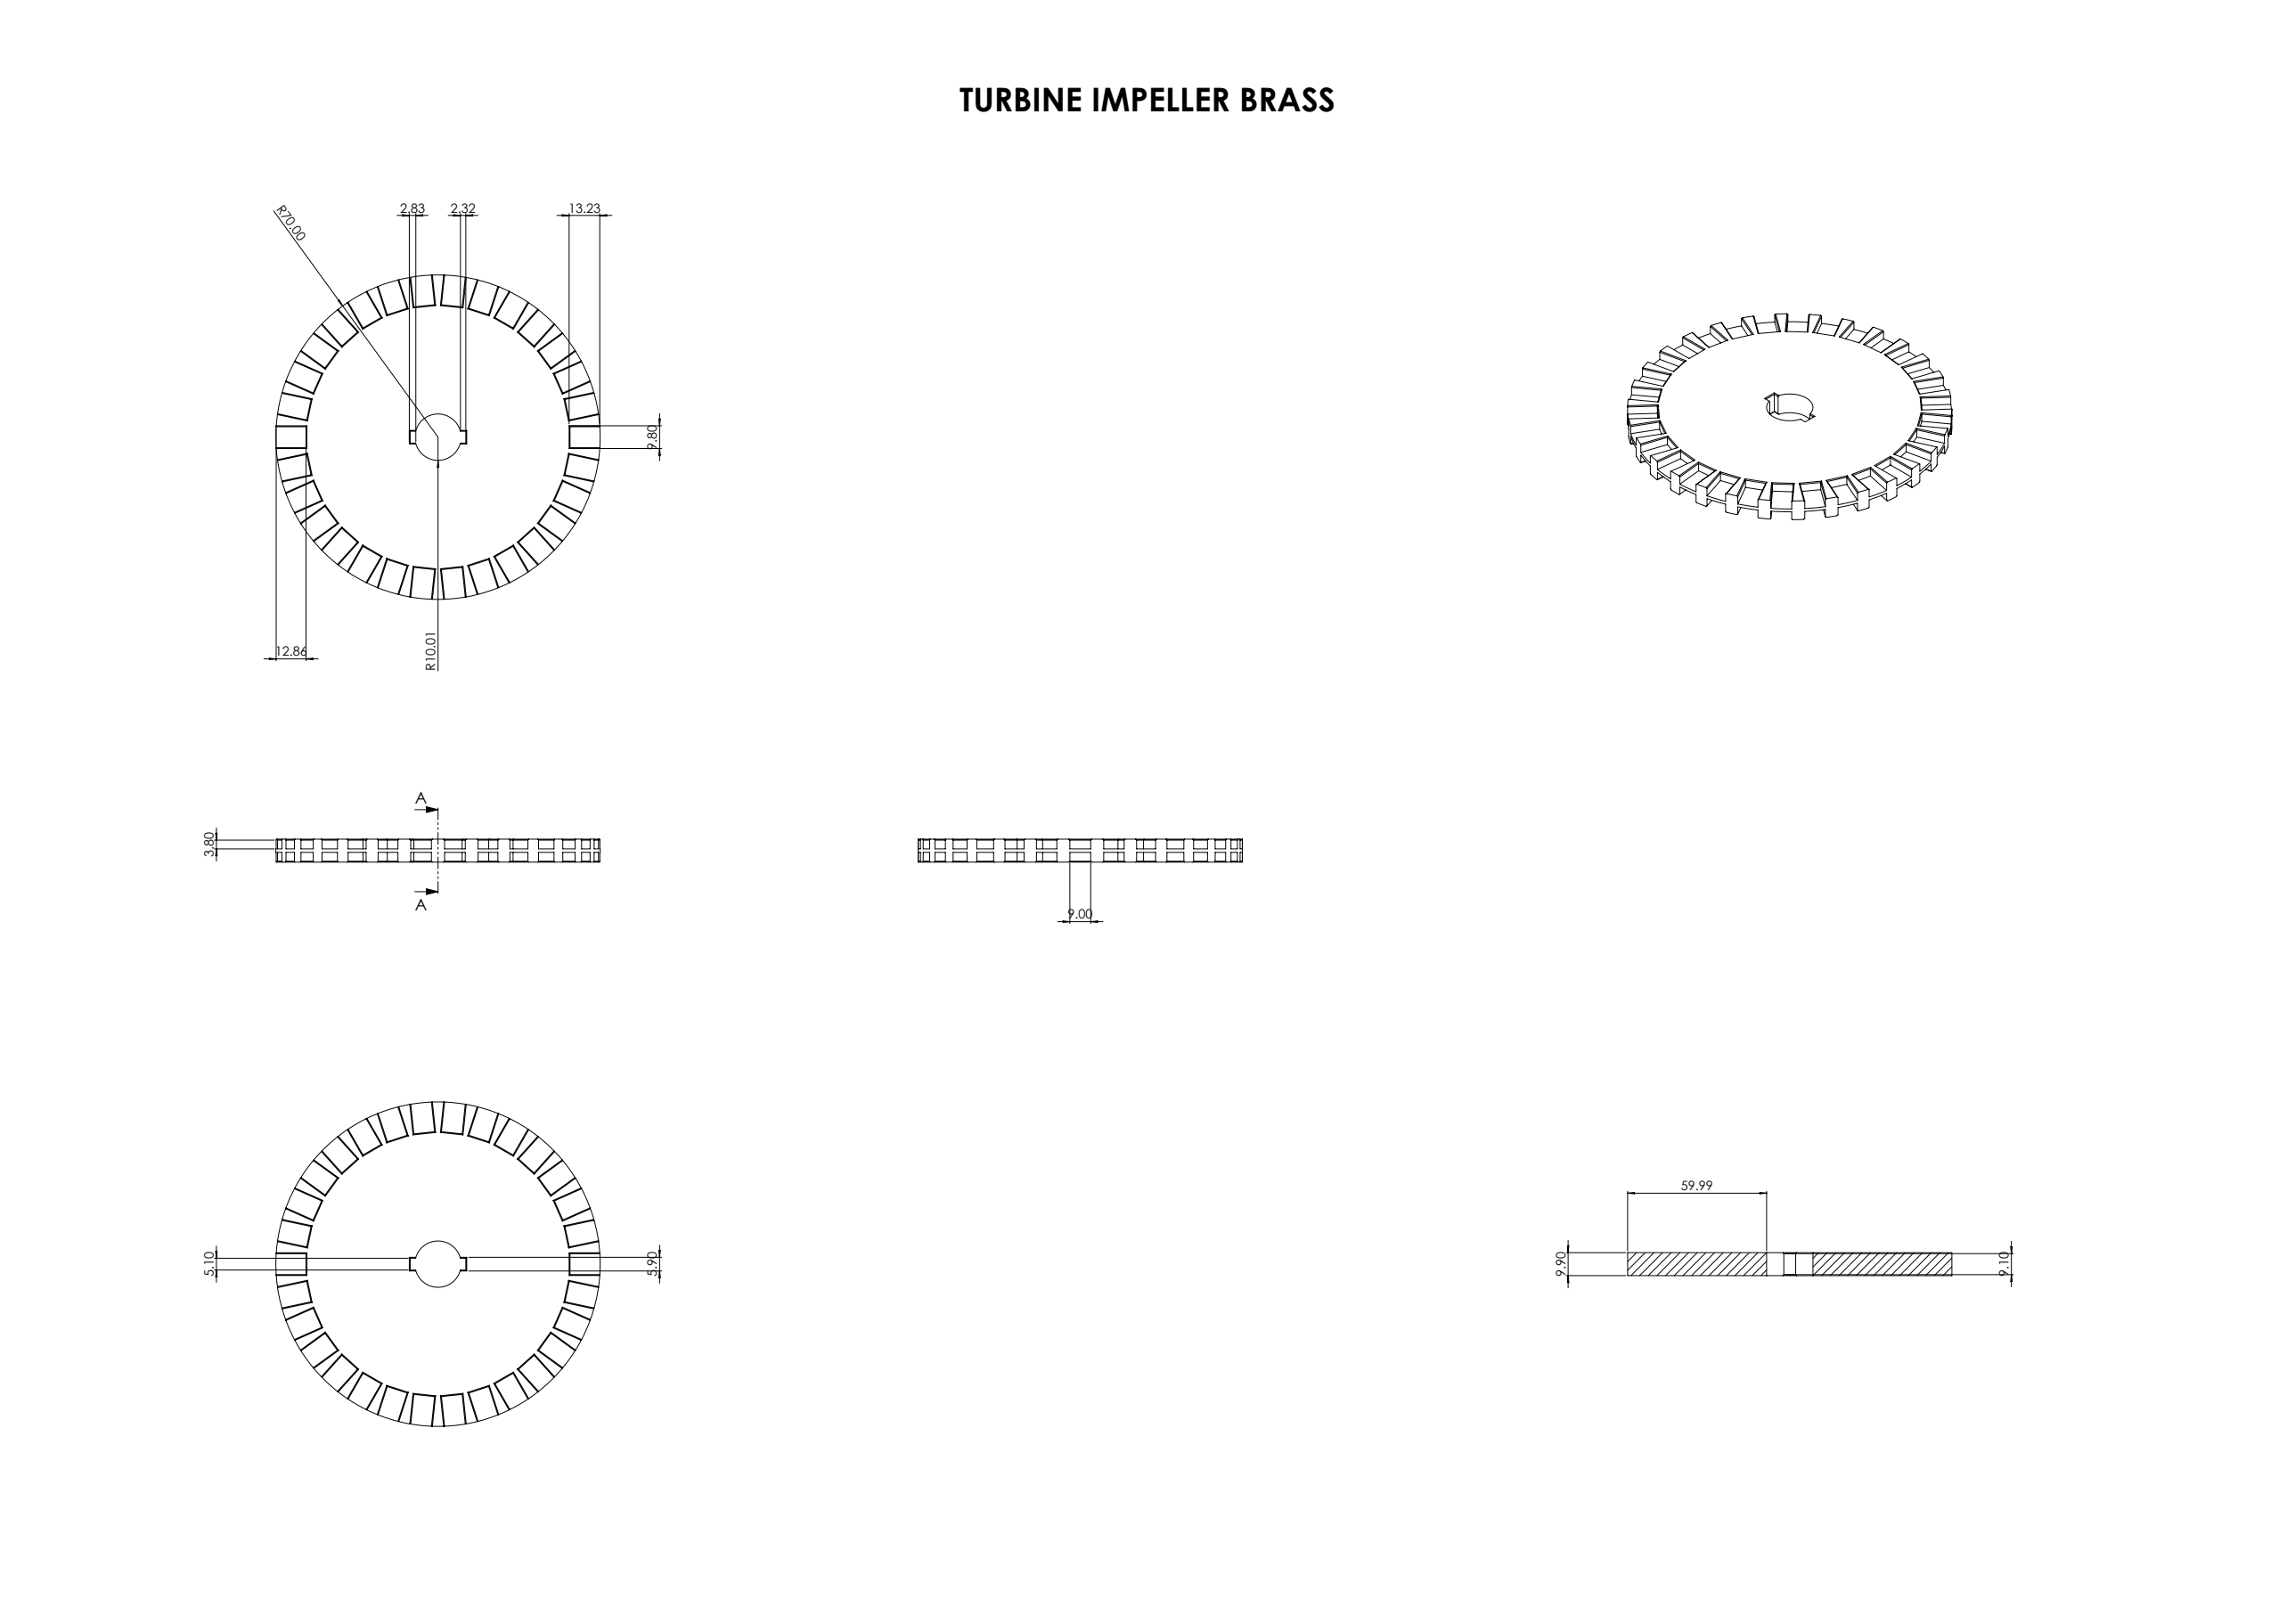
ISO-10303-21;
HEADER;
/* Generated by software containing ST-Developer
 * from STEP Tools, Inc. (www.steptools.com) 
 */

FILE_DESCRIPTION(
/* description */ (''),
/* implementation_level */ '2;1');

FILE_NAME(
/* name */ '04_Turbine_Impeller_Brass.step',
/* time_stamp */ '2026-10-26T04:15:57-07:00',
/* author */ (''),
/* organization */ (''),
/* preprocessor_version */ 'ST-DEVELOPER v20.2',
/* originating_system */ 'Autodesk Translation Framework v15.15.0.0',
/* authorisation */ '');

FILE_SCHEMA (('AUTOMOTIVE_DESIGN { 1 0 10303 214 3 1 1 }'));
ENDSEC;

DATA;
#10=MECHANICAL_DESIGN_GEOMETRIC_PRESENTATION_REPRESENTATION('',(#455),#55737);
#202=ELLIPSE('',#28373,98.9949493661168,70.);
#203=ELLIPSE('',#28377,98.9949493661169,70.);
#204=ELLIPSE('',#28379,98.994949366116,70.);
#205=ELLIPSE('',#28381,98.9949493661166,70.);
#206=ELLIPSE('',#28383,98.9949493661167,70.);
#207=ELLIPSE('',#28386,98.9949493661165,70.);
#208=ELLIPSE('',#28388,98.9949493661168,70.);
#209=ELLIPSE('',#28390,98.9949493661164,70.);
#210=ELLIPSE('',#28392,98.9949493661164,70.);
#211=ELLIPSE('',#28394,98.9949493661161,70.);
#212=ELLIPSE('',#28396,98.9949493661166,70.);
#213=ELLIPSE('',#28398,98.9949493661183,70.);
#214=ELLIPSE('',#28400,98.9949493661177,70.);
#215=ELLIPSE('',#28402,98.9949493661167,70.);
#216=ELLIPSE('',#28404,98.9949493661162,70.);
#217=ELLIPSE('',#28406,98.9949493661183,70.);
#218=ELLIPSE('',#28408,98.9949493661169,70.);
#219=ELLIPSE('',#28410,98.9949493661158,70.);
#220=ELLIPSE('',#28412,98.9949493661173,70.);
#221=ELLIPSE('',#28414,98.9949493661164,70.);
#222=ELLIPSE('',#28416,98.9949493661164,70.);
#223=ELLIPSE('',#28418,98.9949493661165,70.);
#224=ELLIPSE('',#28420,98.9949493661166,70.);
#225=ELLIPSE('',#28422,98.9949493661157,70.);
#226=ELLIPSE('',#28424,98.9949493661165,70.);
#227=ELLIPSE('',#28426,98.9949493661161,70.);
#228=ELLIPSE('',#28428,98.9949493661176,70.);
#229=ELLIPSE('',#28430,98.9949493661175,70.);
#230=ELLIPSE('',#28432,98.9949493661175,70.);
#231=ELLIPSE('',#28434,98.9949493661157,70.);
#232=ELLIPSE('',#28436,98.9949493661157,70.);
#233=ELLIPSE('',#28438,98.9949493661164,70.);
#234=ELLIPSE('',#28440,98.9949493661164,70.);
#235=ELLIPSE('',#28442,98.9949493661168,70.);
#236=ELLIPSE('',#28444,98.9949493661168,70.);
#237=ELLIPSE('',#28446,98.9949493661169,70.);
#238=ELLIPSE('',#28448,98.9949493661168,70.);
#239=ELLIPSE('',#28450,98.9949493661164,70.);
#240=ELLIPSE('',#28452,98.9949493661169,70.);
#241=ELLIPSE('',#28454,98.9949493661162,70.);
#242=ELLIPSE('',#28456,98.9949493661177,70.);
#243=ELLIPSE('',#28458,98.9949493661175,70.);
#244=ELLIPSE('',#28460,98.9949493661171,70.);
#245=ELLIPSE('',#28462,98.9949493661161,70.);
#246=ELLIPSE('',#28464,98.9949493661165,70.);
#247=ELLIPSE('',#28466,98.9949493661153,70.);
#248=ELLIPSE('',#28468,98.9949493661177,70.);
#249=ELLIPSE('',#28470,98.9949493661165,70.);
#250=ELLIPSE('',#28472,98.9949493661174,70.);
#251=ELLIPSE('',#28474,98.9949493661164,70.);
#252=ELLIPSE('',#28476,98.9949493661164,70.);
#253=ELLIPSE('',#28478,98.9949493661163,70.);
#254=ELLIPSE('',#28480,98.9949493661165,70.);
#255=ELLIPSE('',#28482,98.994949366118,70.);
#256=ELLIPSE('',#28484,98.9949493661142,70.);
#257=ELLIPSE('',#28486,98.9949493661172,70.);
#258=ELLIPSE('',#28488,98.9949493661162,70.);
#259=ELLIPSE('',#28490,98.9949493661172,70.);
#260=ELLIPSE('',#28492,98.9949493661145,70.);
#261=ELLIPSE('',#28494,98.9949493661177,70.);
#262=ELLIPSE('',#28496,98.9949493661172,70.);
#263=ELLIPSE('',#28498,98.9949493661164,70.);
#264=ELLIPSE('',#28500,98.9949493661167,70.);
#265=ELLIPSE('',#28502,98.9949493661168,70.);
#266=ELLIPSE('',#28504,98.9949493661167,70.);
#267=ELLIPSE('',#28507,98.9949493661169,70.);
#268=ELLIPSE('',#28509,98.9949493661168,70.);
#269=ELLIPSE('',#28511,98.9949493661169,70.);
#270=ELLIPSE('',#28513,98.9949493661159,70.);
#271=ELLIPSE('',#28515,98.9949493661171,70.);
#272=ELLIPSE('',#28517,98.994949366117,70.);
#273=ELLIPSE('',#28519,98.9949493661175,70.);
#274=ELLIPSE('',#28521,98.9949493661167,70.);
#275=ELLIPSE('',#28523,98.9949493661162,70.);
#276=ELLIPSE('',#28525,98.9949493661158,70.);
#277=ELLIPSE('',#28527,98.9949493661165,70.);
#278=ELLIPSE('',#28529,98.9949493661165,70.);
#279=ELLIPSE('',#28531,98.9949493661172,70.);
#280=ELLIPSE('',#28533,98.9949493661169,70.);
#281=ELLIPSE('',#28535,98.9949493661167,70.);
#282=ELLIPSE('',#28537,98.9949493661167,70.);
#283=ELLIPSE('',#28539,98.9949493661169,70.);
#284=ELLIPSE('',#28541,98.9949493661168,70.);
#285=ELLIPSE('',#28543,98.9949493661168,70.);
#286=ELLIPSE('',#28545,98.9949493661165,70.);
#287=ELLIPSE('',#28547,98.9949493661166,70.);
#288=ELLIPSE('',#28549,98.9949493661168,70.);
#289=ELLIPSE('',#28551,98.9949493661175,70.);
#290=ELLIPSE('',#28553,98.9949493661167,70.);
#291=ELLIPSE('',#28555,98.994949366117,70.);
#292=ELLIPSE('',#28557,98.9949493661167,70.);
#293=ELLIPSE('',#28559,98.9949493661163,70.);
#294=ELLIPSE('',#28561,98.9949493661166,70.);
#295=ELLIPSE('',#28563,98.9949493661168,70.);
#296=ELLIPSE('',#28565,98.9949493661167,70.);
#297=ELLIPSE('',#28567,98.9949493661168,70.);
#298=ELLIPSE('',#28569,98.9949493661169,70.);
#299=ELLIPSE('',#28571,98.9949493661166,70.);
#300=ELLIPSE('',#28573,98.9949493661162,70.);
#301=ELLIPSE('',#28575,98.994949366117,70.);
#302=ELLIPSE('',#28577,98.9949493661165,70.);
#303=ELLIPSE('',#28579,98.9949493661173,70.);
#304=ELLIPSE('',#28581,98.9949493661167,70.);
#305=ELLIPSE('',#28583,98.9949493661156,70.);
#306=ELLIPSE('',#28585,98.9949493661166,70.);
#307=ELLIPSE('',#28587,98.9949493661165,70.);
#308=ELLIPSE('',#28589,98.9949493661157,70.);
#309=ELLIPSE('',#28591,98.9949493661168,70.);
#310=ELLIPSE('',#28593,98.9949493661167,70.);
#311=ELLIPSE('',#28595,98.9949493661167,70.);
#312=ELLIPSE('',#28597,98.9949493661167,70.);
#313=ELLIPSE('',#28599,98.9949493661168,70.);
#314=ELLIPSE('',#28601,98.9949493661165,70.);
#315=ELLIPSE('',#28603,98.9949493661168,70.);
#316=ELLIPSE('',#28605,98.994949366117,70.);
#317=ELLIPSE('',#28607,98.9949493661166,70.);
#318=ELLIPSE('',#28609,98.9949493661156,70.);
#319=ELLIPSE('',#28611,98.9949493661171,70.);
#320=ELLIPSE('',#28613,98.9949493661167,70.);
#321=ELLIPSE('',#28615,98.9949493661169,70.);
#322=ELLIPSE('',#28899,14.1562777593547,10.01);
#323=ELLIPSE('',#28901,14.1562777593547,10.01);
#324=ELLIPSE('',#28906,14.1562777593547,10.01);
#325=ELLIPSE('',#28907,14.1562777593547,10.01);
#326=ELLIPSE('',#28908,14.1562777593547,10.01);
#327=ELLIPSE('',#28912,14.1562777593547,10.01);
#328=ELLIPSE('',#28914,14.1562777593547,10.01);
#329=ELLIPSE('',#28921,14.1562777593547,10.01);
#415=SHAPE_REPRESENTATION_RELATIONSHIP('SRR','None',#55824,#435);
#435=ADVANCED_BREP_SHAPE_REPRESENTATION('',(#475),#55720);
#455=STYLED_ITEM('',(#55984),#475);
#475=MANIFOLD_SOLID_BREP('Body1',#27224);
#681=FACE_BOUND('',#9022,.T.);
#682=FACE_BOUND('',#9161,.T.);
#929=PLANE('',#28372);
#930=PLANE('',#28374);
#931=PLANE('',#28617);
#932=PLANE('',#28618);
#933=PLANE('',#28619);
#934=PLANE('',#28620);
#935=PLANE('',#28621);
#936=PLANE('',#28622);
#937=PLANE('',#28623);
#938=PLANE('',#28624);
#939=PLANE('',#28625);
#940=PLANE('',#28626);
#941=PLANE('',#28627);
#942=PLANE('',#28628);
#943=PLANE('',#28629);
#944=PLANE('',#28630);
#945=PLANE('',#28631);
#946=PLANE('',#28632);
#947=PLANE('',#28633);
#948=PLANE('',#28634);
#949=PLANE('',#28635);
#950=PLANE('',#28636);
#951=PLANE('',#28637);
#952=PLANE('',#28638);
#953=PLANE('',#28639);
#954=PLANE('',#28640);
#955=PLANE('',#28643);
#956=PLANE('',#28644);
#957=PLANE('',#28645);
#958=PLANE('',#28646);
#959=PLANE('',#28647);
#960=PLANE('',#28648);
#961=PLANE('',#28649);
#962=PLANE('',#28650);
#963=PLANE('',#28651);
#964=PLANE('',#28652);
#965=PLANE('',#28653);
#966=PLANE('',#28654);
#967=PLANE('',#28655);
#968=PLANE('',#28656);
#969=PLANE('',#28657);
#970=PLANE('',#28658);
#971=PLANE('',#28659);
#972=PLANE('',#28660);
#973=PLANE('',#28661);
#974=PLANE('',#28662);
#975=PLANE('',#28663);
#976=PLANE('',#28664);
#977=PLANE('',#28665);
#978=PLANE('',#28666);
#979=PLANE('',#28667);
#980=PLANE('',#28668);
#981=PLANE('',#28669);
#982=PLANE('',#28670);
#983=PLANE('',#28671);
#984=PLANE('',#28672);
#985=PLANE('',#28673);
#986=PLANE('',#28674);
#987=PLANE('',#28675);
#988=PLANE('',#28676);
#989=PLANE('',#28677);
#990=PLANE('',#28678);
#991=PLANE('',#28679);
#992=PLANE('',#28680);
#993=PLANE('',#28681);
#994=PLANE('',#28682);
#995=PLANE('',#28683);
#996=PLANE('',#28684);
#997=PLANE('',#28685);
#998=PLANE('',#28686);
#999=PLANE('',#28687);
#1000=PLANE('',#28688);
#1001=PLANE('',#28689);
#1002=PLANE('',#28690);
#1003=PLANE('',#28691);
#1004=PLANE('',#28692);
#1005=PLANE('',#28693);
#1006=PLANE('',#28694);
#1007=PLANE('',#28695);
#1008=PLANE('',#28696);
#1009=PLANE('',#28697);
#1010=PLANE('',#28698);
#1011=PLANE('',#28699);
#1012=PLANE('',#28700);
#1013=PLANE('',#28701);
#1014=PLANE('',#28702);
#1015=PLANE('',#28703);
#1016=PLANE('',#28704);
#1017=PLANE('',#28705);
#1018=PLANE('',#28706);
#1019=PLANE('',#28707);
#1020=PLANE('',#28708);
#1021=PLANE('',#28709);
#1022=PLANE('',#28710);
#1023=PLANE('',#28711);
#1024=PLANE('',#28712);
#1025=PLANE('',#28713);
#1026=PLANE('',#28714);
#1027=PLANE('',#28715);
#1028=PLANE('',#28716);
#1029=PLANE('',#28717);
#1030=PLANE('',#28718);
#1031=PLANE('',#28719);
#1032=PLANE('',#28720);
#1033=PLANE('',#28721);
#1034=PLANE('',#28722);
#1035=PLANE('',#28723);
#1036=PLANE('',#28724);
#1037=PLANE('',#28725);
#1038=PLANE('',#28726);
#1039=PLANE('',#28727);
#1040=PLANE('',#28728);
#1041=PLANE('',#28729);
#1042=PLANE('',#28730);
#1043=PLANE('',#28731);
#1044=PLANE('',#28732);
#1045=PLANE('',#28733);
#1046=PLANE('',#28734);
#1047=PLANE('',#28735);
#1048=PLANE('',#28736);
#1049=PLANE('',#28737);
#1050=PLANE('',#28738);
#1051=PLANE('',#28739);
#1052=PLANE('',#28740);
#1053=PLANE('',#28741);
#1054=PLANE('',#28742);
#1055=PLANE('',#28743);
#1056=PLANE('',#28744);
#1057=PLANE('',#28745);
#1058=PLANE('',#28746);
#1059=PLANE('',#28747);
#1060=PLANE('',#28748);
#1061=PLANE('',#28749);
#1062=PLANE('',#28750);
#1063=PLANE('',#28751);
#1064=PLANE('',#28752);
#1065=PLANE('',#28753);
#1066=PLANE('',#28754);
#1067=PLANE('',#28755);
#1068=PLANE('',#28756);
#1069=PLANE('',#28757);
#1070=PLANE('',#28758);
#1071=PLANE('',#28759);
#1072=PLANE('',#28760);
#1073=PLANE('',#28761);
#1074=PLANE('',#28762);
#1075=PLANE('',#28763);
#1076=PLANE('',#28764);
#1077=PLANE('',#28765);
#1078=PLANE('',#28766);
#1079=PLANE('',#28767);
#1080=PLANE('',#28768);
#1081=PLANE('',#28769);
#1082=PLANE('',#28770);
#1083=PLANE('',#28771);
#1084=PLANE('',#28772);
#1085=PLANE('',#28773);
#1086=PLANE('',#28774);
#1087=PLANE('',#28775);
#1088=PLANE('',#28776);
#1089=PLANE('',#28777);
#1090=PLANE('',#28778);
#1091=PLANE('',#28779);
#1092=PLANE('',#28780);
#1093=PLANE('',#28783);
#1094=PLANE('',#28784);
#1095=PLANE('',#28785);
#1096=PLANE('',#28786);
#1097=PLANE('',#28787);
#1098=PLANE('',#28788);
#1099=PLANE('',#28789);
#1100=PLANE('',#28790);
#1101=PLANE('',#28791);
#1102=PLANE('',#28792);
#1103=PLANE('',#28793);
#1104=PLANE('',#28794);
#1105=PLANE('',#28795);
#1106=PLANE('',#28796);
#1107=PLANE('',#28797);
#1108=PLANE('',#28798);
#1109=PLANE('',#28799);
#1110=PLANE('',#28800);
#1111=PLANE('',#28801);
#1112=PLANE('',#28802);
#1113=PLANE('',#28803);
#1114=PLANE('',#28804);
#1115=PLANE('',#28805);
#1116=PLANE('',#28806);
#1117=PLANE('',#28807);
#1118=PLANE('',#28808);
#1119=PLANE('',#28809);
#1120=PLANE('',#28810);
#1121=PLANE('',#28811);
#1122=PLANE('',#28812);
#1123=PLANE('',#28813);
#1124=PLANE('',#28814);
#1125=PLANE('',#28815);
#1126=PLANE('',#28816);
#1127=PLANE('',#28817);
#1128=PLANE('',#28818);
#1129=PLANE('',#28819);
#1130=PLANE('',#28820);
#1131=PLANE('',#28821);
#1132=PLANE('',#28822);
#1133=PLANE('',#28823);
#1134=PLANE('',#28824);
#1135=PLANE('',#28825);
#1136=PLANE('',#28826);
#1137=PLANE('',#28827);
#1138=PLANE('',#28828);
#1139=PLANE('',#28829);
#1140=PLANE('',#28830);
#1141=PLANE('',#28831);
#1142=PLANE('',#28832);
#1143=PLANE('',#28833);
#1144=PLANE('',#28834);
#1145=PLANE('',#28835);
#1146=PLANE('',#28836);
#1147=PLANE('',#28837);
#1148=PLANE('',#28838);
#1149=PLANE('',#28839);
#1150=PLANE('',#28840);
#1151=PLANE('',#28841);
#1152=PLANE('',#28842);
#1153=PLANE('',#28843);
#1154=PLANE('',#28844);
#1155=PLANE('',#28845);
#1156=PLANE('',#28846);
#1157=PLANE('',#28847);
#1158=PLANE('',#28848);
#1159=PLANE('',#28849);
#1160=PLANE('',#28850);
#1161=PLANE('',#28851);
#1162=PLANE('',#28852);
#1163=PLANE('',#28853);
#1164=PLANE('',#28854);
#1165=PLANE('',#28855);
#1166=PLANE('',#28856);
#1167=PLANE('',#28857);
#1168=PLANE('',#28858);
#1169=PLANE('',#28859);
#1170=PLANE('',#28860);
#1171=PLANE('',#28861);
#1172=PLANE('',#28862);
#1173=PLANE('',#28863);
#1174=PLANE('',#28864);
#1175=PLANE('',#28865);
#1176=PLANE('',#28866);
#1177=PLANE('',#28867);
#1178=PLANE('',#28868);
#1179=PLANE('',#28869);
#1180=PLANE('',#28870);
#1181=PLANE('',#28871);
#1182=PLANE('',#28872);
#1183=PLANE('',#28873);
#1184=PLANE('',#28874);
#1185=PLANE('',#28875);
#1186=PLANE('',#28876);
#1187=PLANE('',#28877);
#1188=PLANE('',#28878);
#1189=PLANE('',#28879);
#1190=PLANE('',#28880);
#1191=PLANE('',#28881);
#1192=PLANE('',#28882);
#1193=PLANE('',#28883);
#1194=PLANE('',#28884);
#1195=PLANE('',#28885);
#1196=PLANE('',#28886);
#1197=PLANE('',#28887);
#1198=PLANE('',#28888);
#1199=PLANE('',#28889);
#1200=PLANE('',#28890);
#1201=PLANE('',#28891);
#1202=PLANE('',#28892);
#1203=PLANE('',#28893);
#1204=PLANE('',#28894);
#1205=PLANE('',#28895);
#1206=PLANE('',#28896);
#1207=PLANE('',#28897);
#1208=PLANE('',#28898);
#1209=PLANE('',#28900);
#1210=PLANE('',#28902);
#1211=PLANE('',#28903);
#1212=PLANE('',#28904);
#1213=PLANE('',#28909);
#1214=PLANE('',#28910);
#1215=PLANE('',#28911);
#1216=PLANE('',#28913);
#1217=PLANE('',#28915);
#1218=PLANE('',#28916);
#1219=PLANE('',#28917);
#1220=PLANE('',#28918);
#1221=PLANE('',#28919);
#1222=PLANE('',#28920);
#1223=PLANE('',#28922);
#1224=PLANE('',#28923);
#1225=PLANE('',#28924);
#1226=PLANE('',#28925);
#1227=PLANE('',#28926);
#1228=PLANE('',#28927);
#1229=PLANE('',#28928);
#1230=PLANE('',#28929);
#1231=PLANE('',#28930);
#1232=PLANE('',#28931);
#1233=PLANE('',#28932);
#1234=PLANE('',#28933);
#1235=PLANE('',#28934);
#1236=PLANE('',#28935);
#1237=PLANE('',#28936);
#1238=PLANE('',#28937);
#1239=PLANE('',#28938);
#1240=PLANE('',#28939);
#1241=PLANE('',#28940);
#1242=PLANE('',#28941);
#1243=PLANE('',#28942);
#1244=PLANE('',#28943);
#1245=PLANE('',#28944);
#1246=PLANE('',#28945);
#1247=PLANE('',#28946);
#1248=PLANE('',#28947);
#1249=PLANE('',#28948);
#1250=PLANE('',#28949);
#1251=PLANE('',#28950);
#1252=PLANE('',#28951);
#1253=PLANE('',#28952);
#1254=PLANE('',#28953);
#1255=PLANE('',#28954);
#1256=PLANE('',#28955);
#1257=PLANE('',#28956);
#1258=PLANE('',#28957);
#1259=PLANE('',#28958);
#1260=PLANE('',#28959);
#1261=PLANE('',#28960);
#1262=PLANE('',#28961);
#1263=PLANE('',#28962);
#1264=PLANE('',#28963);
#1265=PLANE('',#28964);
#1266=PLANE('',#28965);
#1267=PLANE('',#28966);
#1268=PLANE('',#28967);
#1269=PLANE('',#28968);
#1270=PLANE('',#28969);
#1271=PLANE('',#28970);
#1272=PLANE('',#28971);
#1273=PLANE('',#28972);
#1274=PLANE('',#28973);
#1275=PLANE('',#28974);
#1276=PLANE('',#28975);
#1277=PLANE('',#28976);
#1278=PLANE('',#28977);
#1279=PLANE('',#28978);
#1280=PLANE('',#28979);
#1281=PLANE('',#28980);
#1282=PLANE('',#28981);
#1283=PLANE('',#28982);
#1284=PLANE('',#28983);
#1285=PLANE('',#28984);
#1286=PLANE('',#28985);
#1287=PLANE('',#28986);
#1288=PLANE('',#28987);
#1289=PLANE('',#28988);
#1290=PLANE('',#28989);
#1291=PLANE('',#28990);
#1292=PLANE('',#28991);
#1293=PLANE('',#28992);
#1294=PLANE('',#28993);
#1295=PLANE('',#28994);
#1296=PLANE('',#28995);
#1297=PLANE('',#28996);
#1298=PLANE('',#28997);
#1299=PLANE('',#28998);
#1300=PLANE('',#28999);
#1301=PLANE('',#29000);
#1302=PLANE('',#29001);
#1303=PLANE('',#29002);
#1304=PLANE('',#29003);
#1305=PLANE('',#29004);
#1306=PLANE('',#29005);
#1307=PLANE('',#29006);
#1308=PLANE('',#29007);
#1309=PLANE('',#29008);
#1310=PLANE('',#29009);
#1311=PLANE('',#29010);
#1312=PLANE('',#29011);
#1313=PLANE('',#29012);
#1314=PLANE('',#29013);
#1315=PLANE('',#29014);
#1316=PLANE('',#29015);
#1317=PLANE('',#29016);
#1318=PLANE('',#29017);
#1319=PLANE('',#29018);
#1320=PLANE('',#29019);
#1321=PLANE('',#29020);
#1322=PLANE('',#29021);
#1323=PLANE('',#29022);
#1324=PLANE('',#29023);
#1325=PLANE('',#29024);
#1326=PLANE('',#29025);
#1327=PLANE('',#29026);
#1328=PLANE('',#29027);
#1329=PLANE('',#29028);
#1330=PLANE('',#29029);
#1331=PLANE('',#29030);
#1332=PLANE('',#29031);
#1333=PLANE('',#29032);
#1334=PLANE('',#29033);
#1335=PLANE('',#29034);
#1336=PLANE('',#29035);
#1337=PLANE('',#29036);
#1338=PLANE('',#29037);
#1339=PLANE('',#29038);
#1340=PLANE('',#29039);
#1341=PLANE('',#29040);
#1342=PLANE('',#29041);
#1343=PLANE('',#29042);
#1344=PLANE('',#29043);
#1345=PLANE('',#29044);
#1346=PLANE('',#29045);
#1347=PLANE('',#29046);
#1348=PLANE('',#29047);
#1349=PLANE('',#29048);
#1350=PLANE('',#29049);
#1351=PLANE('',#29050);
#1352=PLANE('',#29051);
#1353=PLANE('',#29052);
#1354=PLANE('',#29053);
#1355=PLANE('',#29054);
#1356=PLANE('',#29055);
#1357=PLANE('',#29056);
#1358=PLANE('',#29057);
#1359=PLANE('',#29058);
#1360=PLANE('',#29059);
#1361=PLANE('',#29060);
#1362=PLANE('',#29061);
#1363=PLANE('',#29062);
#1364=PLANE('',#29063);
#1365=PLANE('',#29064);
#1366=PLANE('',#29065);
#1367=PLANE('',#29066);
#1368=PLANE('',#29067);
#2353=LINE('',#42571,#4724);
#2354=LINE('',#42573,#4725);
#2355=LINE('',#42574,#4726);
#2356=LINE('',#42577,#4727);
#2357=LINE('',#42579,#4728);
#2358=LINE('',#42580,#4729);
#2359=LINE('',#42587,#4730);
#2360=LINE('',#42591,#4731);
#2361=LINE('',#42599,#4732);
#2362=LINE('',#42603,#4733);
#2363=LINE('',#42609,#4734);
#2364=LINE('',#42615,#4735);
#2365=LINE('',#42619,#4736);
#2366=LINE('',#42627,#4737);
#2367=LINE('',#42631,#4738);
#2368=LINE('',#42639,#4739);
#2369=LINE('',#42643,#4740);
#2370=LINE('',#42651,#4741);
#2371=LINE('',#42655,#4742);
#2372=LINE('',#42663,#4743);
#2373=LINE('',#42667,#4744);
#2374=LINE('',#42675,#4745);
#2375=LINE('',#42679,#4746);
#2376=LINE('',#42687,#4747);
#2377=LINE('',#42691,#4748);
#2378=LINE('',#42699,#4749);
#2379=LINE('',#42703,#4750);
#2380=LINE('',#42711,#4751);
#2381=LINE('',#42715,#4752);
#2382=LINE('',#42723,#4753);
#2383=LINE('',#42727,#4754);
#2384=LINE('',#42735,#4755);
#2385=LINE('',#42739,#4756);
#2386=LINE('',#42747,#4757);
#2387=LINE('',#42751,#4758);
#2388=LINE('',#42759,#4759);
#2389=LINE('',#42763,#4760);
#2390=LINE('',#42771,#4761);
#2391=LINE('',#42775,#4762);
#2392=LINE('',#42783,#4763);
#2393=LINE('',#42787,#4764);
#2394=LINE('',#42795,#4765);
#2395=LINE('',#42799,#4766);
#2396=LINE('',#42807,#4767);
#2397=LINE('',#42811,#4768);
#2398=LINE('',#42819,#4769);
#2399=LINE('',#42823,#4770);
#2400=LINE('',#42831,#4771);
#2401=LINE('',#42835,#4772);
#2402=LINE('',#42843,#4773);
#2403=LINE('',#42847,#4774);
#2404=LINE('',#42855,#4775);
#2405=LINE('',#42859,#4776);
#2406=LINE('',#42867,#4777);
#2407=LINE('',#42871,#4778);
#2408=LINE('',#42879,#4779);
#2409=LINE('',#42883,#4780);
#2410=LINE('',#42891,#4781);
#2411=LINE('',#42895,#4782);
#2412=LINE('',#42903,#4783);
#2413=LINE('',#42907,#4784);
#2414=LINE('',#42915,#4785);
#2415=LINE('',#42919,#4786);
#2416=LINE('',#42927,#4787);
#2417=LINE('',#42931,#4788);
#2418=LINE('',#42939,#4789);
#2419=LINE('',#42943,#4790);
#2420=LINE('',#42951,#4791);
#2421=LINE('',#42955,#4792);
#2422=LINE('',#42963,#4793);
#2423=LINE('',#42967,#4794);
#2424=LINE('',#42976,#4795);
#2425=LINE('',#42980,#4796);
#2426=LINE('',#42988,#4797);
#2427=LINE('',#42992,#4798);
#2428=LINE('',#43000,#4799);
#2429=LINE('',#43004,#4800);
#2430=LINE('',#43012,#4801);
#2431=LINE('',#43016,#4802);
#2432=LINE('',#43024,#4803);
#2433=LINE('',#43028,#4804);
#2434=LINE('',#43036,#4805);
#2435=LINE('',#43040,#4806);
#2436=LINE('',#43048,#4807);
#2437=LINE('',#43052,#4808);
#2438=LINE('',#43060,#4809);
#2439=LINE('',#43064,#4810);
#2440=LINE('',#43072,#4811);
#2441=LINE('',#43076,#4812);
#2442=LINE('',#43084,#4813);
#2443=LINE('',#43088,#4814);
#2444=LINE('',#43096,#4815);
#2445=LINE('',#43100,#4816);
#2446=LINE('',#43108,#4817);
#2447=LINE('',#43112,#4818);
#2448=LINE('',#43120,#4819);
#2449=LINE('',#43124,#4820);
#2450=LINE('',#43132,#4821);
#2451=LINE('',#43136,#4822);
#2452=LINE('',#43144,#4823);
#2453=LINE('',#43148,#4824);
#2454=LINE('',#43156,#4825);
#2455=LINE('',#43160,#4826);
#2456=LINE('',#43168,#4827);
#2457=LINE('',#43172,#4828);
#2458=LINE('',#43180,#4829);
#2459=LINE('',#43184,#4830);
#2460=LINE('',#43192,#4831);
#2461=LINE('',#43196,#4832);
#2462=LINE('',#43204,#4833);
#2463=LINE('',#43208,#4834);
#2464=LINE('',#43216,#4835);
#2465=LINE('',#43220,#4836);
#2466=LINE('',#43228,#4837);
#2467=LINE('',#43232,#4838);
#2468=LINE('',#43240,#4839);
#2469=LINE('',#43244,#4840);
#2470=LINE('',#43252,#4841);
#2471=LINE('',#43256,#4842);
#2472=LINE('',#43264,#4843);
#2473=LINE('',#43268,#4844);
#2474=LINE('',#43276,#4845);
#2475=LINE('',#43280,#4846);
#2476=LINE('',#43288,#4847);
#2477=LINE('',#43292,#4848);
#2478=LINE('',#43300,#4849);
#2479=LINE('',#43304,#4850);
#2480=LINE('',#43306,#4851);
#2481=LINE('',#43307,#4852);
#2482=LINE('',#43310,#4853);
#2483=LINE('',#43312,#4854);
#2484=LINE('',#43313,#4855);
#2485=LINE('',#43315,#4856);
#2486=LINE('',#43316,#4857);
#2487=LINE('',#43319,#4858);
#2488=LINE('',#43320,#4859);
#2489=LINE('',#43323,#4860);
#2490=LINE('',#43324,#4861);
#2491=LINE('',#43326,#4862);
#2492=LINE('',#43329,#4863);
#2493=LINE('',#43331,#4864);
#2494=LINE('',#43332,#4865);
#2495=LINE('',#43335,#4866);
#2496=LINE('',#43337,#4867);
#2497=LINE('',#43338,#4868);
#2498=LINE('',#43340,#4869);
#2499=LINE('',#43341,#4870);
#2500=LINE('',#43344,#4871);
#2501=LINE('',#43345,#4872);
#2502=LINE('',#43348,#4873);
#2503=LINE('',#43349,#4874);
#2504=LINE('',#43351,#4875);
#2505=LINE('',#43354,#4876);
#2506=LINE('',#43356,#4877);
#2507=LINE('',#43357,#4878);
#2508=LINE('',#43360,#4879);
#2509=LINE('',#43362,#4880);
#2510=LINE('',#43363,#4881);
#2511=LINE('',#43365,#4882);
#2512=LINE('',#43366,#4883);
#2513=LINE('',#43369,#4884);
#2514=LINE('',#43370,#4885);
#2515=LINE('',#43373,#4886);
#2516=LINE('',#43374,#4887);
#2517=LINE('',#43376,#4888);
#2518=LINE('',#43379,#4889);
#2519=LINE('',#43381,#4890);
#2520=LINE('',#43382,#4891);
#2521=LINE('',#43385,#4892);
#2522=LINE('',#43387,#4893);
#2523=LINE('',#43388,#4894);
#2524=LINE('',#43391,#4895);
#2525=LINE('',#43392,#4896);
#2526=LINE('',#43395,#4897);
#2527=LINE('',#43396,#4898);
#2528=LINE('',#43398,#4899);
#2529=LINE('',#43399,#4900);
#2530=LINE('',#43402,#4901);
#2531=LINE('',#43403,#4902);
#2532=LINE('',#43405,#4903);
#2533=LINE('',#43407,#4904);
#2534=LINE('',#43408,#4905);
#2535=LINE('',#43410,#4906);
#2536=LINE('',#43412,#4907);
#2537=LINE('',#43413,#4908);
#2538=LINE('',#43415,#4909);
#2539=LINE('',#43417,#4910);
#2540=LINE('',#43418,#4911);
#2541=LINE('',#43420,#4912);
#2542=LINE('',#43422,#4913);
#2543=LINE('',#43423,#4914);
#2544=LINE('',#43425,#4915);
#2545=LINE('',#43427,#4916);
#2546=LINE('',#43428,#4917);
#2547=LINE('',#43430,#4918);
#2548=LINE('',#43432,#4919);
#2549=LINE('',#43433,#4920);
#2550=LINE('',#43435,#4921);
#2551=LINE('',#43437,#4922);
#2552=LINE('',#43438,#4923);
#2553=LINE('',#43440,#4924);
#2554=LINE('',#43442,#4925);
#2555=LINE('',#43443,#4926);
#2556=LINE('',#43445,#4927);
#2557=LINE('',#43447,#4928);
#2558=LINE('',#43448,#4929);
#2559=LINE('',#43450,#4930);
#2560=LINE('',#43452,#4931);
#2561=LINE('',#43453,#4932);
#2562=LINE('',#43455,#4933);
#2563=LINE('',#43457,#4934);
#2564=LINE('',#43458,#4935);
#2565=LINE('',#43460,#4936);
#2566=LINE('',#43462,#4937);
#2567=LINE('',#43463,#4938);
#2568=LINE('',#43465,#4939);
#2569=LINE('',#43467,#4940);
#2570=LINE('',#43468,#4941);
#2571=LINE('',#43470,#4942);
#2572=LINE('',#43472,#4943);
#2573=LINE('',#43473,#4944);
#2574=LINE('',#43475,#4945);
#2575=LINE('',#43477,#4946);
#2576=LINE('',#43478,#4947);
#2577=LINE('',#43480,#4948);
#2578=LINE('',#43482,#4949);
#2579=LINE('',#43483,#4950);
#2580=LINE('',#43485,#4951);
#2581=LINE('',#43487,#4952);
#2582=LINE('',#43488,#4953);
#2583=LINE('',#43490,#4954);
#2584=LINE('',#43492,#4955);
#2585=LINE('',#43493,#4956);
#2586=LINE('',#43495,#4957);
#2587=LINE('',#43497,#4958);
#2588=LINE('',#43498,#4959);
#2589=LINE('',#43500,#4960);
#2590=LINE('',#43502,#4961);
#2591=LINE('',#43503,#4962);
#2592=LINE('',#43505,#4963);
#2593=LINE('',#43507,#4964);
#2594=LINE('',#43508,#4965);
#2595=LINE('',#43510,#4966);
#2596=LINE('',#43512,#4967);
#2597=LINE('',#43513,#4968);
#2598=LINE('',#43515,#4969);
#2599=LINE('',#43517,#4970);
#2600=LINE('',#43518,#4971);
#2601=LINE('',#43520,#4972);
#2602=LINE('',#43522,#4973);
#2603=LINE('',#43523,#4974);
#2604=LINE('',#43525,#4975);
#2605=LINE('',#43527,#4976);
#2606=LINE('',#43528,#4977);
#2607=LINE('',#43531,#4978);
#2608=LINE('',#43535,#4979);
#2609=LINE('',#43537,#4980);
#2610=LINE('',#43539,#4981);
#2611=LINE('',#43543,#4982);
#2612=LINE('',#43544,#4983);
#2613=LINE('',#43547,#4984);
#2614=LINE('',#43548,#4985);
#2615=LINE('',#43551,#4986);
#2616=LINE('',#43552,#4987);
#2617=LINE('',#43554,#4988);
#2618=LINE('',#43557,#4989);
#2619=LINE('',#43558,#4990);
#2620=LINE('',#43561,#4991);
#2621=LINE('',#43562,#4992);
#2622=LINE('',#43564,#4993);
#2623=LINE('',#43567,#4994);
#2624=LINE('',#43568,#4995);
#2625=LINE('',#43571,#4996);
#2626=LINE('',#43572,#4997);
#2627=LINE('',#43574,#4998);
#2628=LINE('',#43577,#4999);
#2629=LINE('',#43578,#5000);
#2630=LINE('',#43581,#5001);
#2631=LINE('',#43582,#5002);
#2632=LINE('',#43584,#5003);
#2633=LINE('',#43587,#5004);
#2634=LINE('',#43588,#5005);
#2635=LINE('',#43591,#5006);
#2636=LINE('',#43592,#5007);
#2637=LINE('',#43594,#5008);
#2638=LINE('',#43597,#5009);
#2639=LINE('',#43598,#5010);
#2640=LINE('',#43601,#5011);
#2641=LINE('',#43602,#5012);
#2642=LINE('',#43604,#5013);
#2643=LINE('',#43607,#5014);
#2644=LINE('',#43608,#5015);
#2645=LINE('',#43611,#5016);
#2646=LINE('',#43612,#5017);
#2647=LINE('',#43614,#5018);
#2648=LINE('',#43617,#5019);
#2649=LINE('',#43618,#5020);
#2650=LINE('',#43621,#5021);
#2651=LINE('',#43622,#5022);
#2652=LINE('',#43624,#5023);
#2653=LINE('',#43627,#5024);
#2654=LINE('',#43628,#5025);
#2655=LINE('',#43631,#5026);
#2656=LINE('',#43632,#5027);
#2657=LINE('',#43634,#5028);
#2658=LINE('',#43637,#5029);
#2659=LINE('',#43638,#5030);
#2660=LINE('',#43641,#5031);
#2661=LINE('',#43642,#5032);
#2662=LINE('',#43644,#5033);
#2663=LINE('',#43647,#5034);
#2664=LINE('',#43648,#5035);
#2665=LINE('',#43651,#5036);
#2666=LINE('',#43652,#5037);
#2667=LINE('',#43654,#5038);
#2668=LINE('',#43657,#5039);
#2669=LINE('',#43658,#5040);
#2670=LINE('',#43661,#5041);
#2671=LINE('',#43662,#5042);
#2672=LINE('',#43664,#5043);
#2673=LINE('',#43667,#5044);
#2674=LINE('',#43668,#5045);
#2675=LINE('',#43671,#5046);
#2676=LINE('',#43672,#5047);
#2677=LINE('',#43674,#5048);
#2678=LINE('',#43677,#5049);
#2679=LINE('',#43678,#5050);
#2680=LINE('',#43681,#5051);
#2681=LINE('',#43682,#5052);
#2682=LINE('',#43684,#5053);
#2683=LINE('',#43687,#5054);
#2684=LINE('',#43688,#5055);
#2685=LINE('',#43691,#5056);
#2686=LINE('',#43692,#5057);
#2687=LINE('',#43694,#5058);
#2688=LINE('',#43697,#5059);
#2689=LINE('',#43698,#5060);
#2690=LINE('',#43701,#5061);
#2691=LINE('',#43702,#5062);
#2692=LINE('',#43704,#5063);
#2693=LINE('',#43707,#5064);
#2694=LINE('',#43708,#5065);
#2695=LINE('',#43711,#5066);
#2696=LINE('',#43712,#5067);
#2697=LINE('',#43714,#5068);
#2698=LINE('',#43717,#5069);
#2699=LINE('',#43718,#5070);
#2700=LINE('',#43721,#5071);
#2701=LINE('',#43722,#5072);
#2702=LINE('',#43724,#5073);
#2703=LINE('',#43727,#5074);
#2704=LINE('',#43728,#5075);
#2705=LINE('',#43731,#5076);
#2706=LINE('',#43732,#5077);
#2707=LINE('',#43734,#5078);
#2708=LINE('',#43737,#5079);
#2709=LINE('',#43738,#5080);
#2710=LINE('',#43741,#5081);
#2711=LINE('',#43742,#5082);
#2712=LINE('',#43745,#5083);
#2713=LINE('',#43746,#5084);
#2714=LINE('',#43748,#5085);
#2715=LINE('',#43751,#5086);
#2716=LINE('',#43752,#5087);
#2717=LINE('',#43754,#5088);
#2718=LINE('',#43757,#5089);
#2719=LINE('',#43758,#5090);
#2720=LINE('',#43761,#5091);
#2721=LINE('',#43762,#5092);
#2722=LINE('',#43764,#5093);
#2723=LINE('',#43767,#5094);
#2724=LINE('',#43768,#5095);
#2725=LINE('',#43771,#5096);
#2726=LINE('',#43772,#5097);
#2727=LINE('',#43774,#5098);
#2728=LINE('',#43777,#5099);
#2729=LINE('',#43778,#5100);
#2730=LINE('',#43781,#5101);
#2731=LINE('',#43782,#5102);
#2732=LINE('',#43784,#5103);
#2733=LINE('',#43787,#5104);
#2734=LINE('',#43788,#5105);
#2735=LINE('',#43791,#5106);
#2736=LINE('',#43792,#5107);
#2737=LINE('',#43794,#5108);
#2738=LINE('',#43797,#5109);
#2739=LINE('',#43798,#5110);
#2740=LINE('',#43801,#5111);
#2741=LINE('',#43802,#5112);
#2742=LINE('',#43804,#5113);
#2743=LINE('',#43807,#5114);
#2744=LINE('',#43808,#5115);
#2745=LINE('',#43811,#5116);
#2746=LINE('',#43812,#5117);
#2747=LINE('',#43814,#5118);
#2748=LINE('',#43817,#5119);
#2749=LINE('',#43818,#5120);
#2750=LINE('',#43821,#5121);
#2751=LINE('',#43822,#5122);
#2752=LINE('',#43824,#5123);
#2753=LINE('',#43827,#5124);
#2754=LINE('',#43828,#5125);
#2755=LINE('',#43831,#5126);
#2756=LINE('',#43832,#5127);
#2757=LINE('',#43834,#5128);
#2758=LINE('',#43837,#5129);
#2759=LINE('',#43838,#5130);
#2760=LINE('',#43841,#5131);
#2761=LINE('',#43842,#5132);
#2762=LINE('',#43844,#5133);
#2763=LINE('',#43847,#5134);
#2764=LINE('',#43848,#5135);
#2765=LINE('',#43851,#5136);
#2766=LINE('',#43852,#5137);
#2767=LINE('',#43854,#5138);
#2768=LINE('',#43857,#5139);
#2769=LINE('',#43858,#5140);
#2770=LINE('',#43861,#5141);
#2771=LINE('',#43862,#5142);
#2772=LINE('',#43864,#5143);
#2773=LINE('',#43867,#5144);
#2774=LINE('',#43868,#5145);
#2775=LINE('',#43871,#5146);
#2776=LINE('',#43872,#5147);
#2777=LINE('',#43874,#5148);
#2778=LINE('',#43877,#5149);
#2779=LINE('',#43878,#5150);
#2780=LINE('',#43881,#5151);
#2781=LINE('',#43882,#5152);
#2782=LINE('',#43884,#5153);
#2783=LINE('',#43887,#5154);
#2784=LINE('',#43888,#5155);
#2785=LINE('',#43891,#5156);
#2786=LINE('',#43892,#5157);
#2787=LINE('',#43894,#5158);
#2788=LINE('',#43897,#5159);
#2789=LINE('',#43898,#5160);
#2790=LINE('',#43901,#5161);
#2791=LINE('',#43902,#5162);
#2792=LINE('',#43904,#5163);
#2793=LINE('',#43907,#5164);
#2794=LINE('',#43908,#5165);
#2795=LINE('',#43911,#5166);
#2796=LINE('',#43912,#5167);
#2797=LINE('',#43914,#5168);
#2798=LINE('',#43917,#5169);
#2799=LINE('',#43918,#5170);
#2800=LINE('',#43921,#5171);
#2801=LINE('',#43922,#5172);
#2802=LINE('',#43924,#5173);
#2803=LINE('',#43927,#5174);
#2804=LINE('',#43928,#5175);
#2805=LINE('',#43931,#5176);
#2806=LINE('',#43932,#5177);
#2807=LINE('',#43934,#5178);
#2808=LINE('',#43937,#5179);
#2809=LINE('',#43938,#5180);
#2810=LINE('',#43941,#5181);
#2811=LINE('',#43942,#5182);
#2812=LINE('',#43944,#5183);
#2813=LINE('',#43947,#5184);
#2814=LINE('',#43948,#5185);
#2815=LINE('',#43951,#5186);
#2816=LINE('',#43952,#5187);
#2817=LINE('',#43954,#5188);
#2818=LINE('',#43957,#5189);
#2819=LINE('',#43958,#5190);
#2820=LINE('',#43961,#5191);
#2821=LINE('',#43962,#5192);
#2822=LINE('',#43964,#5193);
#2823=LINE('',#43967,#5194);
#2824=LINE('',#43968,#5195);
#2825=LINE('',#43971,#5196);
#2826=LINE('',#43972,#5197);
#2827=LINE('',#43974,#5198);
#2828=LINE('',#43977,#5199);
#2829=LINE('',#43978,#5200);
#2830=LINE('',#43981,#5201);
#2831=LINE('',#43982,#5202);
#2832=LINE('',#43984,#5203);
#2833=LINE('',#43987,#5204);
#2834=LINE('',#43988,#5205);
#2835=LINE('',#43991,#5206);
#2836=LINE('',#43992,#5207);
#2837=LINE('',#43994,#5208);
#2838=LINE('',#43998,#5209);
#2839=LINE('',#44000,#5210);
#2840=LINE('',#44002,#5211);
#2841=LINE('',#44003,#5212);
#2842=LINE('',#44005,#5213);
#2843=LINE('',#44006,#5214);
#2844=LINE('',#44008,#5215);
#2845=LINE('',#44010,#5216);
#2846=LINE('',#44012,#5217);
#2847=LINE('',#44013,#5218);
#2848=LINE('',#44015,#5219);
#2849=LINE('',#44017,#5220);
#2850=LINE('',#44018,#5221);
#2851=LINE('',#44020,#5222);
#2852=LINE('',#44022,#5223);
#2853=LINE('',#44023,#5224);
#2854=LINE('',#44025,#5225);
#2855=LINE('',#44027,#5226);
#2856=LINE('',#44028,#5227);
#2857=LINE('',#44030,#5228);
#2858=LINE('',#44032,#5229);
#2859=LINE('',#44033,#5230);
#2860=LINE('',#44035,#5231);
#2861=LINE('',#44037,#5232);
#2862=LINE('',#44038,#5233);
#2863=LINE('',#44040,#5234);
#2864=LINE('',#44042,#5235);
#2865=LINE('',#44043,#5236);
#2866=LINE('',#44045,#5237);
#2867=LINE('',#44047,#5238);
#2868=LINE('',#44048,#5239);
#2869=LINE('',#44050,#5240);
#2870=LINE('',#44052,#5241);
#2871=LINE('',#44053,#5242);
#2872=LINE('',#44055,#5243);
#2873=LINE('',#44057,#5244);
#2874=LINE('',#44058,#5245);
#2875=LINE('',#44060,#5246);
#2876=LINE('',#44062,#5247);
#2877=LINE('',#44063,#5248);
#2878=LINE('',#44065,#5249);
#2879=LINE('',#44067,#5250);
#2880=LINE('',#44068,#5251);
#2881=LINE('',#44070,#5252);
#2882=LINE('',#44072,#5253);
#2883=LINE('',#44073,#5254);
#2884=LINE('',#44075,#5255);
#2885=LINE('',#44077,#5256);
#2886=LINE('',#44078,#5257);
#2887=LINE('',#44080,#5258);
#2888=LINE('',#44082,#5259);
#2889=LINE('',#44083,#5260);
#2890=LINE('',#44085,#5261);
#2891=LINE('',#44087,#5262);
#2892=LINE('',#44088,#5263);
#2893=LINE('',#44090,#5264);
#2894=LINE('',#44092,#5265);
#2895=LINE('',#44093,#5266);
#2896=LINE('',#44095,#5267);
#2897=LINE('',#44097,#5268);
#2898=LINE('',#44098,#5269);
#2899=LINE('',#44100,#5270);
#2900=LINE('',#44102,#5271);
#2901=LINE('',#44103,#5272);
#2902=LINE('',#44105,#5273);
#2903=LINE('',#44107,#5274);
#2904=LINE('',#44108,#5275);
#2905=LINE('',#44110,#5276);
#2906=LINE('',#44112,#5277);
#2907=LINE('',#44113,#5278);
#2908=LINE('',#44115,#5279);
#2909=LINE('',#44117,#5280);
#2910=LINE('',#44118,#5281);
#2911=LINE('',#44120,#5282);
#2912=LINE('',#44122,#5283);
#2913=LINE('',#44123,#5284);
#2914=LINE('',#44125,#5285);
#2915=LINE('',#44127,#5286);
#2916=LINE('',#44128,#5287);
#2917=LINE('',#44130,#5288);
#2918=LINE('',#44132,#5289);
#2919=LINE('',#44133,#5290);
#2920=LINE('',#44135,#5291);
#2921=LINE('',#44137,#5292);
#2922=LINE('',#44138,#5293);
#2923=LINE('',#44140,#5294);
#2924=LINE('',#44142,#5295);
#2925=LINE('',#44143,#5296);
#2926=LINE('',#44145,#5297);
#2927=LINE('',#44147,#5298);
#2928=LINE('',#44148,#5299);
#2929=LINE('',#44150,#5300);
#2930=LINE('',#44152,#5301);
#2931=LINE('',#44153,#5302);
#2932=LINE('',#44156,#5303);
#2933=LINE('',#44158,#5304);
#2934=LINE('',#44160,#5305);
#2935=LINE('',#44164,#5306);
#2936=LINE('',#44166,#5307);
#2937=LINE('',#44168,#5308);
#2938=LINE('',#44171,#5309);
#2939=LINE('',#44174,#5310);
#2940=LINE('',#44176,#5311);
#2941=LINE('',#44177,#5312);
#2942=LINE('',#44179,#5313);
#2943=LINE('',#44181,#5314);
#2944=LINE('',#44184,#5315);
#2945=LINE('',#44186,#5316);
#2946=LINE('',#44187,#5317);
#2947=LINE('',#44189,#5318);
#2948=LINE('',#44191,#5319);
#2949=LINE('',#44194,#5320);
#2950=LINE('',#44195,#5321);
#2951=LINE('',#44198,#5322);
#2952=LINE('',#44199,#5323);
#2953=LINE('',#44202,#5324);
#2954=LINE('',#44204,#5325);
#2955=LINE('',#44205,#5326);
#2956=LINE('',#44207,#5327);
#2957=LINE('',#44209,#5328);
#2958=LINE('',#44212,#5329);
#2959=LINE('',#44214,#5330);
#2960=LINE('',#44215,#5331);
#2961=LINE('',#44217,#5332);
#2962=LINE('',#44219,#5333);
#2963=LINE('',#44222,#5334);
#2964=LINE('',#44223,#5335);
#2965=LINE('',#44226,#5336);
#2966=LINE('',#44227,#5337);
#2967=LINE('',#44230,#5338);
#2968=LINE('',#44232,#5339);
#2969=LINE('',#44233,#5340);
#2970=LINE('',#44235,#5341);
#2971=LINE('',#44237,#5342);
#2972=LINE('',#44240,#5343);
#2973=LINE('',#44242,#5344);
#2974=LINE('',#44243,#5345);
#2975=LINE('',#44245,#5346);
#2976=LINE('',#44247,#5347);
#2977=LINE('',#44250,#5348);
#2978=LINE('',#44251,#5349);
#2979=LINE('',#44254,#5350);
#2980=LINE('',#44255,#5351);
#2981=LINE('',#44258,#5352);
#2982=LINE('',#44259,#5353);
#2983=LINE('',#44262,#5354);
#2984=LINE('',#44263,#5355);
#2985=LINE('',#44265,#5356);
#2986=LINE('',#44268,#5357);
#2987=LINE('',#44270,#5358);
#2988=LINE('',#44271,#5359);
#2989=LINE('',#44273,#5360);
#2990=LINE('',#44275,#5361);
#2991=LINE('',#44278,#5362);
#2992=LINE('',#44280,#5363);
#2993=LINE('',#44281,#5364);
#2994=LINE('',#44283,#5365);
#2995=LINE('',#44285,#5366);
#2996=LINE('',#44288,#5367);
#2997=LINE('',#44289,#5368);
#2998=LINE('',#44292,#5369);
#2999=LINE('',#44293,#5370);
#3000=LINE('',#44296,#5371);
#3001=LINE('',#44298,#5372);
#3002=LINE('',#44299,#5373);
#3003=LINE('',#44301,#5374);
#3004=LINE('',#44303,#5375);
#3005=LINE('',#44306,#5376);
#3006=LINE('',#44308,#5377);
#3007=LINE('',#44309,#5378);
#3008=LINE('',#44311,#5379);
#3009=LINE('',#44313,#5380);
#3010=LINE('',#44316,#5381);
#3011=LINE('',#44317,#5382);
#3012=LINE('',#44320,#5383);
#3013=LINE('',#44321,#5384);
#3014=LINE('',#44324,#5385);
#3015=LINE('',#44326,#5386);
#3016=LINE('',#44327,#5387);
#3017=LINE('',#44329,#5388);
#3018=LINE('',#44331,#5389);
#3019=LINE('',#44334,#5390);
#3020=LINE('',#44336,#5391);
#3021=LINE('',#44337,#5392);
#3022=LINE('',#44339,#5393);
#3023=LINE('',#44341,#5394);
#3024=LINE('',#44344,#5395);
#3025=LINE('',#44345,#5396);
#3026=LINE('',#44348,#5397);
#3027=LINE('',#44349,#5398);
#3028=LINE('',#44352,#5399);
#3029=LINE('',#44354,#5400);
#3030=LINE('',#44355,#5401);
#3031=LINE('',#44357,#5402);
#3032=LINE('',#44359,#5403);
#3033=LINE('',#44362,#5404);
#3034=LINE('',#44364,#5405);
#3035=LINE('',#44365,#5406);
#3036=LINE('',#44367,#5407);
#3037=LINE('',#44369,#5408);
#3038=LINE('',#44372,#5409);
#3039=LINE('',#44373,#5410);
#3040=LINE('',#44376,#5411);
#3041=LINE('',#44377,#5412);
#3042=LINE('',#44380,#5413);
#3043=LINE('',#44382,#5414);
#3044=LINE('',#44383,#5415);
#3045=LINE('',#44385,#5416);
#3046=LINE('',#44387,#5417);
#3047=LINE('',#44390,#5418);
#3048=LINE('',#44392,#5419);
#3049=LINE('',#44393,#5420);
#3050=LINE('',#44395,#5421);
#3051=LINE('',#44397,#5422);
#3052=LINE('',#44400,#5423);
#3053=LINE('',#44401,#5424);
#3054=LINE('',#44404,#5425);
#3055=LINE('',#44405,#5426);
#3056=LINE('',#44408,#5427);
#3057=LINE('',#44410,#5428);
#3058=LINE('',#44411,#5429);
#3059=LINE('',#44413,#5430);
#3060=LINE('',#44415,#5431);
#3061=LINE('',#44418,#5432);
#3062=LINE('',#44420,#5433);
#3063=LINE('',#44421,#5434);
#3064=LINE('',#44423,#5435);
#3065=LINE('',#44425,#5436);
#3066=LINE('',#44428,#5437);
#3067=LINE('',#44429,#5438);
#3068=LINE('',#44432,#5439);
#3069=LINE('',#44433,#5440);
#3070=LINE('',#44436,#5441);
#3071=LINE('',#44438,#5442);
#3072=LINE('',#44439,#5443);
#3073=LINE('',#44441,#5444);
#3074=LINE('',#44443,#5445);
#3075=LINE('',#44446,#5446);
#3076=LINE('',#44448,#5447);
#3077=LINE('',#44449,#5448);
#3078=LINE('',#44451,#5449);
#3079=LINE('',#44453,#5450);
#3080=LINE('',#44456,#5451);
#3081=LINE('',#44458,#5452);
#3082=LINE('',#44459,#5453);
#3083=LINE('',#44461,#5454);
#3084=LINE('',#44463,#5455);
#3085=LINE('',#44466,#5456);
#3086=LINE('',#44467,#5457);
#3087=LINE('',#44470,#5458);
#3088=LINE('',#44471,#5459);
#3089=LINE('',#44474,#5460);
#3090=LINE('',#44476,#5461);
#3091=LINE('',#44477,#5462);
#3092=LINE('',#44479,#5463);
#3093=LINE('',#44481,#5464);
#3094=LINE('',#44484,#5465);
#3095=LINE('',#44486,#5466);
#3096=LINE('',#44487,#5467);
#3097=LINE('',#44489,#5468);
#3098=LINE('',#44491,#5469);
#3099=LINE('',#44494,#5470);
#3100=LINE('',#44495,#5471);
#3101=LINE('',#44498,#5472);
#3102=LINE('',#44499,#5473);
#3103=LINE('',#44502,#5474);
#3104=LINE('',#44504,#5475);
#3105=LINE('',#44505,#5476);
#3106=LINE('',#44507,#5477);
#3107=LINE('',#44509,#5478);
#3108=LINE('',#44512,#5479);
#3109=LINE('',#44514,#5480);
#3110=LINE('',#44515,#5481);
#3111=LINE('',#44517,#5482);
#3112=LINE('',#44519,#5483);
#3113=LINE('',#44522,#5484);
#3114=LINE('',#44523,#5485);
#3115=LINE('',#44526,#5486);
#3116=LINE('',#44527,#5487);
#3117=LINE('',#44530,#5488);
#3118=LINE('',#44531,#5489);
#3119=LINE('',#44534,#5490);
#3120=LINE('',#44535,#5491);
#3121=LINE('',#44537,#5492);
#3122=LINE('',#44540,#5493);
#3123=LINE('',#44542,#5494);
#3124=LINE('',#44543,#5495);
#3125=LINE('',#44545,#5496);
#3126=LINE('',#44547,#5497);
#3127=LINE('',#44550,#5498);
#3128=LINE('',#44552,#5499);
#3129=LINE('',#44553,#5500);
#3130=LINE('',#44555,#5501);
#3131=LINE('',#44557,#5502);
#3132=LINE('',#44560,#5503);
#3133=LINE('',#44561,#5504);
#3134=LINE('',#44564,#5505);
#3135=LINE('',#44565,#5506);
#3136=LINE('',#44568,#5507);
#3137=LINE('',#44570,#5508);
#3138=LINE('',#44571,#5509);
#3139=LINE('',#44575,#5510);
#3140=LINE('',#44578,#5511);
#3141=LINE('',#44582,#5512);
#3142=LINE('',#44584,#5513);
#3143=LINE('',#44585,#5514);
#3144=LINE('',#44588,#5515);
#3145=LINE('',#44589,#5516);
#3146=LINE('',#44592,#5517);
#3147=LINE('',#44593,#5518);
#3148=LINE('',#44598,#5519);
#3149=LINE('',#44602,#5520);
#3150=LINE('',#44603,#5521);
#3151=LINE('',#44610,#5522);
#3152=LINE('',#44612,#5523);
#3153=LINE('',#44615,#5524);
#3154=LINE('',#44616,#5525);
#3155=LINE('',#44618,#5526);
#3156=LINE('',#44621,#5527);
#3157=LINE('',#44623,#5528);
#3158=LINE('',#44624,#5529);
#3159=LINE('',#44627,#5530);
#3160=LINE('',#44628,#5531);
#3161=LINE('',#44630,#5532);
#3162=LINE('',#44633,#5533);
#3163=LINE('',#44635,#5534);
#3164=LINE('',#44639,#5535);
#3165=LINE('',#44644,#5536);
#3166=LINE('',#44646,#5537);
#3167=LINE('',#44647,#5538);
#3168=LINE('',#44649,#5539);
#3169=LINE('',#44651,#5540);
#3170=LINE('',#44656,#5541);
#3171=LINE('',#44658,#5542);
#3172=LINE('',#44659,#5543);
#3173=LINE('',#44661,#5544);
#3174=LINE('',#44663,#5545);
#3175=LINE('',#44667,#5546);
#3176=LINE('',#44672,#5547);
#3177=LINE('',#44674,#5548);
#3178=LINE('',#44675,#5549);
#3179=LINE('',#44677,#5550);
#3180=LINE('',#44679,#5551);
#3181=LINE('',#44683,#5552);
#3182=LINE('',#44688,#5553);
#3183=LINE('',#44690,#5554);
#3184=LINE('',#44691,#5555);
#3185=LINE('',#44693,#5556);
#3186=LINE('',#44695,#5557);
#3187=LINE('',#44699,#5558);
#3188=LINE('',#44704,#5559);
#3189=LINE('',#44706,#5560);
#3190=LINE('',#44707,#5561);
#3191=LINE('',#44709,#5562);
#3192=LINE('',#44711,#5563);
#3193=LINE('',#44716,#5564);
#3194=LINE('',#44718,#5565);
#3195=LINE('',#44719,#5566);
#3196=LINE('',#44721,#5567);
#3197=LINE('',#44723,#5568);
#3198=LINE('',#44727,#5569);
#3199=LINE('',#44732,#5570);
#3200=LINE('',#44734,#5571);
#3201=LINE('',#44735,#5572);
#3202=LINE('',#44737,#5573);
#3203=LINE('',#44739,#5574);
#3204=LINE('',#44743,#5575);
#3205=LINE('',#44748,#5576);
#3206=LINE('',#44750,#5577);
#3207=LINE('',#44751,#5578);
#3208=LINE('',#44753,#5579);
#3209=LINE('',#44755,#5580);
#3210=LINE('',#44759,#5581);
#3211=LINE('',#44764,#5582);
#3212=LINE('',#44766,#5583);
#3213=LINE('',#44767,#5584);
#3214=LINE('',#44769,#5585);
#3215=LINE('',#44771,#5586);
#3216=LINE('',#44775,#5587);
#3217=LINE('',#44780,#5588);
#3218=LINE('',#44782,#5589);
#3219=LINE('',#44783,#5590);
#3220=LINE('',#44785,#5591);
#3221=LINE('',#44787,#5592);
#3222=LINE('',#44791,#5593);
#3223=LINE('',#44794,#5594);
#3224=LINE('',#44798,#5595);
#3225=LINE('',#44800,#5596);
#3226=LINE('',#44801,#5597);
#3227=LINE('',#44803,#5598);
#3228=LINE('',#44805,#5599);
#3229=LINE('',#44809,#5600);
#3230=LINE('',#44814,#5601);
#3231=LINE('',#44816,#5602);
#3232=LINE('',#44817,#5603);
#3233=LINE('',#44819,#5604);
#3234=LINE('',#44821,#5605);
#3235=LINE('',#44826,#5606);
#3236=LINE('',#44828,#5607);
#3237=LINE('',#44829,#5608);
#3238=LINE('',#44831,#5609);
#3239=LINE('',#44833,#5610);
#3240=LINE('',#44836,#5611);
#3241=LINE('',#44839,#5612);
#3242=LINE('',#44843,#5613);
#3243=LINE('',#44844,#5614);
#3244=LINE('',#44847,#5615);
#3245=LINE('',#44848,#5616);
#3246=LINE('',#44850,#5617);
#3247=LINE('',#44854,#5618);
#3248=LINE('',#44856,#5619);
#3249=LINE('',#44857,#5620);
#3250=LINE('',#44859,#5621);
#3251=LINE('',#44861,#5622);
#3252=LINE('',#44865,#5623);
#3253=LINE('',#44866,#5624);
#3254=LINE('',#44869,#5625);
#3255=LINE('',#44870,#5626);
#3256=LINE('',#44872,#5627);
#3257=LINE('',#44875,#5628);
#3258=LINE('',#44879,#5629);
#3259=LINE('',#44880,#5630);
#3260=LINE('',#44883,#5631);
#3261=LINE('',#44884,#5632);
#3262=LINE('',#44886,#5633);
#3263=LINE('',#44890,#5634);
#3264=LINE('',#44892,#5635);
#3265=LINE('',#44893,#5636);
#3266=LINE('',#44895,#5637);
#3267=LINE('',#44897,#5638);
#3268=LINE('',#44901,#5639);
#3269=LINE('',#44902,#5640);
#3270=LINE('',#44905,#5641);
#3271=LINE('',#44906,#5642);
#3272=LINE('',#44908,#5643);
#3273=LINE('',#44911,#5644);
#3274=LINE('',#44915,#5645);
#3275=LINE('',#44916,#5646);
#3276=LINE('',#44919,#5647);
#3277=LINE('',#44920,#5648);
#3278=LINE('',#44922,#5649);
#3279=LINE('',#44926,#5650);
#3280=LINE('',#44928,#5651);
#3281=LINE('',#44929,#5652);
#3282=LINE('',#44931,#5653);
#3283=LINE('',#44933,#5654);
#3284=LINE('',#44937,#5655);
#3285=LINE('',#44938,#5656);
#3286=LINE('',#44941,#5657);
#3287=LINE('',#44942,#5658);
#3288=LINE('',#44944,#5659);
#3289=LINE('',#44948,#5660);
#3290=LINE('',#44950,#5661);
#3291=LINE('',#44951,#5662);
#3292=LINE('',#44953,#5663);
#3293=LINE('',#44955,#5664);
#4724=VECTOR('',#32395,10.);
#4725=VECTOR('',#32396,10.);
#4726=VECTOR('',#32397,10.);
#4727=VECTOR('',#32400,10.);
#4728=VECTOR('',#32401,10.);
#4729=VECTOR('',#32402,10.);
#4730=VECTOR('',#32409,10.);
#4731=VECTOR('',#32412,10.);
#4732=VECTOR('',#32419,10.);
#4733=VECTOR('',#32422,10.);
#4734=VECTOR('',#32427,70.);
#4735=VECTOR('',#32432,10.);
#4736=VECTOR('',#32435,10.);
#4737=VECTOR('',#32442,10.);
#4738=VECTOR('',#32445,10.);
#4739=VECTOR('',#32452,10.);
#4740=VECTOR('',#32455,10.);
#4741=VECTOR('',#32462,10.);
#4742=VECTOR('',#32465,10.);
#4743=VECTOR('',#32472,10.);
#4744=VECTOR('',#32475,10.);
#4745=VECTOR('',#32482,10.);
#4746=VECTOR('',#32485,10.);
#4747=VECTOR('',#32492,10.);
#4748=VECTOR('',#32495,10.);
#4749=VECTOR('',#32502,10.);
#4750=VECTOR('',#32505,10.);
#4751=VECTOR('',#32512,10.);
#4752=VECTOR('',#32515,10.);
#4753=VECTOR('',#32522,10.);
#4754=VECTOR('',#32525,10.);
#4755=VECTOR('',#32532,10.);
#4756=VECTOR('',#32535,10.);
#4757=VECTOR('',#32542,10.);
#4758=VECTOR('',#32545,10.);
#4759=VECTOR('',#32552,10.);
#4760=VECTOR('',#32555,10.);
#4761=VECTOR('',#32562,10.);
#4762=VECTOR('',#32565,10.);
#4763=VECTOR('',#32572,10.);
#4764=VECTOR('',#32575,10.);
#4765=VECTOR('',#32582,10.);
#4766=VECTOR('',#32585,10.);
#4767=VECTOR('',#32592,10.);
#4768=VECTOR('',#32595,10.);
#4769=VECTOR('',#32602,10.);
#4770=VECTOR('',#32605,10.);
#4771=VECTOR('',#32612,10.);
#4772=VECTOR('',#32615,10.);
#4773=VECTOR('',#32622,10.);
#4774=VECTOR('',#32625,10.);
#4775=VECTOR('',#32632,10.);
#4776=VECTOR('',#32635,10.);
#4777=VECTOR('',#32642,10.);
#4778=VECTOR('',#32645,10.);
#4779=VECTOR('',#32652,10.);
#4780=VECTOR('',#32655,10.);
#4781=VECTOR('',#32662,10.);
#4782=VECTOR('',#32665,10.);
#4783=VECTOR('',#32672,10.);
#4784=VECTOR('',#32675,10.);
#4785=VECTOR('',#32682,10.);
#4786=VECTOR('',#32685,10.);
#4787=VECTOR('',#32692,10.);
#4788=VECTOR('',#32695,10.);
#4789=VECTOR('',#32702,10.);
#4790=VECTOR('',#32705,10.);
#4791=VECTOR('',#32712,10.);
#4792=VECTOR('',#32715,10.);
#4793=VECTOR('',#32722,10.);
#4794=VECTOR('',#32725,10.);
#4795=VECTOR('',#32734,10.);
#4796=VECTOR('',#32737,10.);
#4797=VECTOR('',#32744,10.);
#4798=VECTOR('',#32747,10.);
#4799=VECTOR('',#32754,10.);
#4800=VECTOR('',#32757,10.);
#4801=VECTOR('',#32764,10.);
#4802=VECTOR('',#32767,10.);
#4803=VECTOR('',#32774,10.);
#4804=VECTOR('',#32777,10.);
#4805=VECTOR('',#32784,10.);
#4806=VECTOR('',#32787,10.);
#4807=VECTOR('',#32794,10.);
#4808=VECTOR('',#32797,10.);
#4809=VECTOR('',#32804,10.);
#4810=VECTOR('',#32807,10.);
#4811=VECTOR('',#32814,10.);
#4812=VECTOR('',#32817,10.);
#4813=VECTOR('',#32824,10.);
#4814=VECTOR('',#32827,10.);
#4815=VECTOR('',#32834,10.);
#4816=VECTOR('',#32837,10.);
#4817=VECTOR('',#32844,10.);
#4818=VECTOR('',#32847,10.);
#4819=VECTOR('',#32854,10.);
#4820=VECTOR('',#32857,10.);
#4821=VECTOR('',#32864,10.);
#4822=VECTOR('',#32867,10.);
#4823=VECTOR('',#32874,10.);
#4824=VECTOR('',#32877,10.);
#4825=VECTOR('',#32884,10.);
#4826=VECTOR('',#32887,10.);
#4827=VECTOR('',#32894,10.);
#4828=VECTOR('',#32897,10.);
#4829=VECTOR('',#32904,10.);
#4830=VECTOR('',#32907,10.);
#4831=VECTOR('',#32914,10.);
#4832=VECTOR('',#32917,10.);
#4833=VECTOR('',#32924,10.);
#4834=VECTOR('',#32927,10.);
#4835=VECTOR('',#32934,10.);
#4836=VECTOR('',#32937,10.);
#4837=VECTOR('',#32944,10.);
#4838=VECTOR('',#32947,10.);
#4839=VECTOR('',#32954,10.);
#4840=VECTOR('',#32957,10.);
#4841=VECTOR('',#32964,10.);
#4842=VECTOR('',#32967,10.);
#4843=VECTOR('',#32974,10.);
#4844=VECTOR('',#32977,10.);
#4845=VECTOR('',#32984,10.);
#4846=VECTOR('',#32987,10.);
#4847=VECTOR('',#32994,10.);
#4848=VECTOR('',#32997,10.);
#4849=VECTOR('',#33004,10.);
#4850=VECTOR('',#33009,10.);
#4851=VECTOR('',#33010,10.);
#4852=VECTOR('',#33011,10.);
#4853=VECTOR('',#33014,10.);
#4854=VECTOR('',#33015,10.);
#4855=VECTOR('',#33016,10.);
#4856=VECTOR('',#33019,10.);
#4857=VECTOR('',#33020,10.);
#4858=VECTOR('',#33023,10.);
#4859=VECTOR('',#33024,10.);
#4860=VECTOR('',#33027,10.);
#4861=VECTOR('',#33028,10.);
#4862=VECTOR('',#33031,10.);
#4863=VECTOR('',#33034,10.);
#4864=VECTOR('',#33035,10.);
#4865=VECTOR('',#33036,10.);
#4866=VECTOR('',#33039,10.);
#4867=VECTOR('',#33040,10.);
#4868=VECTOR('',#33041,10.);
#4869=VECTOR('',#33044,10.);
#4870=VECTOR('',#33045,10.);
#4871=VECTOR('',#33048,10.);
#4872=VECTOR('',#33049,10.);
#4873=VECTOR('',#33052,10.);
#4874=VECTOR('',#33053,10.);
#4875=VECTOR('',#33056,10.);
#4876=VECTOR('',#33059,10.);
#4877=VECTOR('',#33060,10.);
#4878=VECTOR('',#33061,10.);
#4879=VECTOR('',#33064,10.);
#4880=VECTOR('',#33065,10.);
#4881=VECTOR('',#33066,10.);
#4882=VECTOR('',#33069,10.);
#4883=VECTOR('',#33070,10.);
#4884=VECTOR('',#33073,10.);
#4885=VECTOR('',#33074,10.);
#4886=VECTOR('',#33077,10.);
#4887=VECTOR('',#33078,10.);
#4888=VECTOR('',#33081,10.);
#4889=VECTOR('',#33084,10.);
#4890=VECTOR('',#33085,10.);
#4891=VECTOR('',#33086,10.);
#4892=VECTOR('',#33089,10.);
#4893=VECTOR('',#33090,10.);
#4894=VECTOR('',#33091,10.);
#4895=VECTOR('',#33094,10.);
#4896=VECTOR('',#33095,10.);
#4897=VECTOR('',#33098,10.);
#4898=VECTOR('',#33099,10.);
#4899=VECTOR('',#33102,10.);
#4900=VECTOR('',#33103,10.);
#4901=VECTOR('',#33106,10.);
#4902=VECTOR('',#33107,10.);
#4903=VECTOR('',#33108,10.);
#4904=VECTOR('',#33109,10.);
#4905=VECTOR('',#33110,10.);
#4906=VECTOR('',#33111,10.);
#4907=VECTOR('',#33112,10.);
#4908=VECTOR('',#33113,10.);
#4909=VECTOR('',#33114,10.);
#4910=VECTOR('',#33115,10.);
#4911=VECTOR('',#33116,10.);
#4912=VECTOR('',#33117,10.);
#4913=VECTOR('',#33118,10.);
#4914=VECTOR('',#33119,10.);
#4915=VECTOR('',#33120,10.);
#4916=VECTOR('',#33121,10.);
#4917=VECTOR('',#33122,10.);
#4918=VECTOR('',#33123,10.);
#4919=VECTOR('',#33124,10.);
#4920=VECTOR('',#33125,10.);
#4921=VECTOR('',#33126,10.);
#4922=VECTOR('',#33127,10.);
#4923=VECTOR('',#33128,10.);
#4924=VECTOR('',#33129,10.);
#4925=VECTOR('',#33130,10.);
#4926=VECTOR('',#33131,10.);
#4927=VECTOR('',#33132,10.);
#4928=VECTOR('',#33133,10.);
#4929=VECTOR('',#33134,10.);
#4930=VECTOR('',#33135,10.);
#4931=VECTOR('',#33136,10.);
#4932=VECTOR('',#33137,10.);
#4933=VECTOR('',#33138,10.);
#4934=VECTOR('',#33139,10.);
#4935=VECTOR('',#33140,10.);
#4936=VECTOR('',#33141,10.);
#4937=VECTOR('',#33142,10.);
#4938=VECTOR('',#33143,10.);
#4939=VECTOR('',#33144,10.);
#4940=VECTOR('',#33145,10.);
#4941=VECTOR('',#33146,10.);
#4942=VECTOR('',#33147,10.);
#4943=VECTOR('',#33148,10.);
#4944=VECTOR('',#33149,10.);
#4945=VECTOR('',#33150,10.);
#4946=VECTOR('',#33151,10.);
#4947=VECTOR('',#33152,10.);
#4948=VECTOR('',#33153,10.);
#4949=VECTOR('',#33154,10.);
#4950=VECTOR('',#33155,10.);
#4951=VECTOR('',#33156,10.);
#4952=VECTOR('',#33157,10.);
#4953=VECTOR('',#33158,10.);
#4954=VECTOR('',#33159,10.);
#4955=VECTOR('',#33160,10.);
#4956=VECTOR('',#33161,10.);
#4957=VECTOR('',#33162,10.);
#4958=VECTOR('',#33163,10.);
#4959=VECTOR('',#33164,10.);
#4960=VECTOR('',#33165,10.);
#4961=VECTOR('',#33166,10.);
#4962=VECTOR('',#33167,10.);
#4963=VECTOR('',#33168,10.);
#4964=VECTOR('',#33169,10.);
#4965=VECTOR('',#33170,10.);
#4966=VECTOR('',#33171,10.);
#4967=VECTOR('',#33172,10.);
#4968=VECTOR('',#33173,10.);
#4969=VECTOR('',#33174,10.);
#4970=VECTOR('',#33175,10.);
#4971=VECTOR('',#33176,10.);
#4972=VECTOR('',#33177,10.);
#4973=VECTOR('',#33178,10.);
#4974=VECTOR('',#33179,10.);
#4975=VECTOR('',#33180,10.);
#4976=VECTOR('',#33181,10.);
#4977=VECTOR('',#33182,10.);
#4978=VECTOR('',#33183,10.);
#4979=VECTOR('',#33186,10.);
#4980=VECTOR('',#33187,10.);
#4981=VECTOR('',#33188,10.);
#4982=VECTOR('',#33191,10.);
#4983=VECTOR('',#33192,10.);
#4984=VECTOR('',#33195,10.);
#4985=VECTOR('',#33196,10.);
#4986=VECTOR('',#33199,10.);
#4987=VECTOR('',#33200,10.);
#4988=VECTOR('',#33203,10.);
#4989=VECTOR('',#33206,10.);
#4990=VECTOR('',#33207,10.);
#4991=VECTOR('',#33210,10.);
#4992=VECTOR('',#33211,10.);
#4993=VECTOR('',#33214,10.);
#4994=VECTOR('',#33217,10.);
#4995=VECTOR('',#33218,10.);
#4996=VECTOR('',#33221,10.);
#4997=VECTOR('',#33222,10.);
#4998=VECTOR('',#33225,10.);
#4999=VECTOR('',#33228,10.);
#5000=VECTOR('',#33229,10.);
#5001=VECTOR('',#33232,10.);
#5002=VECTOR('',#33233,10.);
#5003=VECTOR('',#33236,10.);
#5004=VECTOR('',#33239,10.);
#5005=VECTOR('',#33240,10.);
#5006=VECTOR('',#33243,10.);
#5007=VECTOR('',#33244,10.);
#5008=VECTOR('',#33247,10.);
#5009=VECTOR('',#33250,10.);
#5010=VECTOR('',#33251,10.);
#5011=VECTOR('',#33254,10.);
#5012=VECTOR('',#33255,10.);
#5013=VECTOR('',#33258,10.);
#5014=VECTOR('',#33261,10.);
#5015=VECTOR('',#33262,10.);
#5016=VECTOR('',#33265,10.);
#5017=VECTOR('',#33266,10.);
#5018=VECTOR('',#33269,10.);
#5019=VECTOR('',#33272,10.);
#5020=VECTOR('',#33273,10.);
#5021=VECTOR('',#33276,10.);
#5022=VECTOR('',#33277,10.);
#5023=VECTOR('',#33280,10.);
#5024=VECTOR('',#33283,10.);
#5025=VECTOR('',#33284,10.);
#5026=VECTOR('',#33287,10.);
#5027=VECTOR('',#33288,10.);
#5028=VECTOR('',#33291,10.);
#5029=VECTOR('',#33294,10.);
#5030=VECTOR('',#33295,10.);
#5031=VECTOR('',#33298,10.);
#5032=VECTOR('',#33299,10.);
#5033=VECTOR('',#33302,10.);
#5034=VECTOR('',#33305,10.);
#5035=VECTOR('',#33306,10.);
#5036=VECTOR('',#33309,10.);
#5037=VECTOR('',#33310,10.);
#5038=VECTOR('',#33313,10.);
#5039=VECTOR('',#33316,10.);
#5040=VECTOR('',#33317,10.);
#5041=VECTOR('',#33320,10.);
#5042=VECTOR('',#33321,10.);
#5043=VECTOR('',#33324,10.);
#5044=VECTOR('',#33327,10.);
#5045=VECTOR('',#33328,10.);
#5046=VECTOR('',#33331,10.);
#5047=VECTOR('',#33332,10.);
#5048=VECTOR('',#33335,10.);
#5049=VECTOR('',#33338,10.);
#5050=VECTOR('',#33339,10.);
#5051=VECTOR('',#33342,10.);
#5052=VECTOR('',#33343,10.);
#5053=VECTOR('',#33346,10.);
#5054=VECTOR('',#33349,10.);
#5055=VECTOR('',#33350,10.);
#5056=VECTOR('',#33353,10.);
#5057=VECTOR('',#33354,10.);
#5058=VECTOR('',#33357,10.);
#5059=VECTOR('',#33360,10.);
#5060=VECTOR('',#33361,10.);
#5061=VECTOR('',#33364,10.);
#5062=VECTOR('',#33365,10.);
#5063=VECTOR('',#33368,10.);
#5064=VECTOR('',#33371,10.);
#5065=VECTOR('',#33372,10.);
#5066=VECTOR('',#33375,10.);
#5067=VECTOR('',#33376,10.);
#5068=VECTOR('',#33379,10.);
#5069=VECTOR('',#33382,10.);
#5070=VECTOR('',#33383,10.);
#5071=VECTOR('',#33386,10.);
#5072=VECTOR('',#33387,10.);
#5073=VECTOR('',#33390,10.);
#5074=VECTOR('',#33393,10.);
#5075=VECTOR('',#33394,10.);
#5076=VECTOR('',#33397,10.);
#5077=VECTOR('',#33398,10.);
#5078=VECTOR('',#33401,10.);
#5079=VECTOR('',#33404,10.);
#5080=VECTOR('',#33405,10.);
#5081=VECTOR('',#33408,10.);
#5082=VECTOR('',#33409,10.);
#5083=VECTOR('',#33412,10.);
#5084=VECTOR('',#33413,10.);
#5085=VECTOR('',#33416,10.);
#5086=VECTOR('',#33419,10.);
#5087=VECTOR('',#33420,10.);
#5088=VECTOR('',#33423,10.);
#5089=VECTOR('',#33426,10.);
#5090=VECTOR('',#33427,10.);
#5091=VECTOR('',#33430,10.);
#5092=VECTOR('',#33431,10.);
#5093=VECTOR('',#33434,10.);
#5094=VECTOR('',#33437,10.);
#5095=VECTOR('',#33438,10.);
#5096=VECTOR('',#33441,10.);
#5097=VECTOR('',#33442,10.);
#5098=VECTOR('',#33445,10.);
#5099=VECTOR('',#33448,10.);
#5100=VECTOR('',#33449,10.);
#5101=VECTOR('',#33452,10.);
#5102=VECTOR('',#33453,10.);
#5103=VECTOR('',#33456,10.);
#5104=VECTOR('',#33459,10.);
#5105=VECTOR('',#33460,10.);
#5106=VECTOR('',#33463,10.);
#5107=VECTOR('',#33464,10.);
#5108=VECTOR('',#33467,10.);
#5109=VECTOR('',#33470,10.);
#5110=VECTOR('',#33471,10.);
#5111=VECTOR('',#33474,10.);
#5112=VECTOR('',#33475,10.);
#5113=VECTOR('',#33478,10.);
#5114=VECTOR('',#33481,10.);
#5115=VECTOR('',#33482,10.);
#5116=VECTOR('',#33485,10.);
#5117=VECTOR('',#33486,10.);
#5118=VECTOR('',#33489,10.);
#5119=VECTOR('',#33492,10.);
#5120=VECTOR('',#33493,10.);
#5121=VECTOR('',#33496,10.);
#5122=VECTOR('',#33497,10.);
#5123=VECTOR('',#33500,10.);
#5124=VECTOR('',#33503,10.);
#5125=VECTOR('',#33504,10.);
#5126=VECTOR('',#33507,10.);
#5127=VECTOR('',#33508,10.);
#5128=VECTOR('',#33511,10.);
#5129=VECTOR('',#33514,10.);
#5130=VECTOR('',#33515,10.);
#5131=VECTOR('',#33518,10.);
#5132=VECTOR('',#33519,10.);
#5133=VECTOR('',#33522,10.);
#5134=VECTOR('',#33525,10.);
#5135=VECTOR('',#33526,10.);
#5136=VECTOR('',#33529,10.);
#5137=VECTOR('',#33530,10.);
#5138=VECTOR('',#33533,10.);
#5139=VECTOR('',#33536,10.);
#5140=VECTOR('',#33537,10.);
#5141=VECTOR('',#33540,10.);
#5142=VECTOR('',#33541,10.);
#5143=VECTOR('',#33544,10.);
#5144=VECTOR('',#33547,10.);
#5145=VECTOR('',#33548,10.);
#5146=VECTOR('',#33551,10.);
#5147=VECTOR('',#33552,10.);
#5148=VECTOR('',#33555,10.);
#5149=VECTOR('',#33558,10.);
#5150=VECTOR('',#33559,10.);
#5151=VECTOR('',#33562,10.);
#5152=VECTOR('',#33563,10.);
#5153=VECTOR('',#33566,10.);
#5154=VECTOR('',#33569,10.);
#5155=VECTOR('',#33570,10.);
#5156=VECTOR('',#33573,10.);
#5157=VECTOR('',#33574,10.);
#5158=VECTOR('',#33577,10.);
#5159=VECTOR('',#33580,10.);
#5160=VECTOR('',#33581,10.);
#5161=VECTOR('',#33584,10.);
#5162=VECTOR('',#33585,10.);
#5163=VECTOR('',#33588,10.);
#5164=VECTOR('',#33591,10.);
#5165=VECTOR('',#33592,10.);
#5166=VECTOR('',#33595,10.);
#5167=VECTOR('',#33596,10.);
#5168=VECTOR('',#33599,10.);
#5169=VECTOR('',#33602,10.);
#5170=VECTOR('',#33603,10.);
#5171=VECTOR('',#33606,10.);
#5172=VECTOR('',#33607,10.);
#5173=VECTOR('',#33610,10.);
#5174=VECTOR('',#33613,10.);
#5175=VECTOR('',#33614,10.);
#5176=VECTOR('',#33617,10.);
#5177=VECTOR('',#33618,10.);
#5178=VECTOR('',#33621,10.);
#5179=VECTOR('',#33624,10.);
#5180=VECTOR('',#33625,10.);
#5181=VECTOR('',#33628,10.);
#5182=VECTOR('',#33629,10.);
#5183=VECTOR('',#33632,10.);
#5184=VECTOR('',#33635,10.);
#5185=VECTOR('',#33636,10.);
#5186=VECTOR('',#33639,10.);
#5187=VECTOR('',#33640,10.);
#5188=VECTOR('',#33643,10.);
#5189=VECTOR('',#33646,10.);
#5190=VECTOR('',#33647,10.);
#5191=VECTOR('',#33650,10.);
#5192=VECTOR('',#33651,10.);
#5193=VECTOR('',#33654,10.);
#5194=VECTOR('',#33657,10.);
#5195=VECTOR('',#33658,10.);
#5196=VECTOR('',#33661,10.);
#5197=VECTOR('',#33662,10.);
#5198=VECTOR('',#33665,10.);
#5199=VECTOR('',#33668,10.);
#5200=VECTOR('',#33669,10.);
#5201=VECTOR('',#33672,10.);
#5202=VECTOR('',#33673,10.);
#5203=VECTOR('',#33676,10.);
#5204=VECTOR('',#33679,10.);
#5205=VECTOR('',#33680,10.);
#5206=VECTOR('',#33683,10.);
#5207=VECTOR('',#33684,10.);
#5208=VECTOR('',#33687,10.);
#5209=VECTOR('',#33690,10.);
#5210=VECTOR('',#33691,10.);
#5211=VECTOR('',#33692,10.);
#5212=VECTOR('',#33693,10.);
#5213=VECTOR('',#33696,10.);
#5214=VECTOR('',#33697,10.);
#5215=VECTOR('',#33700,10.);
#5216=VECTOR('',#33701,10.);
#5217=VECTOR('',#33702,10.);
#5218=VECTOR('',#33703,10.);
#5219=VECTOR('',#33704,10.);
#5220=VECTOR('',#33705,10.);
#5221=VECTOR('',#33706,10.);
#5222=VECTOR('',#33707,10.);
#5223=VECTOR('',#33708,10.);
#5224=VECTOR('',#33709,10.);
#5225=VECTOR('',#33710,10.);
#5226=VECTOR('',#33711,10.);
#5227=VECTOR('',#33712,10.);
#5228=VECTOR('',#33713,10.);
#5229=VECTOR('',#33714,10.);
#5230=VECTOR('',#33715,10.);
#5231=VECTOR('',#33716,10.);
#5232=VECTOR('',#33717,10.);
#5233=VECTOR('',#33718,10.);
#5234=VECTOR('',#33719,10.);
#5235=VECTOR('',#33720,10.);
#5236=VECTOR('',#33721,10.);
#5237=VECTOR('',#33722,10.);
#5238=VECTOR('',#33723,10.);
#5239=VECTOR('',#33724,10.);
#5240=VECTOR('',#33725,10.);
#5241=VECTOR('',#33726,10.);
#5242=VECTOR('',#33727,10.);
#5243=VECTOR('',#33728,10.);
#5244=VECTOR('',#33729,10.);
#5245=VECTOR('',#33730,10.);
#5246=VECTOR('',#33731,10.);
#5247=VECTOR('',#33732,10.);
#5248=VECTOR('',#33733,10.);
#5249=VECTOR('',#33734,10.);
#5250=VECTOR('',#33735,10.);
#5251=VECTOR('',#33736,10.);
#5252=VECTOR('',#33737,10.);
#5253=VECTOR('',#33738,10.);
#5254=VECTOR('',#33739,10.);
#5255=VECTOR('',#33740,10.);
#5256=VECTOR('',#33741,10.);
#5257=VECTOR('',#33742,10.);
#5258=VECTOR('',#33743,10.);
#5259=VECTOR('',#33744,10.);
#5260=VECTOR('',#33745,10.);
#5261=VECTOR('',#33746,10.);
#5262=VECTOR('',#33747,10.);
#5263=VECTOR('',#33748,10.);
#5264=VECTOR('',#33749,10.);
#5265=VECTOR('',#33750,10.);
#5266=VECTOR('',#33751,10.);
#5267=VECTOR('',#33752,10.);
#5268=VECTOR('',#33753,10.);
#5269=VECTOR('',#33754,10.);
#5270=VECTOR('',#33755,10.);
#5271=VECTOR('',#33756,10.);
#5272=VECTOR('',#33757,10.);
#5273=VECTOR('',#33758,10.);
#5274=VECTOR('',#33759,10.);
#5275=VECTOR('',#33760,10.);
#5276=VECTOR('',#33761,10.);
#5277=VECTOR('',#33762,10.);
#5278=VECTOR('',#33763,10.);
#5279=VECTOR('',#33764,10.);
#5280=VECTOR('',#33765,10.);
#5281=VECTOR('',#33766,10.);
#5282=VECTOR('',#33767,10.);
#5283=VECTOR('',#33768,10.);
#5284=VECTOR('',#33769,10.);
#5285=VECTOR('',#33770,10.);
#5286=VECTOR('',#33771,10.);
#5287=VECTOR('',#33772,10.);
#5288=VECTOR('',#33773,10.);
#5289=VECTOR('',#33774,10.);
#5290=VECTOR('',#33775,10.);
#5291=VECTOR('',#33776,10.);
#5292=VECTOR('',#33777,10.);
#5293=VECTOR('',#33778,10.);
#5294=VECTOR('',#33779,10.);
#5295=VECTOR('',#33780,10.);
#5296=VECTOR('',#33781,10.);
#5297=VECTOR('',#33782,10.);
#5298=VECTOR('',#33783,10.);
#5299=VECTOR('',#33784,10.);
#5300=VECTOR('',#33785,10.);
#5301=VECTOR('',#33786,10.);
#5302=VECTOR('',#33787,10.);
#5303=VECTOR('',#33788,10.);
#5304=VECTOR('',#33789,10.);
#5305=VECTOR('',#33790,10.);
#5306=VECTOR('',#33793,10.);
#5307=VECTOR('',#33794,10.);
#5308=VECTOR('',#33795,10.);
#5309=VECTOR('',#33800,10.);
#5310=VECTOR('',#33803,10.);
#5311=VECTOR('',#33804,10.);
#5312=VECTOR('',#33805,10.);
#5313=VECTOR('',#33808,10.);
#5314=VECTOR('',#33811,10.);
#5315=VECTOR('',#33814,10.);
#5316=VECTOR('',#33815,10.);
#5317=VECTOR('',#33816,10.);
#5318=VECTOR('',#33819,10.);
#5319=VECTOR('',#33822,10.);
#5320=VECTOR('',#33825,10.);
#5321=VECTOR('',#33826,10.);
#5322=VECTOR('',#33829,10.);
#5323=VECTOR('',#33830,10.);
#5324=VECTOR('',#33833,10.);
#5325=VECTOR('',#33834,10.);
#5326=VECTOR('',#33835,10.);
#5327=VECTOR('',#33838,10.);
#5328=VECTOR('',#33841,10.);
#5329=VECTOR('',#33844,10.);
#5330=VECTOR('',#33845,10.);
#5331=VECTOR('',#33846,10.);
#5332=VECTOR('',#33849,10.);
#5333=VECTOR('',#33852,10.);
#5334=VECTOR('',#33855,10.);
#5335=VECTOR('',#33856,10.);
#5336=VECTOR('',#33859,10.);
#5337=VECTOR('',#33860,10.);
#5338=VECTOR('',#33863,10.);
#5339=VECTOR('',#33864,10.);
#5340=VECTOR('',#33865,10.);
#5341=VECTOR('',#33868,10.);
#5342=VECTOR('',#33871,10.);
#5343=VECTOR('',#33874,10.);
#5344=VECTOR('',#33875,10.);
#5345=VECTOR('',#33876,10.);
#5346=VECTOR('',#33879,10.);
#5347=VECTOR('',#33882,10.);
#5348=VECTOR('',#33885,10.);
#5349=VECTOR('',#33886,10.);
#5350=VECTOR('',#33889,10.);
#5351=VECTOR('',#33890,10.);
#5352=VECTOR('',#33893,10.);
#5353=VECTOR('',#33894,10.);
#5354=VECTOR('',#33897,10.);
#5355=VECTOR('',#33898,10.);
#5356=VECTOR('',#33901,10.);
#5357=VECTOR('',#33904,10.);
#5358=VECTOR('',#33905,10.);
#5359=VECTOR('',#33906,10.);
#5360=VECTOR('',#33909,10.);
#5361=VECTOR('',#33912,10.);
#5362=VECTOR('',#33915,10.);
#5363=VECTOR('',#33916,10.);
#5364=VECTOR('',#33917,10.);
#5365=VECTOR('',#33920,10.);
#5366=VECTOR('',#33923,10.);
#5367=VECTOR('',#33926,10.);
#5368=VECTOR('',#33927,10.);
#5369=VECTOR('',#33930,10.);
#5370=VECTOR('',#33931,10.);
#5371=VECTOR('',#33934,10.);
#5372=VECTOR('',#33935,10.);
#5373=VECTOR('',#33936,10.);
#5374=VECTOR('',#33939,10.);
#5375=VECTOR('',#33942,10.);
#5376=VECTOR('',#33945,10.);
#5377=VECTOR('',#33946,10.);
#5378=VECTOR('',#33947,10.);
#5379=VECTOR('',#33950,10.);
#5380=VECTOR('',#33953,10.);
#5381=VECTOR('',#33956,10.);
#5382=VECTOR('',#33957,10.);
#5383=VECTOR('',#33960,10.);
#5384=VECTOR('',#33961,10.);
#5385=VECTOR('',#33964,10.);
#5386=VECTOR('',#33965,10.);
#5387=VECTOR('',#33966,10.);
#5388=VECTOR('',#33969,10.);
#5389=VECTOR('',#33972,10.);
#5390=VECTOR('',#33975,10.);
#5391=VECTOR('',#33976,10.);
#5392=VECTOR('',#33977,10.);
#5393=VECTOR('',#33980,10.);
#5394=VECTOR('',#33983,10.);
#5395=VECTOR('',#33986,10.);
#5396=VECTOR('',#33987,10.);
#5397=VECTOR('',#33990,10.);
#5398=VECTOR('',#33991,10.);
#5399=VECTOR('',#33994,10.);
#5400=VECTOR('',#33995,10.);
#5401=VECTOR('',#33996,10.);
#5402=VECTOR('',#33999,10.);
#5403=VECTOR('',#34002,10.);
#5404=VECTOR('',#34005,10.);
#5405=VECTOR('',#34006,10.);
#5406=VECTOR('',#34007,10.);
#5407=VECTOR('',#34010,10.);
#5408=VECTOR('',#34013,10.);
#5409=VECTOR('',#34016,10.);
#5410=VECTOR('',#34017,10.);
#5411=VECTOR('',#34020,10.);
#5412=VECTOR('',#34021,10.);
#5413=VECTOR('',#34024,10.);
#5414=VECTOR('',#34025,10.);
#5415=VECTOR('',#34026,10.);
#5416=VECTOR('',#34029,10.);
#5417=VECTOR('',#34032,10.);
#5418=VECTOR('',#34035,10.);
#5419=VECTOR('',#34036,10.);
#5420=VECTOR('',#34037,10.);
#5421=VECTOR('',#34040,10.);
#5422=VECTOR('',#34043,10.);
#5423=VECTOR('',#34046,10.);
#5424=VECTOR('',#34047,10.);
#5425=VECTOR('',#34050,10.);
#5426=VECTOR('',#34051,10.);
#5427=VECTOR('',#34054,10.);
#5428=VECTOR('',#34055,10.);
#5429=VECTOR('',#34056,10.);
#5430=VECTOR('',#34059,10.);
#5431=VECTOR('',#34062,10.);
#5432=VECTOR('',#34065,10.);
#5433=VECTOR('',#34066,10.);
#5434=VECTOR('',#34067,10.);
#5435=VECTOR('',#34070,10.);
#5436=VECTOR('',#34073,10.);
#5437=VECTOR('',#34076,10.);
#5438=VECTOR('',#34077,10.);
#5439=VECTOR('',#34080,10.);
#5440=VECTOR('',#34081,10.);
#5441=VECTOR('',#34084,10.);
#5442=VECTOR('',#34085,10.);
#5443=VECTOR('',#34086,10.);
#5444=VECTOR('',#34089,10.);
#5445=VECTOR('',#34092,10.);
#5446=VECTOR('',#34095,10.);
#5447=VECTOR('',#34096,10.);
#5448=VECTOR('',#34097,10.);
#5449=VECTOR('',#34100,10.);
#5450=VECTOR('',#34103,10.);
#5451=VECTOR('',#34106,10.);
#5452=VECTOR('',#34107,10.);
#5453=VECTOR('',#34108,10.);
#5454=VECTOR('',#34111,10.);
#5455=VECTOR('',#34114,10.);
#5456=VECTOR('',#34117,10.);
#5457=VECTOR('',#34118,10.);
#5458=VECTOR('',#34121,10.);
#5459=VECTOR('',#34122,10.);
#5460=VECTOR('',#34125,10.);
#5461=VECTOR('',#34126,10.);
#5462=VECTOR('',#34127,10.);
#5463=VECTOR('',#34130,10.);
#5464=VECTOR('',#34133,10.);
#5465=VECTOR('',#34136,10.);
#5466=VECTOR('',#34137,10.);
#5467=VECTOR('',#34138,10.);
#5468=VECTOR('',#34141,10.);
#5469=VECTOR('',#34144,10.);
#5470=VECTOR('',#34147,10.);
#5471=VECTOR('',#34148,10.);
#5472=VECTOR('',#34151,10.);
#5473=VECTOR('',#34152,10.);
#5474=VECTOR('',#34155,10.);
#5475=VECTOR('',#34156,10.);
#5476=VECTOR('',#34157,10.);
#5477=VECTOR('',#34160,10.);
#5478=VECTOR('',#34163,10.);
#5479=VECTOR('',#34166,10.);
#5480=VECTOR('',#34167,10.);
#5481=VECTOR('',#34168,10.);
#5482=VECTOR('',#34171,10.);
#5483=VECTOR('',#34174,10.);
#5484=VECTOR('',#34177,10.);
#5485=VECTOR('',#34178,10.);
#5486=VECTOR('',#34181,10.);
#5487=VECTOR('',#34182,10.);
#5488=VECTOR('',#34185,10.);
#5489=VECTOR('',#34186,10.);
#5490=VECTOR('',#34189,10.);
#5491=VECTOR('',#34190,10.);
#5492=VECTOR('',#34193,10.);
#5493=VECTOR('',#34196,10.);
#5494=VECTOR('',#34197,10.);
#5495=VECTOR('',#34198,10.);
#5496=VECTOR('',#34201,10.);
#5497=VECTOR('',#34204,10.);
#5498=VECTOR('',#34207,10.);
#5499=VECTOR('',#34208,10.);
#5500=VECTOR('',#34209,10.);
#5501=VECTOR('',#34212,10.);
#5502=VECTOR('',#34215,10.);
#5503=VECTOR('',#34218,10.);
#5504=VECTOR('',#34219,10.);
#5505=VECTOR('',#34222,10.);
#5506=VECTOR('',#34223,10.);
#5507=VECTOR('',#34226,10.);
#5508=VECTOR('',#34227,10.);
#5509=VECTOR('',#34228,10.);
#5510=VECTOR('',#34233,10.);
#5511=VECTOR('',#34236,10.);
#5512=VECTOR('',#34241,10.);
#5513=VECTOR('',#34242,10.);
#5514=VECTOR('',#34243,10.);
#5515=VECTOR('',#34246,10.);
#5516=VECTOR('',#34247,10.);
#5517=VECTOR('',#34250,10.);
#5518=VECTOR('',#34251,10.);
#5519=VECTOR('',#34256,10.);
#5520=VECTOR('',#34263,10.);
#5521=VECTOR('',#34264,10.);
#5522=VECTOR('',#34273,10.);
#5523=VECTOR('',#34276,10.);
#5524=VECTOR('',#34279,10.);
#5525=VECTOR('',#34280,10.);
#5526=VECTOR('',#34283,10.);
#5527=VECTOR('',#34286,10.);
#5528=VECTOR('',#34287,10.);
#5529=VECTOR('',#34288,10.);
#5530=VECTOR('',#34291,10.);
#5531=VECTOR('',#34292,10.);
#5532=VECTOR('',#34295,10.);
#5533=VECTOR('',#34300,10.);
#5534=VECTOR('',#34303,10.);
#5535=VECTOR('',#34310,10.);
#5536=VECTOR('',#34317,10.);
#5537=VECTOR('',#34318,10.);
#5538=VECTOR('',#34319,10.);
#5539=VECTOR('',#34322,10.);
#5540=VECTOR('',#34325,10.);
#5541=VECTOR('',#34332,10.);
#5542=VECTOR('',#34333,10.);
#5543=VECTOR('',#34334,10.);
#5544=VECTOR('',#34337,10.);
#5545=VECTOR('',#34340,10.);
#5546=VECTOR('',#34347,10.);
#5547=VECTOR('',#34354,10.);
#5548=VECTOR('',#34355,10.);
#5549=VECTOR('',#34356,10.);
#5550=VECTOR('',#34359,10.);
#5551=VECTOR('',#34362,10.);
#5552=VECTOR('',#34369,10.);
#5553=VECTOR('',#34376,10.);
#5554=VECTOR('',#34377,10.);
#5555=VECTOR('',#34378,10.);
#5556=VECTOR('',#34381,10.);
#5557=VECTOR('',#34384,10.);
#5558=VECTOR('',#34391,10.);
#5559=VECTOR('',#34398,10.);
#5560=VECTOR('',#34399,10.);
#5561=VECTOR('',#34400,10.);
#5562=VECTOR('',#34403,10.);
#5563=VECTOR('',#34406,10.);
#5564=VECTOR('',#34413,10.);
#5565=VECTOR('',#34414,10.);
#5566=VECTOR('',#34415,10.);
#5567=VECTOR('',#34418,10.);
#5568=VECTOR('',#34421,10.);
#5569=VECTOR('',#34428,10.);
#5570=VECTOR('',#34435,10.);
#5571=VECTOR('',#34436,10.);
#5572=VECTOR('',#34437,10.);
#5573=VECTOR('',#34440,10.);
#5574=VECTOR('',#34443,10.);
#5575=VECTOR('',#34450,10.);
#5576=VECTOR('',#34457,10.);
#5577=VECTOR('',#34458,10.);
#5578=VECTOR('',#34459,10.);
#5579=VECTOR('',#34462,10.);
#5580=VECTOR('',#34465,10.);
#5581=VECTOR('',#34472,10.);
#5582=VECTOR('',#34479,10.);
#5583=VECTOR('',#34480,10.);
#5584=VECTOR('',#34481,10.);
#5585=VECTOR('',#34484,10.);
#5586=VECTOR('',#34487,10.);
#5587=VECTOR('',#34494,10.);
#5588=VECTOR('',#34501,10.);
#5589=VECTOR('',#34502,10.);
#5590=VECTOR('',#34503,10.);
#5591=VECTOR('',#34506,10.);
#5592=VECTOR('',#34509,10.);
#5593=VECTOR('',#34516,10.);
#5594=VECTOR('',#34521,10.);
#5595=VECTOR('',#34526,10.);
#5596=VECTOR('',#34527,10.);
#5597=VECTOR('',#34528,10.);
#5598=VECTOR('',#34531,10.);
#5599=VECTOR('',#34534,10.);
#5600=VECTOR('',#34541,10.);
#5601=VECTOR('',#34548,10.);
#5602=VECTOR('',#34549,10.);
#5603=VECTOR('',#34550,10.);
#5604=VECTOR('',#34553,10.);
#5605=VECTOR('',#34556,10.);
#5606=VECTOR('',#34563,10.);
#5607=VECTOR('',#34564,10.);
#5608=VECTOR('',#34565,10.);
#5609=VECTOR('',#34568,10.);
#5610=VECTOR('',#34571,10.);
#5611=VECTOR('',#34576,10.);
#5612=VECTOR('',#34581,10.);
#5613=VECTOR('',#34586,10.);
#5614=VECTOR('',#34587,10.);
#5615=VECTOR('',#34590,10.);
#5616=VECTOR('',#34591,10.);
#5617=VECTOR('',#34594,10.);
#5618=VECTOR('',#34599,10.);
#5619=VECTOR('',#34600,10.);
#5620=VECTOR('',#34601,10.);
#5621=VECTOR('',#34604,10.);
#5622=VECTOR('',#34607,10.);
#5623=VECTOR('',#34612,10.);
#5624=VECTOR('',#34613,10.);
#5625=VECTOR('',#34616,10.);
#5626=VECTOR('',#34617,10.);
#5627=VECTOR('',#34620,10.);
#5628=VECTOR('',#34625,10.);
#5629=VECTOR('',#34630,10.);
#5630=VECTOR('',#34631,10.);
#5631=VECTOR('',#34634,10.);
#5632=VECTOR('',#34635,10.);
#5633=VECTOR('',#34638,10.);
#5634=VECTOR('',#34643,10.);
#5635=VECTOR('',#34644,10.);
#5636=VECTOR('',#34645,10.);
#5637=VECTOR('',#34648,10.);
#5638=VECTOR('',#34651,10.);
#5639=VECTOR('',#34656,10.);
#5640=VECTOR('',#34657,10.);
#5641=VECTOR('',#34660,10.);
#5642=VECTOR('',#34661,10.);
#5643=VECTOR('',#34664,10.);
#5644=VECTOR('',#34669,10.);
#5645=VECTOR('',#34674,10.);
#5646=VECTOR('',#34675,10.);
#5647=VECTOR('',#34678,10.);
#5648=VECTOR('',#34679,10.);
#5649=VECTOR('',#34682,10.);
#5650=VECTOR('',#34687,10.);
#5651=VECTOR('',#34688,10.);
#5652=VECTOR('',#34689,10.);
#5653=VECTOR('',#34692,10.);
#5654=VECTOR('',#34695,10.);
#5655=VECTOR('',#34700,10.);
#5656=VECTOR('',#34701,10.);
#5657=VECTOR('',#34704,10.);
#5658=VECTOR('',#34705,10.);
#5659=VECTOR('',#34708,10.);
#5660=VECTOR('',#34713,10.);
#5661=VECTOR('',#34714,10.);
#5662=VECTOR('',#34715,10.);
#5663=VECTOR('',#34718,10.);
#5664=VECTOR('',#34721,10.);
#6672=CYLINDRICAL_SURFACE('',#28375,70.);
#6673=CYLINDRICAL_SURFACE('',#28905,10.01);
#6674=CYLINDRICAL_SURFACE('',#29068,10.01);
#7349=FACE_OUTER_BOUND('',#8995,.T.);
#7350=FACE_OUTER_BOUND('',#8996,.T.);
#7351=FACE_OUTER_BOUND('',#8997,.T.);
#7352=FACE_OUTER_BOUND('',#8998,.T.);
#7353=FACE_OUTER_BOUND('',#8999,.T.);
#7354=FACE_OUTER_BOUND('',#9000,.T.);
#7355=FACE_OUTER_BOUND('',#9001,.T.);
#7356=FACE_OUTER_BOUND('',#9002,.T.);
#7357=FACE_OUTER_BOUND('',#9003,.T.);
#7358=FACE_OUTER_BOUND('',#9004,.T.);
#7359=FACE_OUTER_BOUND('',#9005,.T.);
#7360=FACE_OUTER_BOUND('',#9006,.T.);
#7361=FACE_OUTER_BOUND('',#9007,.T.);
#7362=FACE_OUTER_BOUND('',#9008,.T.);
#7363=FACE_OUTER_BOUND('',#9009,.T.);
#7364=FACE_OUTER_BOUND('',#9010,.T.);
#7365=FACE_OUTER_BOUND('',#9011,.T.);
#7366=FACE_OUTER_BOUND('',#9012,.T.);
#7367=FACE_OUTER_BOUND('',#9013,.T.);
#7368=FACE_OUTER_BOUND('',#9014,.T.);
#7369=FACE_OUTER_BOUND('',#9015,.T.);
#7370=FACE_OUTER_BOUND('',#9016,.T.);
#7371=FACE_OUTER_BOUND('',#9017,.T.);
#7372=FACE_OUTER_BOUND('',#9018,.T.);
#7373=FACE_OUTER_BOUND('',#9019,.T.);
#7374=FACE_OUTER_BOUND('',#9020,.T.);
#7375=FACE_OUTER_BOUND('',#9021,.T.);
#7376=FACE_OUTER_BOUND('',#9023,.T.);
#7377=FACE_OUTER_BOUND('',#9024,.T.);
#7378=FACE_OUTER_BOUND('',#9025,.T.);
#7379=FACE_OUTER_BOUND('',#9026,.T.);
#7380=FACE_OUTER_BOUND('',#9027,.T.);
#7381=FACE_OUTER_BOUND('',#9028,.T.);
#7382=FACE_OUTER_BOUND('',#9029,.T.);
#7383=FACE_OUTER_BOUND('',#9030,.T.);
#7384=FACE_OUTER_BOUND('',#9031,.T.);
#7385=FACE_OUTER_BOUND('',#9032,.T.);
#7386=FACE_OUTER_BOUND('',#9033,.T.);
#7387=FACE_OUTER_BOUND('',#9034,.T.);
#7388=FACE_OUTER_BOUND('',#9035,.T.);
#7389=FACE_OUTER_BOUND('',#9036,.T.);
#7390=FACE_OUTER_BOUND('',#9037,.T.);
#7391=FACE_OUTER_BOUND('',#9038,.T.);
#7392=FACE_OUTER_BOUND('',#9039,.T.);
#7393=FACE_OUTER_BOUND('',#9040,.T.);
#7394=FACE_OUTER_BOUND('',#9041,.T.);
#7395=FACE_OUTER_BOUND('',#9042,.T.);
#7396=FACE_OUTER_BOUND('',#9043,.T.);
#7397=FACE_OUTER_BOUND('',#9044,.T.);
#7398=FACE_OUTER_BOUND('',#9045,.T.);
#7399=FACE_OUTER_BOUND('',#9046,.T.);
#7400=FACE_OUTER_BOUND('',#9047,.T.);
#7401=FACE_OUTER_BOUND('',#9048,.T.);
#7402=FACE_OUTER_BOUND('',#9049,.T.);
#7403=FACE_OUTER_BOUND('',#9050,.T.);
#7404=FACE_OUTER_BOUND('',#9051,.T.);
#7405=FACE_OUTER_BOUND('',#9052,.T.);
#7406=FACE_OUTER_BOUND('',#9053,.T.);
#7407=FACE_OUTER_BOUND('',#9054,.T.);
#7408=FACE_OUTER_BOUND('',#9055,.T.);
#7409=FACE_OUTER_BOUND('',#9056,.T.);
#7410=FACE_OUTER_BOUND('',#9057,.T.);
#7411=FACE_OUTER_BOUND('',#9058,.T.);
#7412=FACE_OUTER_BOUND('',#9059,.T.);
#7413=FACE_OUTER_BOUND('',#9060,.T.);
#7414=FACE_OUTER_BOUND('',#9061,.T.);
#7415=FACE_OUTER_BOUND('',#9062,.T.);
#7416=FACE_OUTER_BOUND('',#9063,.T.);
#7417=FACE_OUTER_BOUND('',#9064,.T.);
#7418=FACE_OUTER_BOUND('',#9065,.T.);
#7419=FACE_OUTER_BOUND('',#9066,.T.);
#7420=FACE_OUTER_BOUND('',#9067,.T.);
#7421=FACE_OUTER_BOUND('',#9068,.T.);
#7422=FACE_OUTER_BOUND('',#9069,.T.);
#7423=FACE_OUTER_BOUND('',#9070,.T.);
#7424=FACE_OUTER_BOUND('',#9071,.T.);
#7425=FACE_OUTER_BOUND('',#9072,.T.);
#7426=FACE_OUTER_BOUND('',#9073,.T.);
#7427=FACE_OUTER_BOUND('',#9074,.T.);
#7428=FACE_OUTER_BOUND('',#9075,.T.);
#7429=FACE_OUTER_BOUND('',#9076,.T.);
#7430=FACE_OUTER_BOUND('',#9077,.T.);
#7431=FACE_OUTER_BOUND('',#9078,.T.);
#7432=FACE_OUTER_BOUND('',#9079,.T.);
#7433=FACE_OUTER_BOUND('',#9080,.T.);
#7434=FACE_OUTER_BOUND('',#9081,.T.);
#7435=FACE_OUTER_BOUND('',#9082,.T.);
#7436=FACE_OUTER_BOUND('',#9083,.T.);
#7437=FACE_OUTER_BOUND('',#9084,.T.);
#7438=FACE_OUTER_BOUND('',#9085,.T.);
#7439=FACE_OUTER_BOUND('',#9086,.T.);
#7440=FACE_OUTER_BOUND('',#9087,.T.);
#7441=FACE_OUTER_BOUND('',#9088,.T.);
#7442=FACE_OUTER_BOUND('',#9089,.T.);
#7443=FACE_OUTER_BOUND('',#9090,.T.);
#7444=FACE_OUTER_BOUND('',#9091,.T.);
#7445=FACE_OUTER_BOUND('',#9092,.T.);
#7446=FACE_OUTER_BOUND('',#9093,.T.);
#7447=FACE_OUTER_BOUND('',#9094,.T.);
#7448=FACE_OUTER_BOUND('',#9095,.T.);
#7449=FACE_OUTER_BOUND('',#9096,.T.);
#7450=FACE_OUTER_BOUND('',#9097,.T.);
#7451=FACE_OUTER_BOUND('',#9098,.T.);
#7452=FACE_OUTER_BOUND('',#9099,.T.);
#7453=FACE_OUTER_BOUND('',#9100,.T.);
#7454=FACE_OUTER_BOUND('',#9101,.T.);
#7455=FACE_OUTER_BOUND('',#9102,.T.);
#7456=FACE_OUTER_BOUND('',#9103,.T.);
#7457=FACE_OUTER_BOUND('',#9104,.T.);
#7458=FACE_OUTER_BOUND('',#9105,.T.);
#7459=FACE_OUTER_BOUND('',#9106,.T.);
#7460=FACE_OUTER_BOUND('',#9107,.T.);
#7461=FACE_OUTER_BOUND('',#9108,.T.);
#7462=FACE_OUTER_BOUND('',#9109,.T.);
#7463=FACE_OUTER_BOUND('',#9110,.T.);
#7464=FACE_OUTER_BOUND('',#9111,.T.);
#7465=FACE_OUTER_BOUND('',#9112,.T.);
#7466=FACE_OUTER_BOUND('',#9113,.T.);
#7467=FACE_OUTER_BOUND('',#9114,.T.);
#7468=FACE_OUTER_BOUND('',#9115,.T.);
#7469=FACE_OUTER_BOUND('',#9116,.T.);
#7470=FACE_OUTER_BOUND('',#9117,.T.);
#7471=FACE_OUTER_BOUND('',#9118,.T.);
#7472=FACE_OUTER_BOUND('',#9119,.T.);
#7473=FACE_OUTER_BOUND('',#9120,.T.);
#7474=FACE_OUTER_BOUND('',#9121,.T.);
#7475=FACE_OUTER_BOUND('',#9122,.T.);
#7476=FACE_OUTER_BOUND('',#9123,.T.);
#7477=FACE_OUTER_BOUND('',#9124,.T.);
#7478=FACE_OUTER_BOUND('',#9125,.T.);
#7479=FACE_OUTER_BOUND('',#9126,.T.);
#7480=FACE_OUTER_BOUND('',#9127,.T.);
#7481=FACE_OUTER_BOUND('',#9128,.T.);
#7482=FACE_OUTER_BOUND('',#9129,.T.);
#7483=FACE_OUTER_BOUND('',#9130,.T.);
#7484=FACE_OUTER_BOUND('',#9131,.T.);
#7485=FACE_OUTER_BOUND('',#9132,.T.);
#7486=FACE_OUTER_BOUND('',#9133,.T.);
#7487=FACE_OUTER_BOUND('',#9134,.T.);
#7488=FACE_OUTER_BOUND('',#9135,.T.);
#7489=FACE_OUTER_BOUND('',#9136,.T.);
#7490=FACE_OUTER_BOUND('',#9137,.T.);
#7491=FACE_OUTER_BOUND('',#9138,.T.);
#7492=FACE_OUTER_BOUND('',#9139,.T.);
#7493=FACE_OUTER_BOUND('',#9140,.T.);
#7494=FACE_OUTER_BOUND('',#9141,.T.);
#7495=FACE_OUTER_BOUND('',#9142,.T.);
#7496=FACE_OUTER_BOUND('',#9143,.T.);
#7497=FACE_OUTER_BOUND('',#9144,.T.);
#7498=FACE_OUTER_BOUND('',#9145,.T.);
#7499=FACE_OUTER_BOUND('',#9146,.T.);
#7500=FACE_OUTER_BOUND('',#9147,.T.);
#7501=FACE_OUTER_BOUND('',#9148,.T.);
#7502=FACE_OUTER_BOUND('',#9149,.T.);
#7503=FACE_OUTER_BOUND('',#9150,.T.);
#7504=FACE_OUTER_BOUND('',#9151,.T.);
#7505=FACE_OUTER_BOUND('',#9152,.T.);
#7506=FACE_OUTER_BOUND('',#9153,.T.);
#7507=FACE_OUTER_BOUND('',#9154,.T.);
#7508=FACE_OUTER_BOUND('',#9155,.T.);
#7509=FACE_OUTER_BOUND('',#9156,.T.);
#7510=FACE_OUTER_BOUND('',#9157,.T.);
#7511=FACE_OUTER_BOUND('',#9158,.T.);
#7512=FACE_OUTER_BOUND('',#9159,.T.);
#7513=FACE_OUTER_BOUND('',#9160,.T.);
#7514=FACE_OUTER_BOUND('',#9162,.T.);
#7515=FACE_OUTER_BOUND('',#9163,.T.);
#7516=FACE_OUTER_BOUND('',#9164,.T.);
#7517=FACE_OUTER_BOUND('',#9165,.T.);
#7518=FACE_OUTER_BOUND('',#9166,.T.);
#7519=FACE_OUTER_BOUND('',#9167,.T.);
#7520=FACE_OUTER_BOUND('',#9168,.T.);
#7521=FACE_OUTER_BOUND('',#9169,.T.);
#7522=FACE_OUTER_BOUND('',#9170,.T.);
#7523=FACE_OUTER_BOUND('',#9171,.T.);
#7524=FACE_OUTER_BOUND('',#9172,.T.);
#7525=FACE_OUTER_BOUND('',#9173,.T.);
#7526=FACE_OUTER_BOUND('',#9174,.T.);
#7527=FACE_OUTER_BOUND('',#9175,.T.);
#7528=FACE_OUTER_BOUND('',#9176,.T.);
#7529=FACE_OUTER_BOUND('',#9177,.T.);
#7530=FACE_OUTER_BOUND('',#9178,.T.);
#7531=FACE_OUTER_BOUND('',#9179,.T.);
#7532=FACE_OUTER_BOUND('',#9180,.T.);
#7533=FACE_OUTER_BOUND('',#9181,.T.);
#7534=FACE_OUTER_BOUND('',#9182,.T.);
#7535=FACE_OUTER_BOUND('',#9183,.T.);
#7536=FACE_OUTER_BOUND('',#9184,.T.);
#7537=FACE_OUTER_BOUND('',#9185,.T.);
#7538=FACE_OUTER_BOUND('',#9186,.T.);
#7539=FACE_OUTER_BOUND('',#9187,.T.);
#7540=FACE_OUTER_BOUND('',#9188,.T.);
#7541=FACE_OUTER_BOUND('',#9189,.T.);
#7542=FACE_OUTER_BOUND('',#9190,.T.);
#7543=FACE_OUTER_BOUND('',#9191,.T.);
#7544=FACE_OUTER_BOUND('',#9192,.T.);
#7545=FACE_OUTER_BOUND('',#9193,.T.);
#7546=FACE_OUTER_BOUND('',#9194,.T.);
#7547=FACE_OUTER_BOUND('',#9195,.T.);
#7548=FACE_OUTER_BOUND('',#9196,.T.);
#7549=FACE_OUTER_BOUND('',#9197,.T.);
#7550=FACE_OUTER_BOUND('',#9198,.T.);
#7551=FACE_OUTER_BOUND('',#9199,.T.);
#7552=FACE_OUTER_BOUND('',#9200,.T.);
#7553=FACE_OUTER_BOUND('',#9201,.T.);
#7554=FACE_OUTER_BOUND('',#9202,.T.);
#7555=FACE_OUTER_BOUND('',#9203,.T.);
#7556=FACE_OUTER_BOUND('',#9204,.T.);
#7557=FACE_OUTER_BOUND('',#9205,.T.);
#7558=FACE_OUTER_BOUND('',#9206,.T.);
#7559=FACE_OUTER_BOUND('',#9207,.T.);
#7560=FACE_OUTER_BOUND('',#9208,.T.);
#7561=FACE_OUTER_BOUND('',#9209,.T.);
#7562=FACE_OUTER_BOUND('',#9210,.T.);
#7563=FACE_OUTER_BOUND('',#9211,.T.);
#7564=FACE_OUTER_BOUND('',#9212,.T.);
#7565=FACE_OUTER_BOUND('',#9213,.T.);
#7566=FACE_OUTER_BOUND('',#9214,.T.);
#7567=FACE_OUTER_BOUND('',#9215,.T.);
#7568=FACE_OUTER_BOUND('',#9216,.T.);
#7569=FACE_OUTER_BOUND('',#9217,.T.);
#7570=FACE_OUTER_BOUND('',#9218,.T.);
#7571=FACE_OUTER_BOUND('',#9219,.T.);
#7572=FACE_OUTER_BOUND('',#9220,.T.);
#7573=FACE_OUTER_BOUND('',#9221,.T.);
#7574=FACE_OUTER_BOUND('',#9222,.T.);
#7575=FACE_OUTER_BOUND('',#9223,.T.);
#7576=FACE_OUTER_BOUND('',#9224,.T.);
#7577=FACE_OUTER_BOUND('',#9225,.T.);
#7578=FACE_OUTER_BOUND('',#9226,.T.);
#7579=FACE_OUTER_BOUND('',#9227,.T.);
#7580=FACE_OUTER_BOUND('',#9228,.T.);
#7581=FACE_OUTER_BOUND('',#9229,.T.);
#7582=FACE_OUTER_BOUND('',#9230,.T.);
#7583=FACE_OUTER_BOUND('',#9231,.T.);
#7584=FACE_OUTER_BOUND('',#9232,.T.);
#7585=FACE_OUTER_BOUND('',#9233,.T.);
#7586=FACE_OUTER_BOUND('',#9234,.T.);
#7587=FACE_OUTER_BOUND('',#9235,.T.);
#7588=FACE_OUTER_BOUND('',#9236,.T.);
#7589=FACE_OUTER_BOUND('',#9237,.T.);
#7590=FACE_OUTER_BOUND('',#9238,.T.);
#7591=FACE_OUTER_BOUND('',#9239,.T.);
#7592=FACE_OUTER_BOUND('',#9240,.T.);
#7593=FACE_OUTER_BOUND('',#9241,.T.);
#7594=FACE_OUTER_BOUND('',#9242,.T.);
#7595=FACE_OUTER_BOUND('',#9243,.T.);
#7596=FACE_OUTER_BOUND('',#9244,.T.);
#7597=FACE_OUTER_BOUND('',#9245,.T.);
#7598=FACE_OUTER_BOUND('',#9246,.T.);
#7599=FACE_OUTER_BOUND('',#9247,.T.);
#7600=FACE_OUTER_BOUND('',#9248,.T.);
#7601=FACE_OUTER_BOUND('',#9249,.T.);
#7602=FACE_OUTER_BOUND('',#9250,.T.);
#7603=FACE_OUTER_BOUND('',#9251,.T.);
#7604=FACE_OUTER_BOUND('',#9252,.T.);
#7605=FACE_OUTER_BOUND('',#9253,.T.);
#7606=FACE_OUTER_BOUND('',#9254,.T.);
#7607=FACE_OUTER_BOUND('',#9255,.T.);
#7608=FACE_OUTER_BOUND('',#9256,.T.);
#7609=FACE_OUTER_BOUND('',#9257,.T.);
#7610=FACE_OUTER_BOUND('',#9258,.T.);
#7611=FACE_OUTER_BOUND('',#9259,.T.);
#7612=FACE_OUTER_BOUND('',#9260,.T.);
#7613=FACE_OUTER_BOUND('',#9261,.T.);
#7614=FACE_OUTER_BOUND('',#9262,.T.);
#7615=FACE_OUTER_BOUND('',#9263,.T.);
#7616=FACE_OUTER_BOUND('',#9264,.T.);
#7617=FACE_OUTER_BOUND('',#9265,.T.);
#7618=FACE_OUTER_BOUND('',#9266,.T.);
#7619=FACE_OUTER_BOUND('',#9267,.T.);
#7620=FACE_OUTER_BOUND('',#9268,.T.);
#7621=FACE_OUTER_BOUND('',#9269,.T.);
#7622=FACE_OUTER_BOUND('',#9270,.T.);
#7623=FACE_OUTER_BOUND('',#9271,.T.);
#7624=FACE_OUTER_BOUND('',#9272,.T.);
#7625=FACE_OUTER_BOUND('',#9273,.T.);
#7626=FACE_OUTER_BOUND('',#9274,.T.);
#7627=FACE_OUTER_BOUND('',#9275,.T.);
#7628=FACE_OUTER_BOUND('',#9276,.T.);
#7629=FACE_OUTER_BOUND('',#9277,.T.);
#7630=FACE_OUTER_BOUND('',#9278,.T.);
#7631=FACE_OUTER_BOUND('',#9279,.T.);
#7632=FACE_OUTER_BOUND('',#9280,.T.);
#7633=FACE_OUTER_BOUND('',#9281,.T.);
#7634=FACE_OUTER_BOUND('',#9282,.T.);
#7635=FACE_OUTER_BOUND('',#9283,.T.);
#7636=FACE_OUTER_BOUND('',#9284,.T.);
#7637=FACE_OUTER_BOUND('',#9285,.T.);
#7638=FACE_OUTER_BOUND('',#9286,.T.);
#7639=FACE_OUTER_BOUND('',#9287,.T.);
#7640=FACE_OUTER_BOUND('',#9288,.T.);
#7641=FACE_OUTER_BOUND('',#9289,.T.);
#7642=FACE_OUTER_BOUND('',#9290,.T.);
#7643=FACE_OUTER_BOUND('',#9291,.T.);
#7644=FACE_OUTER_BOUND('',#9292,.T.);
#7645=FACE_OUTER_BOUND('',#9293,.T.);
#7646=FACE_OUTER_BOUND('',#9294,.T.);
#7647=FACE_OUTER_BOUND('',#9295,.T.);
#7648=FACE_OUTER_BOUND('',#9296,.T.);
#7649=FACE_OUTER_BOUND('',#9297,.T.);
#7650=FACE_OUTER_BOUND('',#9298,.T.);
#7651=FACE_OUTER_BOUND('',#9299,.T.);
#7652=FACE_OUTER_BOUND('',#9300,.T.);
#7653=FACE_OUTER_BOUND('',#9301,.T.);
#7654=FACE_OUTER_BOUND('',#9302,.T.);
#7655=FACE_OUTER_BOUND('',#9303,.T.);
#7656=FACE_OUTER_BOUND('',#9304,.T.);
#7657=FACE_OUTER_BOUND('',#9305,.T.);
#7658=FACE_OUTER_BOUND('',#9306,.T.);
#7659=FACE_OUTER_BOUND('',#9307,.T.);
#7660=FACE_OUTER_BOUND('',#9308,.T.);
#7661=FACE_OUTER_BOUND('',#9309,.T.);
#7662=FACE_OUTER_BOUND('',#9310,.T.);
#7663=FACE_OUTER_BOUND('',#9311,.T.);
#7664=FACE_OUTER_BOUND('',#9312,.T.);
#7665=FACE_OUTER_BOUND('',#9313,.T.);
#7666=FACE_OUTER_BOUND('',#9314,.T.);
#7667=FACE_OUTER_BOUND('',#9315,.T.);
#7668=FACE_OUTER_BOUND('',#9316,.T.);
#7669=FACE_OUTER_BOUND('',#9317,.T.);
#7670=FACE_OUTER_BOUND('',#9318,.T.);
#7671=FACE_OUTER_BOUND('',#9319,.T.);
#7672=FACE_OUTER_BOUND('',#9320,.T.);
#7673=FACE_OUTER_BOUND('',#9321,.T.);
#7674=FACE_OUTER_BOUND('',#9322,.T.);
#7675=FACE_OUTER_BOUND('',#9323,.T.);
#7676=FACE_OUTER_BOUND('',#9324,.T.);
#7677=FACE_OUTER_BOUND('',#9325,.T.);
#7678=FACE_OUTER_BOUND('',#9326,.T.);
#7679=FACE_OUTER_BOUND('',#9327,.T.);
#7680=FACE_OUTER_BOUND('',#9328,.T.);
#7681=FACE_OUTER_BOUND('',#9329,.T.);
#7682=FACE_OUTER_BOUND('',#9330,.T.);
#7683=FACE_OUTER_BOUND('',#9331,.T.);
#7684=FACE_OUTER_BOUND('',#9332,.T.);
#7685=FACE_OUTER_BOUND('',#9333,.T.);
#7686=FACE_OUTER_BOUND('',#9334,.T.);
#7687=FACE_OUTER_BOUND('',#9335,.T.);
#7688=FACE_OUTER_BOUND('',#9336,.T.);
#7689=FACE_OUTER_BOUND('',#9337,.T.);
#7690=FACE_OUTER_BOUND('',#9338,.T.);
#7691=FACE_OUTER_BOUND('',#9339,.T.);
#7692=FACE_OUTER_BOUND('',#9340,.T.);
#7693=FACE_OUTER_BOUND('',#9341,.T.);
#7694=FACE_OUTER_BOUND('',#9342,.T.);
#7695=FACE_OUTER_BOUND('',#9343,.T.);
#7696=FACE_OUTER_BOUND('',#9344,.T.);
#7697=FACE_OUTER_BOUND('',#9345,.T.);
#7698=FACE_OUTER_BOUND('',#9346,.T.);
#7699=FACE_OUTER_BOUND('',#9347,.T.);
#7700=FACE_OUTER_BOUND('',#9348,.T.);
#7701=FACE_OUTER_BOUND('',#9349,.T.);
#7702=FACE_OUTER_BOUND('',#9350,.T.);
#7703=FACE_OUTER_BOUND('',#9351,.T.);
#7704=FACE_OUTER_BOUND('',#9352,.T.);
#7705=FACE_OUTER_BOUND('',#9353,.T.);
#7706=FACE_OUTER_BOUND('',#9354,.T.);
#7707=FACE_OUTER_BOUND('',#9355,.T.);
#7708=FACE_OUTER_BOUND('',#9356,.T.);
#7709=FACE_OUTER_BOUND('',#9357,.T.);
#7710=FACE_OUTER_BOUND('',#9358,.T.);
#7711=FACE_OUTER_BOUND('',#9359,.T.);
#7712=FACE_OUTER_BOUND('',#9360,.T.);
#7713=FACE_OUTER_BOUND('',#9361,.T.);
#7714=FACE_OUTER_BOUND('',#9362,.T.);
#7715=FACE_OUTER_BOUND('',#9363,.T.);
#7716=FACE_OUTER_BOUND('',#9364,.T.);
#7717=FACE_OUTER_BOUND('',#9365,.T.);
#7718=FACE_OUTER_BOUND('',#9366,.T.);
#7719=FACE_OUTER_BOUND('',#9367,.T.);
#7720=FACE_OUTER_BOUND('',#9368,.T.);
#7721=FACE_OUTER_BOUND('',#9369,.T.);
#7722=FACE_OUTER_BOUND('',#9370,.T.);
#7723=FACE_OUTER_BOUND('',#9371,.T.);
#7724=FACE_OUTER_BOUND('',#9372,.T.);
#7725=FACE_OUTER_BOUND('',#9373,.T.);
#7726=FACE_OUTER_BOUND('',#9374,.T.);
#7727=FACE_OUTER_BOUND('',#9375,.T.);
#7728=FACE_OUTER_BOUND('',#9376,.T.);
#7729=FACE_OUTER_BOUND('',#9377,.T.);
#7730=FACE_OUTER_BOUND('',#9378,.T.);
#7731=FACE_OUTER_BOUND('',#9379,.T.);
#7732=FACE_OUTER_BOUND('',#9380,.T.);
#7733=FACE_OUTER_BOUND('',#9381,.T.);
#7734=FACE_OUTER_BOUND('',#9382,.T.);
#7735=FACE_OUTER_BOUND('',#9383,.T.);
#7736=FACE_OUTER_BOUND('',#9384,.T.);
#7737=FACE_OUTER_BOUND('',#9385,.T.);
#7738=FACE_OUTER_BOUND('',#9386,.T.);
#7739=FACE_OUTER_BOUND('',#9387,.T.);
#7740=FACE_OUTER_BOUND('',#9388,.T.);
#7741=FACE_OUTER_BOUND('',#9389,.T.);
#7742=FACE_OUTER_BOUND('',#9390,.T.);
#7743=FACE_OUTER_BOUND('',#9391,.T.);
#7744=FACE_OUTER_BOUND('',#9392,.T.);
#7745=FACE_OUTER_BOUND('',#9393,.T.);
#7746=FACE_OUTER_BOUND('',#9394,.T.);
#7747=FACE_OUTER_BOUND('',#9395,.T.);
#7748=FACE_OUTER_BOUND('',#9396,.T.);
#7749=FACE_OUTER_BOUND('',#9397,.T.);
#7750=FACE_OUTER_BOUND('',#9398,.T.);
#7751=FACE_OUTER_BOUND('',#9399,.T.);
#7752=FACE_OUTER_BOUND('',#9400,.T.);
#7753=FACE_OUTER_BOUND('',#9401,.T.);
#7754=FACE_OUTER_BOUND('',#9402,.T.);
#7755=FACE_OUTER_BOUND('',#9403,.T.);
#7756=FACE_OUTER_BOUND('',#9404,.T.);
#7757=FACE_OUTER_BOUND('',#9405,.T.);
#7758=FACE_OUTER_BOUND('',#9406,.T.);
#7759=FACE_OUTER_BOUND('',#9407,.T.);
#7760=FACE_OUTER_BOUND('',#9408,.T.);
#7761=FACE_OUTER_BOUND('',#9409,.T.);
#7762=FACE_OUTER_BOUND('',#9410,.T.);
#7763=FACE_OUTER_BOUND('',#9411,.T.);
#7764=FACE_OUTER_BOUND('',#9412,.T.);
#7765=FACE_OUTER_BOUND('',#9413,.T.);
#7766=FACE_OUTER_BOUND('',#9414,.T.);
#7767=FACE_OUTER_BOUND('',#9415,.T.);
#7768=FACE_OUTER_BOUND('',#9416,.T.);
#7769=FACE_OUTER_BOUND('',#9417,.T.);
#7770=FACE_OUTER_BOUND('',#9418,.T.);
#7771=FACE_OUTER_BOUND('',#9419,.T.);
#7772=FACE_OUTER_BOUND('',#9420,.T.);
#7773=FACE_OUTER_BOUND('',#9421,.T.);
#7774=FACE_OUTER_BOUND('',#9422,.T.);
#7775=FACE_OUTER_BOUND('',#9423,.T.);
#7776=FACE_OUTER_BOUND('',#9424,.T.);
#7777=FACE_OUTER_BOUND('',#9425,.T.);
#7778=FACE_OUTER_BOUND('',#9426,.T.);
#7779=FACE_OUTER_BOUND('',#9427,.T.);
#7780=FACE_OUTER_BOUND('',#9428,.T.);
#7781=FACE_OUTER_BOUND('',#9429,.T.);
#7782=FACE_OUTER_BOUND('',#9430,.T.);
#7783=FACE_OUTER_BOUND('',#9431,.T.);
#7784=FACE_OUTER_BOUND('',#9432,.T.);
#7785=FACE_OUTER_BOUND('',#9433,.T.);
#7786=FACE_OUTER_BOUND('',#9434,.T.);
#7787=FACE_OUTER_BOUND('',#9435,.T.);
#7788=FACE_OUTER_BOUND('',#9436,.T.);
#7789=FACE_OUTER_BOUND('',#9437,.T.);
#7790=FACE_OUTER_BOUND('',#9438,.T.);
#7791=FACE_OUTER_BOUND('',#9439,.T.);
#8995=EDGE_LOOP('',(#20394,#20395,#20396,#20397));
#8996=EDGE_LOOP('',(#20398,#20399,#20400,#20401));
#8997=EDGE_LOOP('',(#20402,#20403,#20404,#20405,#20406,#20407,#20408,#20409,
#20410,#20411,#20412,#20413,#20414,#20415,#20416,#20417,#20418,#20419,#20420,
#20421,#20422,#20423,#20424,#20425,#20426,#20427,#20428,#20429,#20430,#20431,
#20432,#20433,#20434,#20435,#20436,#20437,#20438,#20439,#20440,#20441,#20442,
#20443,#20444,#20445,#20446,#20447,#20448,#20449,#20450,#20451,#20452,#20453,
#20454,#20455,#20456,#20457,#20458,#20459,#20460,#20461,#20462,#20463,#20464,
#20465,#20466,#20467,#20468,#20469,#20470,#20471,#20472,#20473,#20474,#20475,
#20476,#20477,#20478,#20479,#20480,#20481,#20482,#20483,#20484,#20485,#20486,
#20487,#20488,#20489,#20490,#20491,#20492,#20493,#20494,#20495,#20496,#20497,
#20498,#20499,#20500,#20501,#20502,#20503,#20504,#20505,#20506,#20507,#20508,
#20509,#20510,#20511,#20512,#20513,#20514,#20515,#20516,#20517,#20518,#20519,
#20520,#20521,#20522,#20523,#20524,#20525,#20526,#20527,#20528,#20529,#20530,
#20531,#20532,#20533,#20534,#20535,#20536,#20537,#20538,#20539,#20540,#20541,
#20542,#20543,#20544,#20545,#20546,#20547,#20548,#20549,#20550,#20551,#20552,
#20553,#20554,#20555,#20556,#20557,#20558,#20559,#20560,#20561,#20562,#20563,
#20564,#20565,#20566,#20567,#20568,#20569,#20570,#20571,#20572,#20573,#20574,
#20575,#20576,#20577,#20578,#20579,#20580,#20581,#20582,#20583,#20584,#20585,
#20586,#20587,#20588,#20589,#20590,#20591,#20592,#20593,#20594,#20595,#20596,
#20597,#20598,#20599,#20600,#20601,#20602,#20603,#20604,#20605,#20606,#20607,
#20608,#20609,#20610,#20611,#20612,#20613,#20614,#20615,#20616,#20617,#20618,
#20619,#20620,#20621,#20622,#20623,#20624,#20625,#20626,#20627,#20628,#20629,
#20630,#20631,#20632,#20633,#20634,#20635,#20636,#20637,#20638,#20639,#20640,
#20641,#20642,#20643,#20644,#20645,#20646,#20647,#20648,#20649,#20650,#20651,
#20652,#20653,#20654,#20655,#20656,#20657,#20658,#20659,#20660,#20661,#20662,
#20663,#20664,#20665,#20666,#20667,#20668,#20669,#20670,#20671,#20672,#20673,
#20674,#20675,#20676,#20677,#20678,#20679,#20680,#20681,#20682,#20683,#20684,
#20685,#20686,#20687,#20688,#20689,#20690,#20691,#20692,#20693,#20694,#20695,
#20696,#20697,#20698,#20699,#20700,#20701,#20702,#20703,#20704,#20705,#20706,
#20707,#20708,#20709,#20710,#20711,#20712,#20713,#20714,#20715,#20716,#20717,
#20718,#20719,#20720,#20721,#20722,#20723,#20724,#20725,#20726,#20727,#20728,
#20729,#20730,#20731,#20732,#20733,#20734,#20735,#20736,#20737,#20738,#20739,
#20740,#20741,#20742,#20743,#20744,#20745,#20746,#20747,#20748,#20749,#20750,
#20751,#20752,#20753,#20754,#20755,#20756,#20757,#20758,#20759,#20760,#20761,
#20762,#20763,#20764,#20765));
#8998=EDGE_LOOP('',(#20766,#20767,#20768,#20769));
#8999=EDGE_LOOP('',(#20770,#20771,#20772,#20773));
#9000=EDGE_LOOP('',(#20774,#20775,#20776,#20777));
#9001=EDGE_LOOP('',(#20778,#20779,#20780,#20781));
#9002=EDGE_LOOP('',(#20782,#20783,#20784,#20785));
#9003=EDGE_LOOP('',(#20786,#20787,#20788,#20789));
#9004=EDGE_LOOP('',(#20790,#20791,#20792,#20793));
#9005=EDGE_LOOP('',(#20794,#20795,#20796,#20797));
#9006=EDGE_LOOP('',(#20798,#20799,#20800,#20801));
#9007=EDGE_LOOP('',(#20802,#20803,#20804,#20805));
#9008=EDGE_LOOP('',(#20806,#20807,#20808,#20809));
#9009=EDGE_LOOP('',(#20810,#20811,#20812,#20813));
#9010=EDGE_LOOP('',(#20814,#20815,#20816,#20817));
#9011=EDGE_LOOP('',(#20818,#20819,#20820,#20821));
#9012=EDGE_LOOP('',(#20822,#20823,#20824,#20825));
#9013=EDGE_LOOP('',(#20826,#20827,#20828,#20829));
#9014=EDGE_LOOP('',(#20830,#20831,#20832,#20833));
#9015=EDGE_LOOP('',(#20834,#20835,#20836,#20837));
#9016=EDGE_LOOP('',(#20838,#20839,#20840,#20841));
#9017=EDGE_LOOP('',(#20842,#20843,#20844,#20845));
#9018=EDGE_LOOP('',(#20846,#20847,#20848,#20849));
#9019=EDGE_LOOP('',(#20850,#20851,#20852,#20853));
#9020=EDGE_LOOP('',(#20854,#20855,#20856,#20857));
#9021=EDGE_LOOP('',(#20858,#20859,#20860,#20861,#20862,#20863,#20864,#20865,
#20866,#20867,#20868,#20869,#20870,#20871,#20872,#20873,#20874,#20875,#20876,
#20877,#20878,#20879,#20880,#20881,#20882,#20883,#20884,#20885,#20886,#20887,
#20888,#20889,#20890,#20891,#20892,#20893,#20894,#20895,#20896,#20897,#20898,
#20899,#20900,#20901,#20902,#20903,#20904,#20905,#20906,#20907,#20908,#20909,
#20910,#20911,#20912,#20913,#20914,#20915,#20916,#20917,#20918,#20919,#20920,
#20921,#20922,#20923,#20924,#20925,#20926,#20927,#20928,#20929,#20930,#20931,
#20932,#20933,#20934,#20935,#20936,#20937,#20938,#20939,#20940,#20941,#20942,
#20943,#20944,#20945,#20946,#20947,#20948,#20949,#20950,#20951,#20952,#20953,
#20954,#20955,#20956,#20957,#20958,#20959,#20960,#20961,#20962,#20963,#20964,
#20965,#20966,#20967,#20968,#20969,#20970,#20971,#20972,#20973,#20974,#20975,
#20976,#20977,#20978));
#9022=EDGE_LOOP('',(#20979,#20980,#20981,#20982,#20983,#20984,#20985,#20986));
#9023=EDGE_LOOP('',(#20987,#20988,#20989,#20990));
#9024=EDGE_LOOP('',(#20991,#20992,#20993,#20994));
#9025=EDGE_LOOP('',(#20995,#20996,#20997,#20998));
#9026=EDGE_LOOP('',(#20999,#21000,#21001,#21002));
#9027=EDGE_LOOP('',(#21003,#21004,#21005,#21006));
#9028=EDGE_LOOP('',(#21007,#21008,#21009,#21010));
#9029=EDGE_LOOP('',(#21011,#21012,#21013,#21014));
#9030=EDGE_LOOP('',(#21015,#21016,#21017,#21018));
#9031=EDGE_LOOP('',(#21019,#21020,#21021,#21022));
#9032=EDGE_LOOP('',(#21023,#21024,#21025,#21026));
#9033=EDGE_LOOP('',(#21027,#21028,#21029,#21030));
#9034=EDGE_LOOP('',(#21031,#21032,#21033,#21034));
#9035=EDGE_LOOP('',(#21035,#21036,#21037,#21038));
#9036=EDGE_LOOP('',(#21039,#21040,#21041,#21042));
#9037=EDGE_LOOP('',(#21043,#21044,#21045,#21046));
#9038=EDGE_LOOP('',(#21047,#21048,#21049,#21050));
#9039=EDGE_LOOP('',(#21051,#21052,#21053,#21054));
#9040=EDGE_LOOP('',(#21055,#21056,#21057,#21058));
#9041=EDGE_LOOP('',(#21059,#21060,#21061,#21062));
#9042=EDGE_LOOP('',(#21063,#21064,#21065,#21066));
#9043=EDGE_LOOP('',(#21067,#21068,#21069,#21070));
#9044=EDGE_LOOP('',(#21071,#21072,#21073,#21074));
#9045=EDGE_LOOP('',(#21075,#21076,#21077,#21078));
#9046=EDGE_LOOP('',(#21079,#21080,#21081,#21082));
#9047=EDGE_LOOP('',(#21083,#21084,#21085,#21086));
#9048=EDGE_LOOP('',(#21087,#21088,#21089,#21090));
#9049=EDGE_LOOP('',(#21091,#21092,#21093,#21094));
#9050=EDGE_LOOP('',(#21095,#21096,#21097,#21098));
#9051=EDGE_LOOP('',(#21099,#21100,#21101,#21102));
#9052=EDGE_LOOP('',(#21103,#21104,#21105,#21106));
#9053=EDGE_LOOP('',(#21107,#21108,#21109,#21110));
#9054=EDGE_LOOP('',(#21111,#21112,#21113,#21114));
#9055=EDGE_LOOP('',(#21115,#21116,#21117,#21118));
#9056=EDGE_LOOP('',(#21119,#21120,#21121,#21122));
#9057=EDGE_LOOP('',(#21123,#21124,#21125,#21126));
#9058=EDGE_LOOP('',(#21127,#21128,#21129,#21130));
#9059=EDGE_LOOP('',(#21131,#21132,#21133,#21134));
#9060=EDGE_LOOP('',(#21135,#21136,#21137,#21138));
#9061=EDGE_LOOP('',(#21139,#21140,#21141,#21142));
#9062=EDGE_LOOP('',(#21143,#21144,#21145,#21146));
#9063=EDGE_LOOP('',(#21147,#21148,#21149,#21150));
#9064=EDGE_LOOP('',(#21151,#21152,#21153,#21154));
#9065=EDGE_LOOP('',(#21155,#21156,#21157,#21158));
#9066=EDGE_LOOP('',(#21159,#21160,#21161,#21162));
#9067=EDGE_LOOP('',(#21163,#21164,#21165,#21166));
#9068=EDGE_LOOP('',(#21167,#21168,#21169,#21170));
#9069=EDGE_LOOP('',(#21171,#21172,#21173,#21174));
#9070=EDGE_LOOP('',(#21175,#21176,#21177,#21178));
#9071=EDGE_LOOP('',(#21179,#21180,#21181,#21182));
#9072=EDGE_LOOP('',(#21183,#21184,#21185,#21186));
#9073=EDGE_LOOP('',(#21187,#21188,#21189,#21190));
#9074=EDGE_LOOP('',(#21191,#21192,#21193,#21194));
#9075=EDGE_LOOP('',(#21195,#21196,#21197,#21198));
#9076=EDGE_LOOP('',(#21199,#21200,#21201,#21202));
#9077=EDGE_LOOP('',(#21203,#21204,#21205,#21206));
#9078=EDGE_LOOP('',(#21207,#21208,#21209,#21210));
#9079=EDGE_LOOP('',(#21211,#21212,#21213,#21214));
#9080=EDGE_LOOP('',(#21215,#21216,#21217,#21218));
#9081=EDGE_LOOP('',(#21219,#21220,#21221,#21222));
#9082=EDGE_LOOP('',(#21223,#21224,#21225,#21226));
#9083=EDGE_LOOP('',(#21227,#21228,#21229,#21230));
#9084=EDGE_LOOP('',(#21231,#21232,#21233,#21234));
#9085=EDGE_LOOP('',(#21235,#21236,#21237,#21238));
#9086=EDGE_LOOP('',(#21239,#21240,#21241,#21242));
#9087=EDGE_LOOP('',(#21243,#21244,#21245,#21246));
#9088=EDGE_LOOP('',(#21247,#21248,#21249,#21250));
#9089=EDGE_LOOP('',(#21251,#21252,#21253,#21254));
#9090=EDGE_LOOP('',(#21255,#21256,#21257,#21258));
#9091=EDGE_LOOP('',(#21259,#21260,#21261,#21262));
#9092=EDGE_LOOP('',(#21263,#21264,#21265,#21266));
#9093=EDGE_LOOP('',(#21267,#21268,#21269,#21270));
#9094=EDGE_LOOP('',(#21271,#21272,#21273,#21274));
#9095=EDGE_LOOP('',(#21275,#21276,#21277,#21278));
#9096=EDGE_LOOP('',(#21279,#21280,#21281,#21282));
#9097=EDGE_LOOP('',(#21283,#21284,#21285,#21286));
#9098=EDGE_LOOP('',(#21287,#21288,#21289,#21290));
#9099=EDGE_LOOP('',(#21291,#21292,#21293,#21294));
#9100=EDGE_LOOP('',(#21295,#21296,#21297,#21298));
#9101=EDGE_LOOP('',(#21299,#21300,#21301,#21302));
#9102=EDGE_LOOP('',(#21303,#21304,#21305,#21306));
#9103=EDGE_LOOP('',(#21307,#21308,#21309,#21310));
#9104=EDGE_LOOP('',(#21311,#21312,#21313,#21314));
#9105=EDGE_LOOP('',(#21315,#21316,#21317,#21318));
#9106=EDGE_LOOP('',(#21319,#21320,#21321,#21322));
#9107=EDGE_LOOP('',(#21323,#21324,#21325,#21326));
#9108=EDGE_LOOP('',(#21327,#21328,#21329,#21330));
#9109=EDGE_LOOP('',(#21331,#21332,#21333,#21334));
#9110=EDGE_LOOP('',(#21335,#21336,#21337,#21338));
#9111=EDGE_LOOP('',(#21339,#21340,#21341,#21342));
#9112=EDGE_LOOP('',(#21343,#21344,#21345,#21346));
#9113=EDGE_LOOP('',(#21347,#21348,#21349,#21350));
#9114=EDGE_LOOP('',(#21351,#21352,#21353,#21354));
#9115=EDGE_LOOP('',(#21355,#21356,#21357,#21358));
#9116=EDGE_LOOP('',(#21359,#21360,#21361,#21362));
#9117=EDGE_LOOP('',(#21363,#21364,#21365,#21366));
#9118=EDGE_LOOP('',(#21367,#21368,#21369,#21370));
#9119=EDGE_LOOP('',(#21371,#21372,#21373,#21374));
#9120=EDGE_LOOP('',(#21375,#21376,#21377,#21378));
#9121=EDGE_LOOP('',(#21379,#21380,#21381,#21382));
#9122=EDGE_LOOP('',(#21383,#21384,#21385,#21386));
#9123=EDGE_LOOP('',(#21387,#21388,#21389,#21390));
#9124=EDGE_LOOP('',(#21391,#21392,#21393,#21394));
#9125=EDGE_LOOP('',(#21395,#21396,#21397,#21398));
#9126=EDGE_LOOP('',(#21399,#21400,#21401,#21402));
#9127=EDGE_LOOP('',(#21403,#21404,#21405,#21406));
#9128=EDGE_LOOP('',(#21407,#21408,#21409,#21410));
#9129=EDGE_LOOP('',(#21411,#21412,#21413,#21414));
#9130=EDGE_LOOP('',(#21415,#21416,#21417,#21418));
#9131=EDGE_LOOP('',(#21419,#21420,#21421,#21422));
#9132=EDGE_LOOP('',(#21423,#21424,#21425,#21426));
#9133=EDGE_LOOP('',(#21427,#21428,#21429,#21430));
#9134=EDGE_LOOP('',(#21431,#21432,#21433,#21434));
#9135=EDGE_LOOP('',(#21435,#21436,#21437,#21438));
#9136=EDGE_LOOP('',(#21439,#21440,#21441,#21442));
#9137=EDGE_LOOP('',(#21443,#21444,#21445,#21446));
#9138=EDGE_LOOP('',(#21447,#21448,#21449,#21450));
#9139=EDGE_LOOP('',(#21451,#21452,#21453,#21454));
#9140=EDGE_LOOP('',(#21455,#21456,#21457,#21458));
#9141=EDGE_LOOP('',(#21459,#21460,#21461,#21462));
#9142=EDGE_LOOP('',(#21463,#21464,#21465,#21466));
#9143=EDGE_LOOP('',(#21467,#21468,#21469,#21470));
#9144=EDGE_LOOP('',(#21471,#21472,#21473,#21474));
#9145=EDGE_LOOP('',(#21475,#21476,#21477,#21478));
#9146=EDGE_LOOP('',(#21479,#21480,#21481,#21482));
#9147=EDGE_LOOP('',(#21483,#21484,#21485,#21486));
#9148=EDGE_LOOP('',(#21487,#21488,#21489,#21490));
#9149=EDGE_LOOP('',(#21491,#21492,#21493,#21494));
#9150=EDGE_LOOP('',(#21495,#21496,#21497,#21498));
#9151=EDGE_LOOP('',(#21499,#21500,#21501,#21502));
#9152=EDGE_LOOP('',(#21503,#21504,#21505,#21506));
#9153=EDGE_LOOP('',(#21507,#21508,#21509,#21510));
#9154=EDGE_LOOP('',(#21511,#21512,#21513,#21514));
#9155=EDGE_LOOP('',(#21515,#21516,#21517,#21518));
#9156=EDGE_LOOP('',(#21519,#21520,#21521,#21522));
#9157=EDGE_LOOP('',(#21523,#21524,#21525,#21526));
#9158=EDGE_LOOP('',(#21527,#21528,#21529,#21530));
#9159=EDGE_LOOP('',(#21531,#21532,#21533,#21534));
#9160=EDGE_LOOP('',(#21535,#21536,#21537,#21538,#21539,#21540,#21541,#21542,
#21543,#21544,#21545,#21546,#21547,#21548,#21549,#21550,#21551,#21552,#21553,
#21554,#21555,#21556,#21557,#21558,#21559,#21560,#21561,#21562,#21563,#21564,
#21565,#21566,#21567,#21568,#21569,#21570,#21571,#21572,#21573,#21574,#21575,
#21576,#21577,#21578,#21579,#21580,#21581,#21582,#21583,#21584,#21585,#21586,
#21587,#21588,#21589,#21590,#21591,#21592,#21593,#21594,#21595,#21596,#21597,
#21598,#21599,#21600,#21601,#21602,#21603,#21604,#21605,#21606,#21607,#21608,
#21609,#21610,#21611,#21612,#21613,#21614,#21615,#21616,#21617,#21618,#21619,
#21620,#21621,#21622,#21623,#21624,#21625,#21626,#21627,#21628,#21629,#21630,
#21631,#21632,#21633,#21634,#21635,#21636,#21637,#21638,#21639,#21640,#21641,
#21642,#21643,#21644,#21645,#21646,#21647,#21648,#21649,#21650,#21651,#21652,
#21653,#21654,#21655));
#9161=EDGE_LOOP('',(#21656,#21657,#21658,#21659,#21660,#21661,#21662,#21663));
#9162=EDGE_LOOP('',(#21664,#21665,#21666,#21667));
#9163=EDGE_LOOP('',(#21668,#21669,#21670,#21671));
#9164=EDGE_LOOP('',(#21672,#21673,#21674,#21675));
#9165=EDGE_LOOP('',(#21676,#21677,#21678,#21679));
#9166=EDGE_LOOP('',(#21680,#21681,#21682,#21683));
#9167=EDGE_LOOP('',(#21684,#21685,#21686,#21687));
#9168=EDGE_LOOP('',(#21688,#21689,#21690,#21691));
#9169=EDGE_LOOP('',(#21692,#21693,#21694,#21695));
#9170=EDGE_LOOP('',(#21696,#21697,#21698,#21699));
#9171=EDGE_LOOP('',(#21700,#21701,#21702,#21703));
#9172=EDGE_LOOP('',(#21704,#21705,#21706,#21707));
#9173=EDGE_LOOP('',(#21708,#21709,#21710,#21711));
#9174=EDGE_LOOP('',(#21712,#21713,#21714,#21715));
#9175=EDGE_LOOP('',(#21716,#21717,#21718,#21719));
#9176=EDGE_LOOP('',(#21720,#21721,#21722,#21723));
#9177=EDGE_LOOP('',(#21724,#21725,#21726,#21727));
#9178=EDGE_LOOP('',(#21728,#21729,#21730,#21731));
#9179=EDGE_LOOP('',(#21732,#21733,#21734,#21735));
#9180=EDGE_LOOP('',(#21736,#21737,#21738,#21739));
#9181=EDGE_LOOP('',(#21740,#21741,#21742,#21743));
#9182=EDGE_LOOP('',(#21744,#21745,#21746,#21747));
#9183=EDGE_LOOP('',(#21748,#21749,#21750,#21751));
#9184=EDGE_LOOP('',(#21752,#21753,#21754,#21755));
#9185=EDGE_LOOP('',(#21756,#21757,#21758,#21759));
#9186=EDGE_LOOP('',(#21760,#21761,#21762,#21763));
#9187=EDGE_LOOP('',(#21764,#21765,#21766,#21767));
#9188=EDGE_LOOP('',(#21768,#21769,#21770,#21771));
#9189=EDGE_LOOP('',(#21772,#21773,#21774,#21775));
#9190=EDGE_LOOP('',(#21776,#21777,#21778,#21779));
#9191=EDGE_LOOP('',(#21780,#21781,#21782,#21783));
#9192=EDGE_LOOP('',(#21784,#21785,#21786,#21787));
#9193=EDGE_LOOP('',(#21788,#21789,#21790,#21791));
#9194=EDGE_LOOP('',(#21792,#21793,#21794,#21795));
#9195=EDGE_LOOP('',(#21796,#21797,#21798,#21799));
#9196=EDGE_LOOP('',(#21800,#21801,#21802,#21803));
#9197=EDGE_LOOP('',(#21804,#21805,#21806,#21807));
#9198=EDGE_LOOP('',(#21808,#21809,#21810,#21811));
#9199=EDGE_LOOP('',(#21812,#21813,#21814,#21815));
#9200=EDGE_LOOP('',(#21816,#21817,#21818,#21819));
#9201=EDGE_LOOP('',(#21820,#21821,#21822,#21823));
#9202=EDGE_LOOP('',(#21824,#21825,#21826,#21827));
#9203=EDGE_LOOP('',(#21828,#21829,#21830,#21831));
#9204=EDGE_LOOP('',(#21832,#21833,#21834,#21835));
#9205=EDGE_LOOP('',(#21836,#21837,#21838,#21839));
#9206=EDGE_LOOP('',(#21840,#21841,#21842,#21843));
#9207=EDGE_LOOP('',(#21844,#21845,#21846,#21847));
#9208=EDGE_LOOP('',(#21848,#21849,#21850,#21851));
#9209=EDGE_LOOP('',(#21852,#21853,#21854,#21855));
#9210=EDGE_LOOP('',(#21856,#21857,#21858,#21859));
#9211=EDGE_LOOP('',(#21860,#21861,#21862,#21863));
#9212=EDGE_LOOP('',(#21864,#21865,#21866,#21867));
#9213=EDGE_LOOP('',(#21868,#21869,#21870,#21871));
#9214=EDGE_LOOP('',(#21872,#21873,#21874,#21875));
#9215=EDGE_LOOP('',(#21876,#21877,#21878,#21879));
#9216=EDGE_LOOP('',(#21880,#21881,#21882,#21883));
#9217=EDGE_LOOP('',(#21884,#21885,#21886,#21887));
#9218=EDGE_LOOP('',(#21888,#21889,#21890,#21891));
#9219=EDGE_LOOP('',(#21892,#21893,#21894,#21895));
#9220=EDGE_LOOP('',(#21896,#21897,#21898,#21899));
#9221=EDGE_LOOP('',(#21900,#21901,#21902,#21903));
#9222=EDGE_LOOP('',(#21904,#21905,#21906,#21907));
#9223=EDGE_LOOP('',(#21908,#21909,#21910,#21911));
#9224=EDGE_LOOP('',(#21912,#21913,#21914,#21915));
#9225=EDGE_LOOP('',(#21916,#21917,#21918,#21919));
#9226=EDGE_LOOP('',(#21920,#21921,#21922,#21923));
#9227=EDGE_LOOP('',(#21924,#21925,#21926,#21927));
#9228=EDGE_LOOP('',(#21928,#21929,#21930,#21931));
#9229=EDGE_LOOP('',(#21932,#21933,#21934,#21935));
#9230=EDGE_LOOP('',(#21936,#21937,#21938,#21939));
#9231=EDGE_LOOP('',(#21940,#21941,#21942,#21943));
#9232=EDGE_LOOP('',(#21944,#21945,#21946,#21947));
#9233=EDGE_LOOP('',(#21948,#21949,#21950,#21951));
#9234=EDGE_LOOP('',(#21952,#21953,#21954,#21955));
#9235=EDGE_LOOP('',(#21956,#21957,#21958,#21959));
#9236=EDGE_LOOP('',(#21960,#21961,#21962,#21963));
#9237=EDGE_LOOP('',(#21964,#21965,#21966,#21967));
#9238=EDGE_LOOP('',(#21968,#21969,#21970,#21971));
#9239=EDGE_LOOP('',(#21972,#21973,#21974,#21975));
#9240=EDGE_LOOP('',(#21976,#21977,#21978,#21979));
#9241=EDGE_LOOP('',(#21980,#21981,#21982,#21983));
#9242=EDGE_LOOP('',(#21984,#21985,#21986,#21987));
#9243=EDGE_LOOP('',(#21988,#21989,#21990,#21991));
#9244=EDGE_LOOP('',(#21992,#21993,#21994,#21995));
#9245=EDGE_LOOP('',(#21996,#21997,#21998,#21999));
#9246=EDGE_LOOP('',(#22000,#22001,#22002,#22003));
#9247=EDGE_LOOP('',(#22004,#22005,#22006,#22007));
#9248=EDGE_LOOP('',(#22008,#22009,#22010,#22011));
#9249=EDGE_LOOP('',(#22012,#22013,#22014,#22015));
#9250=EDGE_LOOP('',(#22016,#22017,#22018,#22019));
#9251=EDGE_LOOP('',(#22020,#22021,#22022,#22023));
#9252=EDGE_LOOP('',(#22024,#22025,#22026,#22027));
#9253=EDGE_LOOP('',(#22028,#22029,#22030,#22031));
#9254=EDGE_LOOP('',(#22032,#22033,#22034,#22035));
#9255=EDGE_LOOP('',(#22036,#22037,#22038,#22039));
#9256=EDGE_LOOP('',(#22040,#22041,#22042,#22043));
#9257=EDGE_LOOP('',(#22044,#22045,#22046,#22047));
#9258=EDGE_LOOP('',(#22048,#22049,#22050,#22051));
#9259=EDGE_LOOP('',(#22052,#22053,#22054,#22055));
#9260=EDGE_LOOP('',(#22056,#22057,#22058,#22059));
#9261=EDGE_LOOP('',(#22060,#22061,#22062,#22063));
#9262=EDGE_LOOP('',(#22064,#22065,#22066,#22067));
#9263=EDGE_LOOP('',(#22068,#22069,#22070,#22071));
#9264=EDGE_LOOP('',(#22072,#22073,#22074,#22075));
#9265=EDGE_LOOP('',(#22076,#22077,#22078,#22079));
#9266=EDGE_LOOP('',(#22080,#22081,#22082,#22083));
#9267=EDGE_LOOP('',(#22084,#22085,#22086,#22087));
#9268=EDGE_LOOP('',(#22088,#22089,#22090,#22091));
#9269=EDGE_LOOP('',(#22092,#22093,#22094,#22095));
#9270=EDGE_LOOP('',(#22096,#22097,#22098,#22099));
#9271=EDGE_LOOP('',(#22100,#22101,#22102,#22103));
#9272=EDGE_LOOP('',(#22104,#22105,#22106,#22107));
#9273=EDGE_LOOP('',(#22108,#22109,#22110,#22111));
#9274=EDGE_LOOP('',(#22112,#22113,#22114,#22115));
#9275=EDGE_LOOP('',(#22116,#22117,#22118,#22119));
#9276=EDGE_LOOP('',(#22120,#22121,#22122,#22123));
#9277=EDGE_LOOP('',(#22124,#22125,#22126,#22127));
#9278=EDGE_LOOP('',(#22128,#22129,#22130,#22131));
#9279=EDGE_LOOP('',(#22132,#22133,#22134,#22135));
#9280=EDGE_LOOP('',(#22136,#22137,#22138,#22139));
#9281=EDGE_LOOP('',(#22140,#22141,#22142,#22143));
#9282=EDGE_LOOP('',(#22144,#22145,#22146,#22147,#22148,#22149,#22150,#22151));
#9283=EDGE_LOOP('',(#22152,#22153,#22154,#22155));
#9284=EDGE_LOOP('',(#22156,#22157,#22158,#22159));
#9285=EDGE_LOOP('',(#22160,#22161,#22162,#22163));
#9286=EDGE_LOOP('',(#22164,#22165,#22166,#22167));
#9287=EDGE_LOOP('',(#22168,#22169,#22170,#22171));
#9288=EDGE_LOOP('',(#22172,#22173,#22174,#22175));
#9289=EDGE_LOOP('',(#22176,#22177,#22178,#22179));
#9290=EDGE_LOOP('',(#22180,#22181,#22182,#22183));
#9291=EDGE_LOOP('',(#22184,#22185,#22186,#22187));
#9292=EDGE_LOOP('',(#22188,#22189,#22190,#22191));
#9293=EDGE_LOOP('',(#22192,#22193,#22194,#22195));
#9294=EDGE_LOOP('',(#22196,#22197,#22198,#22199));
#9295=EDGE_LOOP('',(#22200,#22201,#22202,#22203));
#9296=EDGE_LOOP('',(#22204,#22205,#22206,#22207));
#9297=EDGE_LOOP('',(#22208,#22209,#22210,#22211));
#9298=EDGE_LOOP('',(#22212,#22213,#22214,#22215));
#9299=EDGE_LOOP('',(#22216,#22217,#22218,#22219));
#9300=EDGE_LOOP('',(#22220,#22221,#22222,#22223));
#9301=EDGE_LOOP('',(#22224,#22225,#22226,#22227));
#9302=EDGE_LOOP('',(#22228,#22229,#22230,#22231));
#9303=EDGE_LOOP('',(#22232,#22233,#22234,#22235));
#9304=EDGE_LOOP('',(#22236,#22237,#22238,#22239));
#9305=EDGE_LOOP('',(#22240,#22241,#22242,#22243));
#9306=EDGE_LOOP('',(#22244,#22245,#22246,#22247));
#9307=EDGE_LOOP('',(#22248,#22249,#22250,#22251));
#9308=EDGE_LOOP('',(#22252,#22253,#22254,#22255));
#9309=EDGE_LOOP('',(#22256,#22257,#22258,#22259));
#9310=EDGE_LOOP('',(#22260,#22261,#22262,#22263));
#9311=EDGE_LOOP('',(#22264,#22265,#22266,#22267));
#9312=EDGE_LOOP('',(#22268,#22269,#22270,#22271));
#9313=EDGE_LOOP('',(#22272,#22273,#22274,#22275));
#9314=EDGE_LOOP('',(#22276,#22277,#22278,#22279));
#9315=EDGE_LOOP('',(#22280,#22281,#22282,#22283));
#9316=EDGE_LOOP('',(#22284,#22285,#22286,#22287));
#9317=EDGE_LOOP('',(#22288,#22289,#22290,#22291));
#9318=EDGE_LOOP('',(#22292,#22293,#22294,#22295));
#9319=EDGE_LOOP('',(#22296,#22297,#22298,#22299));
#9320=EDGE_LOOP('',(#22300,#22301,#22302,#22303));
#9321=EDGE_LOOP('',(#22304,#22305,#22306,#22307));
#9322=EDGE_LOOP('',(#22308,#22309,#22310,#22311));
#9323=EDGE_LOOP('',(#22312,#22313,#22314,#22315));
#9324=EDGE_LOOP('',(#22316,#22317,#22318,#22319));
#9325=EDGE_LOOP('',(#22320,#22321,#22322,#22323));
#9326=EDGE_LOOP('',(#22324,#22325,#22326,#22327));
#9327=EDGE_LOOP('',(#22328,#22329,#22330,#22331));
#9328=EDGE_LOOP('',(#22332,#22333,#22334,#22335));
#9329=EDGE_LOOP('',(#22336,#22337,#22338,#22339));
#9330=EDGE_LOOP('',(#22340,#22341,#22342,#22343));
#9331=EDGE_LOOP('',(#22344,#22345,#22346,#22347));
#9332=EDGE_LOOP('',(#22348,#22349,#22350,#22351));
#9333=EDGE_LOOP('',(#22352,#22353,#22354,#22355));
#9334=EDGE_LOOP('',(#22356,#22357,#22358,#22359));
#9335=EDGE_LOOP('',(#22360,#22361,#22362,#22363));
#9336=EDGE_LOOP('',(#22364,#22365,#22366,#22367));
#9337=EDGE_LOOP('',(#22368,#22369,#22370,#22371));
#9338=EDGE_LOOP('',(#22372,#22373,#22374,#22375));
#9339=EDGE_LOOP('',(#22376,#22377,#22378,#22379));
#9340=EDGE_LOOP('',(#22380,#22381,#22382,#22383));
#9341=EDGE_LOOP('',(#22384,#22385,#22386,#22387));
#9342=EDGE_LOOP('',(#22388,#22389,#22390,#22391));
#9343=EDGE_LOOP('',(#22392,#22393,#22394,#22395));
#9344=EDGE_LOOP('',(#22396,#22397,#22398,#22399));
#9345=EDGE_LOOP('',(#22400,#22401,#22402,#22403));
#9346=EDGE_LOOP('',(#22404,#22405,#22406,#22407));
#9347=EDGE_LOOP('',(#22408,#22409,#22410,#22411));
#9348=EDGE_LOOP('',(#22412,#22413,#22414,#22415));
#9349=EDGE_LOOP('',(#22416,#22417,#22418,#22419));
#9350=EDGE_LOOP('',(#22420,#22421,#22422,#22423));
#9351=EDGE_LOOP('',(#22424,#22425,#22426,#22427));
#9352=EDGE_LOOP('',(#22428,#22429,#22430,#22431));
#9353=EDGE_LOOP('',(#22432,#22433,#22434,#22435));
#9354=EDGE_LOOP('',(#22436,#22437,#22438,#22439));
#9355=EDGE_LOOP('',(#22440,#22441,#22442,#22443));
#9356=EDGE_LOOP('',(#22444,#22445,#22446,#22447));
#9357=EDGE_LOOP('',(#22448,#22449,#22450,#22451));
#9358=EDGE_LOOP('',(#22452,#22453,#22454,#22455));
#9359=EDGE_LOOP('',(#22456,#22457,#22458,#22459));
#9360=EDGE_LOOP('',(#22460,#22461,#22462,#22463));
#9361=EDGE_LOOP('',(#22464,#22465,#22466,#22467));
#9362=EDGE_LOOP('',(#22468,#22469,#22470,#22471));
#9363=EDGE_LOOP('',(#22472,#22473,#22474,#22475));
#9364=EDGE_LOOP('',(#22476,#22477,#22478,#22479));
#9365=EDGE_LOOP('',(#22480,#22481,#22482,#22483));
#9366=EDGE_LOOP('',(#22484,#22485,#22486,#22487));
#9367=EDGE_LOOP('',(#22488,#22489,#22490,#22491));
#9368=EDGE_LOOP('',(#22492,#22493,#22494,#22495));
#9369=EDGE_LOOP('',(#22496,#22497,#22498,#22499));
#9370=EDGE_LOOP('',(#22500,#22501,#22502,#22503));
#9371=EDGE_LOOP('',(#22504,#22505,#22506,#22507));
#9372=EDGE_LOOP('',(#22508,#22509,#22510,#22511));
#9373=EDGE_LOOP('',(#22512,#22513,#22514,#22515));
#9374=EDGE_LOOP('',(#22516,#22517,#22518,#22519));
#9375=EDGE_LOOP('',(#22520,#22521,#22522,#22523));
#9376=EDGE_LOOP('',(#22524,#22525,#22526,#22527));
#9377=EDGE_LOOP('',(#22528,#22529,#22530,#22531));
#9378=EDGE_LOOP('',(#22532,#22533,#22534,#22535));
#9379=EDGE_LOOP('',(#22536,#22537,#22538,#22539));
#9380=EDGE_LOOP('',(#22540,#22541,#22542,#22543));
#9381=EDGE_LOOP('',(#22544,#22545,#22546,#22547));
#9382=EDGE_LOOP('',(#22548,#22549,#22550,#22551));
#9383=EDGE_LOOP('',(#22552,#22553,#22554,#22555));
#9384=EDGE_LOOP('',(#22556,#22557,#22558,#22559));
#9385=EDGE_LOOP('',(#22560,#22561,#22562,#22563));
#9386=EDGE_LOOP('',(#22564,#22565,#22566,#22567));
#9387=EDGE_LOOP('',(#22568,#22569,#22570,#22571));
#9388=EDGE_LOOP('',(#22572,#22573,#22574,#22575));
#9389=EDGE_LOOP('',(#22576,#22577,#22578,#22579));
#9390=EDGE_LOOP('',(#22580,#22581,#22582,#22583));
#9391=EDGE_LOOP('',(#22584,#22585,#22586,#22587));
#9392=EDGE_LOOP('',(#22588,#22589,#22590,#22591));
#9393=EDGE_LOOP('',(#22592,#22593,#22594,#22595));
#9394=EDGE_LOOP('',(#22596,#22597,#22598,#22599));
#9395=EDGE_LOOP('',(#22600,#22601,#22602,#22603));
#9396=EDGE_LOOP('',(#22604,#22605,#22606,#22607));
#9397=EDGE_LOOP('',(#22608,#22609,#22610,#22611));
#9398=EDGE_LOOP('',(#22612,#22613,#22614,#22615));
#9399=EDGE_LOOP('',(#22616,#22617,#22618,#22619));
#9400=EDGE_LOOP('',(#22620,#22621,#22622,#22623));
#9401=EDGE_LOOP('',(#22624,#22625,#22626,#22627));
#9402=EDGE_LOOP('',(#22628,#22629,#22630,#22631));
#9403=EDGE_LOOP('',(#22632,#22633,#22634,#22635));
#9404=EDGE_LOOP('',(#22636,#22637,#22638,#22639));
#9405=EDGE_LOOP('',(#22640,#22641,#22642,#22643));
#9406=EDGE_LOOP('',(#22644,#22645,#22646,#22647));
#9407=EDGE_LOOP('',(#22648,#22649,#22650,#22651));
#9408=EDGE_LOOP('',(#22652,#22653,#22654,#22655));
#9409=EDGE_LOOP('',(#22656,#22657,#22658,#22659));
#9410=EDGE_LOOP('',(#22660,#22661,#22662,#22663));
#9411=EDGE_LOOP('',(#22664,#22665,#22666,#22667));
#9412=EDGE_LOOP('',(#22668,#22669,#22670,#22671));
#9413=EDGE_LOOP('',(#22672,#22673,#22674,#22675));
#9414=EDGE_LOOP('',(#22676,#22677,#22678,#22679));
#9415=EDGE_LOOP('',(#22680,#22681,#22682,#22683));
#9416=EDGE_LOOP('',(#22684,#22685,#22686,#22687));
#9417=EDGE_LOOP('',(#22688,#22689,#22690,#22691));
#9418=EDGE_LOOP('',(#22692,#22693,#22694,#22695));
#9419=EDGE_LOOP('',(#22696,#22697,#22698,#22699));
#9420=EDGE_LOOP('',(#22700,#22701,#22702,#22703));
#9421=EDGE_LOOP('',(#22704,#22705,#22706,#22707));
#9422=EDGE_LOOP('',(#22708,#22709,#22710,#22711));
#9423=EDGE_LOOP('',(#22712,#22713,#22714,#22715));
#9424=EDGE_LOOP('',(#22716,#22717,#22718,#22719));
#9425=EDGE_LOOP('',(#22720,#22721,#22722,#22723));
#9426=EDGE_LOOP('',(#22724,#22725,#22726,#22727));
#9427=EDGE_LOOP('',(#22728,#22729,#22730,#22731));
#9428=EDGE_LOOP('',(#22732,#22733,#22734,#22735));
#9429=EDGE_LOOP('',(#22736,#22737,#22738,#22739));
#9430=EDGE_LOOP('',(#22740,#22741,#22742,#22743));
#9431=EDGE_LOOP('',(#22744,#22745,#22746,#22747));
#9432=EDGE_LOOP('',(#22748,#22749,#22750,#22751));
#9433=EDGE_LOOP('',(#22752,#22753,#22754,#22755));
#9434=EDGE_LOOP('',(#22756,#22757,#22758,#22759));
#9435=EDGE_LOOP('',(#22760,#22761,#22762,#22763));
#9436=EDGE_LOOP('',(#22764,#22765,#22766,#22767));
#9437=EDGE_LOOP('',(#22768,#22769,#22770,#22771));
#9438=EDGE_LOOP('',(#22772,#22773,#22774,#22775));
#9439=EDGE_LOOP('',(#22776,#22777,#22778,#22779,#22780,#22781,#22782,#22783));
#10596=CIRCLE('',#28376,70.);
#10597=CIRCLE('',#28378,70.);
#10598=CIRCLE('',#28380,70.);
#10599=CIRCLE('',#28382,70.);
#10600=CIRCLE('',#28384,70.);
#10601=CIRCLE('',#28385,70.);
#10602=CIRCLE('',#28387,70.);
#10603=CIRCLE('',#28389,70.);
#10604=CIRCLE('',#28391,70.);
#10605=CIRCLE('',#28393,70.);
#10606=CIRCLE('',#28395,70.);
#10607=CIRCLE('',#28397,70.);
#10608=CIRCLE('',#28399,70.);
#10609=CIRCLE('',#28401,70.);
#10610=CIRCLE('',#28403,70.);
#10611=CIRCLE('',#28405,70.);
#10612=CIRCLE('',#28407,70.);
#10613=CIRCLE('',#28409,70.);
#10614=CIRCLE('',#28411,70.);
#10615=CIRCLE('',#28413,70.);
#10616=CIRCLE('',#28415,70.);
#10617=CIRCLE('',#28417,70.);
#10618=CIRCLE('',#28419,70.);
#10619=CIRCLE('',#28421,70.);
#10620=CIRCLE('',#28423,70.);
#10621=CIRCLE('',#28425,70.);
#10622=CIRCLE('',#28427,70.);
#10623=CIRCLE('',#28429,70.);
#10624=CIRCLE('',#28431,70.);
#10625=CIRCLE('',#28433,70.);
#10626=CIRCLE('',#28435,70.);
#10627=CIRCLE('',#28437,70.);
#10628=CIRCLE('',#28439,70.);
#10629=CIRCLE('',#28441,70.);
#10630=CIRCLE('',#28443,70.);
#10631=CIRCLE('',#28445,70.);
#10632=CIRCLE('',#28447,70.);
#10633=CIRCLE('',#28449,70.);
#10634=CIRCLE('',#28451,70.);
#10635=CIRCLE('',#28453,70.);
#10636=CIRCLE('',#28455,70.);
#10637=CIRCLE('',#28457,70.);
#10638=CIRCLE('',#28459,70.);
#10639=CIRCLE('',#28461,70.);
#10640=CIRCLE('',#28463,70.);
#10641=CIRCLE('',#28465,70.);
#10642=CIRCLE('',#28467,70.);
#10643=CIRCLE('',#28469,70.);
#10644=CIRCLE('',#28471,70.);
#10645=CIRCLE('',#28473,70.);
#10646=CIRCLE('',#28475,70.);
#10647=CIRCLE('',#28477,70.);
#10648=CIRCLE('',#28479,70.);
#10649=CIRCLE('',#28481,70.);
#10650=CIRCLE('',#28483,70.);
#10651=CIRCLE('',#28485,70.);
#10652=CIRCLE('',#28487,70.);
#10653=CIRCLE('',#28489,70.);
#10654=CIRCLE('',#28491,70.);
#10655=CIRCLE('',#28493,70.);
#10656=CIRCLE('',#28495,70.);
#10657=CIRCLE('',#28497,70.);
#10658=CIRCLE('',#28499,70.);
#10659=CIRCLE('',#28501,70.);
#10660=CIRCLE('',#28503,70.);
#10661=CIRCLE('',#28505,70.);
#10662=CIRCLE('',#28506,70.);
#10663=CIRCLE('',#28508,70.);
#10664=CIRCLE('',#28510,70.);
#10665=CIRCLE('',#28512,70.);
#10666=CIRCLE('',#28514,70.);
#10667=CIRCLE('',#28516,70.);
#10668=CIRCLE('',#28518,70.);
#10669=CIRCLE('',#28520,70.);
#10670=CIRCLE('',#28522,70.);
#10671=CIRCLE('',#28524,70.);
#10672=CIRCLE('',#28526,70.);
#10673=CIRCLE('',#28528,70.);
#10674=CIRCLE('',#28530,70.);
#10675=CIRCLE('',#28532,70.);
#10676=CIRCLE('',#28534,70.);
#10677=CIRCLE('',#28536,70.);
#10678=CIRCLE('',#28538,70.);
#10679=CIRCLE('',#28540,70.);
#10680=CIRCLE('',#28542,70.);
#10681=CIRCLE('',#28544,70.);
#10682=CIRCLE('',#28546,70.);
#10683=CIRCLE('',#28548,70.);
#10684=CIRCLE('',#28550,70.);
#10685=CIRCLE('',#28552,70.);
#10686=CIRCLE('',#28554,70.);
#10687=CIRCLE('',#28556,70.);
#10688=CIRCLE('',#28558,70.);
#10689=CIRCLE('',#28560,70.);
#10690=CIRCLE('',#28562,70.);
#10691=CIRCLE('',#28564,70.);
#10692=CIRCLE('',#28566,70.);
#10693=CIRCLE('',#28568,70.);
#10694=CIRCLE('',#28570,70.);
#10695=CIRCLE('',#28572,70.);
#10696=CIRCLE('',#28574,70.);
#10697=CIRCLE('',#28576,70.);
#10698=CIRCLE('',#28578,70.);
#10699=CIRCLE('',#28580,70.);
#10700=CIRCLE('',#28582,70.);
#10701=CIRCLE('',#28584,70.);
#10702=CIRCLE('',#28586,70.);
#10703=CIRCLE('',#28588,70.);
#10704=CIRCLE('',#28590,70.);
#10705=CIRCLE('',#28592,70.);
#10706=CIRCLE('',#28594,70.);
#10707=CIRCLE('',#28596,70.);
#10708=CIRCLE('',#28598,70.);
#10709=CIRCLE('',#28600,70.);
#10710=CIRCLE('',#28602,70.);
#10711=CIRCLE('',#28604,70.);
#10712=CIRCLE('',#28606,70.);
#10713=CIRCLE('',#28608,70.);
#10714=CIRCLE('',#28610,70.);
#10715=CIRCLE('',#28612,70.);
#10716=CIRCLE('',#28614,70.);
#10717=CIRCLE('',#28616,70.);
#10718=CIRCLE('',#28641,10.01);
#10719=CIRCLE('',#28642,10.01);
#10720=CIRCLE('',#28781,10.01);
#10721=CIRCLE('',#28782,10.01);
#12268=VERTEX_POINT('',#42567);
#12269=VERTEX_POINT('',#42568);
#12270=VERTEX_POINT('',#42570);
#12271=VERTEX_POINT('',#42572);
#12272=VERTEX_POINT('',#42576);
#12273=VERTEX_POINT('',#42578);
#12274=VERTEX_POINT('',#42582);
#12275=VERTEX_POINT('',#42584);
#12276=VERTEX_POINT('',#42586);
#12277=VERTEX_POINT('',#42588);
#12278=VERTEX_POINT('',#42590);
#12279=VERTEX_POINT('',#42592);
#12280=VERTEX_POINT('',#42594);
#12281=VERTEX_POINT('',#42596);
#12282=VERTEX_POINT('',#42598);
#12283=VERTEX_POINT('',#42600);
#12284=VERTEX_POINT('',#42602);
#12285=VERTEX_POINT('',#42604);
#12286=VERTEX_POINT('',#42606);
#12287=VERTEX_POINT('',#42608);
#12288=VERTEX_POINT('',#42610);
#12289=VERTEX_POINT('',#42612);
#12290=VERTEX_POINT('',#42614);
#12291=VERTEX_POINT('',#42616);
#12292=VERTEX_POINT('',#42618);
#12293=VERTEX_POINT('',#42620);
#12294=VERTEX_POINT('',#42622);
#12295=VERTEX_POINT('',#42624);
#12296=VERTEX_POINT('',#42626);
#12297=VERTEX_POINT('',#42628);
#12298=VERTEX_POINT('',#42630);
#12299=VERTEX_POINT('',#42632);
#12300=VERTEX_POINT('',#42634);
#12301=VERTEX_POINT('',#42636);
#12302=VERTEX_POINT('',#42638);
#12303=VERTEX_POINT('',#42640);
#12304=VERTEX_POINT('',#42642);
#12305=VERTEX_POINT('',#42644);
#12306=VERTEX_POINT('',#42646);
#12307=VERTEX_POINT('',#42648);
#12308=VERTEX_POINT('',#42650);
#12309=VERTEX_POINT('',#42652);
#12310=VERTEX_POINT('',#42654);
#12311=VERTEX_POINT('',#42656);
#12312=VERTEX_POINT('',#42658);
#12313=VERTEX_POINT('',#42660);
#12314=VERTEX_POINT('',#42662);
#12315=VERTEX_POINT('',#42664);
#12316=VERTEX_POINT('',#42666);
#12317=VERTEX_POINT('',#42668);
#12318=VERTEX_POINT('',#42670);
#12319=VERTEX_POINT('',#42672);
#12320=VERTEX_POINT('',#42674);
#12321=VERTEX_POINT('',#42676);
#12322=VERTEX_POINT('',#42678);
#12323=VERTEX_POINT('',#42680);
#12324=VERTEX_POINT('',#42682);
#12325=VERTEX_POINT('',#42684);
#12326=VERTEX_POINT('',#42686);
#12327=VERTEX_POINT('',#42688);
#12328=VERTEX_POINT('',#42690);
#12329=VERTEX_POINT('',#42692);
#12330=VERTEX_POINT('',#42694);
#12331=VERTEX_POINT('',#42696);
#12332=VERTEX_POINT('',#42698);
#12333=VERTEX_POINT('',#42700);
#12334=VERTEX_POINT('',#42702);
#12335=VERTEX_POINT('',#42704);
#12336=VERTEX_POINT('',#42706);
#12337=VERTEX_POINT('',#42708);
#12338=VERTEX_POINT('',#42710);
#12339=VERTEX_POINT('',#42712);
#12340=VERTEX_POINT('',#42714);
#12341=VERTEX_POINT('',#42716);
#12342=VERTEX_POINT('',#42718);
#12343=VERTEX_POINT('',#42720);
#12344=VERTEX_POINT('',#42722);
#12345=VERTEX_POINT('',#42724);
#12346=VERTEX_POINT('',#42726);
#12347=VERTEX_POINT('',#42728);
#12348=VERTEX_POINT('',#42730);
#12349=VERTEX_POINT('',#42732);
#12350=VERTEX_POINT('',#42734);
#12351=VERTEX_POINT('',#42736);
#12352=VERTEX_POINT('',#42738);
#12353=VERTEX_POINT('',#42740);
#12354=VERTEX_POINT('',#42742);
#12355=VERTEX_POINT('',#42744);
#12356=VERTEX_POINT('',#42746);
#12357=VERTEX_POINT('',#42748);
#12358=VERTEX_POINT('',#42750);
#12359=VERTEX_POINT('',#42752);
#12360=VERTEX_POINT('',#42754);
#12361=VERTEX_POINT('',#42756);
#12362=VERTEX_POINT('',#42758);
#12363=VERTEX_POINT('',#42760);
#12364=VERTEX_POINT('',#42762);
#12365=VERTEX_POINT('',#42764);
#12366=VERTEX_POINT('',#42766);
#12367=VERTEX_POINT('',#42768);
#12368=VERTEX_POINT('',#42770);
#12369=VERTEX_POINT('',#42772);
#12370=VERTEX_POINT('',#42774);
#12371=VERTEX_POINT('',#42776);
#12372=VERTEX_POINT('',#42778);
#12373=VERTEX_POINT('',#42780);
#12374=VERTEX_POINT('',#42782);
#12375=VERTEX_POINT('',#42784);
#12376=VERTEX_POINT('',#42786);
#12377=VERTEX_POINT('',#42788);
#12378=VERTEX_POINT('',#42790);
#12379=VERTEX_POINT('',#42792);
#12380=VERTEX_POINT('',#42794);
#12381=VERTEX_POINT('',#42796);
#12382=VERTEX_POINT('',#42798);
#12383=VERTEX_POINT('',#42800);
#12384=VERTEX_POINT('',#42802);
#12385=VERTEX_POINT('',#42804);
#12386=VERTEX_POINT('',#42806);
#12387=VERTEX_POINT('',#42808);
#12388=VERTEX_POINT('',#42810);
#12389=VERTEX_POINT('',#42812);
#12390=VERTEX_POINT('',#42814);
#12391=VERTEX_POINT('',#42816);
#12392=VERTEX_POINT('',#42818);
#12393=VERTEX_POINT('',#42820);
#12394=VERTEX_POINT('',#42822);
#12395=VERTEX_POINT('',#42824);
#12396=VERTEX_POINT('',#42826);
#12397=VERTEX_POINT('',#42828);
#12398=VERTEX_POINT('',#42830);
#12399=VERTEX_POINT('',#42832);
#12400=VERTEX_POINT('',#42834);
#12401=VERTEX_POINT('',#42836);
#12402=VERTEX_POINT('',#42838);
#12403=VERTEX_POINT('',#42840);
#12404=VERTEX_POINT('',#42842);
#12405=VERTEX_POINT('',#42844);
#12406=VERTEX_POINT('',#42846);
#12407=VERTEX_POINT('',#42848);
#12408=VERTEX_POINT('',#42850);
#12409=VERTEX_POINT('',#42852);
#12410=VERTEX_POINT('',#42854);
#12411=VERTEX_POINT('',#42856);
#12412=VERTEX_POINT('',#42858);
#12413=VERTEX_POINT('',#42860);
#12414=VERTEX_POINT('',#42862);
#12415=VERTEX_POINT('',#42864);
#12416=VERTEX_POINT('',#42866);
#12417=VERTEX_POINT('',#42868);
#12418=VERTEX_POINT('',#42870);
#12419=VERTEX_POINT('',#42872);
#12420=VERTEX_POINT('',#42874);
#12421=VERTEX_POINT('',#42876);
#12422=VERTEX_POINT('',#42878);
#12423=VERTEX_POINT('',#42880);
#12424=VERTEX_POINT('',#42882);
#12425=VERTEX_POINT('',#42884);
#12426=VERTEX_POINT('',#42886);
#12427=VERTEX_POINT('',#42888);
#12428=VERTEX_POINT('',#42890);
#12429=VERTEX_POINT('',#42892);
#12430=VERTEX_POINT('',#42894);
#12431=VERTEX_POINT('',#42896);
#12432=VERTEX_POINT('',#42898);
#12433=VERTEX_POINT('',#42900);
#12434=VERTEX_POINT('',#42902);
#12435=VERTEX_POINT('',#42904);
#12436=VERTEX_POINT('',#42906);
#12437=VERTEX_POINT('',#42908);
#12438=VERTEX_POINT('',#42910);
#12439=VERTEX_POINT('',#42912);
#12440=VERTEX_POINT('',#42914);
#12441=VERTEX_POINT('',#42916);
#12442=VERTEX_POINT('',#42918);
#12443=VERTEX_POINT('',#42920);
#12444=VERTEX_POINT('',#42922);
#12445=VERTEX_POINT('',#42924);
#12446=VERTEX_POINT('',#42926);
#12447=VERTEX_POINT('',#42928);
#12448=VERTEX_POINT('',#42930);
#12449=VERTEX_POINT('',#42932);
#12450=VERTEX_POINT('',#42934);
#12451=VERTEX_POINT('',#42936);
#12452=VERTEX_POINT('',#42938);
#12453=VERTEX_POINT('',#42940);
#12454=VERTEX_POINT('',#42942);
#12455=VERTEX_POINT('',#42944);
#12456=VERTEX_POINT('',#42946);
#12457=VERTEX_POINT('',#42948);
#12458=VERTEX_POINT('',#42950);
#12459=VERTEX_POINT('',#42952);
#12460=VERTEX_POINT('',#42954);
#12461=VERTEX_POINT('',#42956);
#12462=VERTEX_POINT('',#42958);
#12463=VERTEX_POINT('',#42960);
#12464=VERTEX_POINT('',#42962);
#12465=VERTEX_POINT('',#42964);
#12466=VERTEX_POINT('',#42966);
#12467=VERTEX_POINT('',#42968);
#12468=VERTEX_POINT('',#42971);
#12469=VERTEX_POINT('',#42973);
#12470=VERTEX_POINT('',#42975);
#12471=VERTEX_POINT('',#42977);
#12472=VERTEX_POINT('',#42979);
#12473=VERTEX_POINT('',#42981);
#12474=VERTEX_POINT('',#42983);
#12475=VERTEX_POINT('',#42985);
#12476=VERTEX_POINT('',#42987);
#12477=VERTEX_POINT('',#42989);
#12478=VERTEX_POINT('',#42991);
#12479=VERTEX_POINT('',#42993);
#12480=VERTEX_POINT('',#42995);
#12481=VERTEX_POINT('',#42997);
#12482=VERTEX_POINT('',#42999);
#12483=VERTEX_POINT('',#43001);
#12484=VERTEX_POINT('',#43003);
#12485=VERTEX_POINT('',#43005);
#12486=VERTEX_POINT('',#43007);
#12487=VERTEX_POINT('',#43009);
#12488=VERTEX_POINT('',#43011);
#12489=VERTEX_POINT('',#43013);
#12490=VERTEX_POINT('',#43015);
#12491=VERTEX_POINT('',#43017);
#12492=VERTEX_POINT('',#43019);
#12493=VERTEX_POINT('',#43021);
#12494=VERTEX_POINT('',#43023);
#12495=VERTEX_POINT('',#43025);
#12496=VERTEX_POINT('',#43027);
#12497=VERTEX_POINT('',#43029);
#12498=VERTEX_POINT('',#43031);
#12499=VERTEX_POINT('',#43033);
#12500=VERTEX_POINT('',#43035);
#12501=VERTEX_POINT('',#43037);
#12502=VERTEX_POINT('',#43039);
#12503=VERTEX_POINT('',#43041);
#12504=VERTEX_POINT('',#43043);
#12505=VERTEX_POINT('',#43045);
#12506=VERTEX_POINT('',#43047);
#12507=VERTEX_POINT('',#43049);
#12508=VERTEX_POINT('',#43051);
#12509=VERTEX_POINT('',#43053);
#12510=VERTEX_POINT('',#43055);
#12511=VERTEX_POINT('',#43057);
#12512=VERTEX_POINT('',#43059);
#12513=VERTEX_POINT('',#43061);
#12514=VERTEX_POINT('',#43063);
#12515=VERTEX_POINT('',#43065);
#12516=VERTEX_POINT('',#43067);
#12517=VERTEX_POINT('',#43069);
#12518=VERTEX_POINT('',#43071);
#12519=VERTEX_POINT('',#43073);
#12520=VERTEX_POINT('',#43075);
#12521=VERTEX_POINT('',#43077);
#12522=VERTEX_POINT('',#43079);
#12523=VERTEX_POINT('',#43081);
#12524=VERTEX_POINT('',#43083);
#12525=VERTEX_POINT('',#43085);
#12526=VERTEX_POINT('',#43087);
#12527=VERTEX_POINT('',#43089);
#12528=VERTEX_POINT('',#43091);
#12529=VERTEX_POINT('',#43093);
#12530=VERTEX_POINT('',#43095);
#12531=VERTEX_POINT('',#43097);
#12532=VERTEX_POINT('',#43099);
#12533=VERTEX_POINT('',#43101);
#12534=VERTEX_POINT('',#43103);
#12535=VERTEX_POINT('',#43105);
#12536=VERTEX_POINT('',#43107);
#12537=VERTEX_POINT('',#43109);
#12538=VERTEX_POINT('',#43111);
#12539=VERTEX_POINT('',#43113);
#12540=VERTEX_POINT('',#43115);
#12541=VERTEX_POINT('',#43117);
#12542=VERTEX_POINT('',#43119);
#12543=VERTEX_POINT('',#43121);
#12544=VERTEX_POINT('',#43123);
#12545=VERTEX_POINT('',#43125);
#12546=VERTEX_POINT('',#43127);
#12547=VERTEX_POINT('',#43129);
#12548=VERTEX_POINT('',#43131);
#12549=VERTEX_POINT('',#43133);
#12550=VERTEX_POINT('',#43135);
#12551=VERTEX_POINT('',#43137);
#12552=VERTEX_POINT('',#43139);
#12553=VERTEX_POINT('',#43141);
#12554=VERTEX_POINT('',#43143);
#12555=VERTEX_POINT('',#43145);
#12556=VERTEX_POINT('',#43147);
#12557=VERTEX_POINT('',#43149);
#12558=VERTEX_POINT('',#43151);
#12559=VERTEX_POINT('',#43153);
#12560=VERTEX_POINT('',#43155);
#12561=VERTEX_POINT('',#43157);
#12562=VERTEX_POINT('',#43159);
#12563=VERTEX_POINT('',#43161);
#12564=VERTEX_POINT('',#43163);
#12565=VERTEX_POINT('',#43165);
#12566=VERTEX_POINT('',#43167);
#12567=VERTEX_POINT('',#43169);
#12568=VERTEX_POINT('',#43171);
#12569=VERTEX_POINT('',#43173);
#12570=VERTEX_POINT('',#43175);
#12571=VERTEX_POINT('',#43177);
#12572=VERTEX_POINT('',#43179);
#12573=VERTEX_POINT('',#43181);
#12574=VERTEX_POINT('',#43183);
#12575=VERTEX_POINT('',#43185);
#12576=VERTEX_POINT('',#43187);
#12577=VERTEX_POINT('',#43189);
#12578=VERTEX_POINT('',#43191);
#12579=VERTEX_POINT('',#43193);
#12580=VERTEX_POINT('',#43195);
#12581=VERTEX_POINT('',#43197);
#12582=VERTEX_POINT('',#43199);
#12583=VERTEX_POINT('',#43201);
#12584=VERTEX_POINT('',#43203);
#12585=VERTEX_POINT('',#43205);
#12586=VERTEX_POINT('',#43207);
#12587=VERTEX_POINT('',#43209);
#12588=VERTEX_POINT('',#43211);
#12589=VERTEX_POINT('',#43213);
#12590=VERTEX_POINT('',#43215);
#12591=VERTEX_POINT('',#43217);
#12592=VERTEX_POINT('',#43219);
#12593=VERTEX_POINT('',#43221);
#12594=VERTEX_POINT('',#43223);
#12595=VERTEX_POINT('',#43225);
#12596=VERTEX_POINT('',#43227);
#12597=VERTEX_POINT('',#43229);
#12598=VERTEX_POINT('',#43231);
#12599=VERTEX_POINT('',#43233);
#12600=VERTEX_POINT('',#43235);
#12601=VERTEX_POINT('',#43237);
#12602=VERTEX_POINT('',#43239);
#12603=VERTEX_POINT('',#43241);
#12604=VERTEX_POINT('',#43243);
#12605=VERTEX_POINT('',#43245);
#12606=VERTEX_POINT('',#43247);
#12607=VERTEX_POINT('',#43249);
#12608=VERTEX_POINT('',#43251);
#12609=VERTEX_POINT('',#43253);
#12610=VERTEX_POINT('',#43255);
#12611=VERTEX_POINT('',#43257);
#12612=VERTEX_POINT('',#43259);
#12613=VERTEX_POINT('',#43261);
#12614=VERTEX_POINT('',#43263);
#12615=VERTEX_POINT('',#43265);
#12616=VERTEX_POINT('',#43267);
#12617=VERTEX_POINT('',#43269);
#12618=VERTEX_POINT('',#43271);
#12619=VERTEX_POINT('',#43273);
#12620=VERTEX_POINT('',#43275);
#12621=VERTEX_POINT('',#43277);
#12622=VERTEX_POINT('',#43279);
#12623=VERTEX_POINT('',#43281);
#12624=VERTEX_POINT('',#43283);
#12625=VERTEX_POINT('',#43285);
#12626=VERTEX_POINT('',#43287);
#12627=VERTEX_POINT('',#43289);
#12628=VERTEX_POINT('',#43291);
#12629=VERTEX_POINT('',#43293);
#12630=VERTEX_POINT('',#43295);
#12631=VERTEX_POINT('',#43297);
#12632=VERTEX_POINT('',#43299);
#12633=VERTEX_POINT('',#43303);
#12634=VERTEX_POINT('',#43305);
#12635=VERTEX_POINT('',#43309);
#12636=VERTEX_POINT('',#43311);
#12637=VERTEX_POINT('',#43318);
#12638=VERTEX_POINT('',#43322);
#12639=VERTEX_POINT('',#43328);
#12640=VERTEX_POINT('',#43330);
#12641=VERTEX_POINT('',#43334);
#12642=VERTEX_POINT('',#43336);
#12643=VERTEX_POINT('',#43343);
#12644=VERTEX_POINT('',#43347);
#12645=VERTEX_POINT('',#43353);
#12646=VERTEX_POINT('',#43355);
#12647=VERTEX_POINT('',#43359);
#12648=VERTEX_POINT('',#43361);
#12649=VERTEX_POINT('',#43368);
#12650=VERTEX_POINT('',#43372);
#12651=VERTEX_POINT('',#43378);
#12652=VERTEX_POINT('',#43380);
#12653=VERTEX_POINT('',#43384);
#12654=VERTEX_POINT('',#43386);
#12655=VERTEX_POINT('',#43390);
#12656=VERTEX_POINT('',#43394);
#12657=VERTEX_POINT('',#43401);
#12658=VERTEX_POINT('',#43404);
#12659=VERTEX_POINT('',#43406);
#12660=VERTEX_POINT('',#43409);
#12661=VERTEX_POINT('',#43411);
#12662=VERTEX_POINT('',#43414);
#12663=VERTEX_POINT('',#43416);
#12664=VERTEX_POINT('',#43419);
#12665=VERTEX_POINT('',#43421);
#12666=VERTEX_POINT('',#43424);
#12667=VERTEX_POINT('',#43426);
#12668=VERTEX_POINT('',#43429);
#12669=VERTEX_POINT('',#43431);
#12670=VERTEX_POINT('',#43434);
#12671=VERTEX_POINT('',#43436);
#12672=VERTEX_POINT('',#43439);
#12673=VERTEX_POINT('',#43441);
#12674=VERTEX_POINT('',#43444);
#12675=VERTEX_POINT('',#43446);
#12676=VERTEX_POINT('',#43449);
#12677=VERTEX_POINT('',#43451);
#12678=VERTEX_POINT('',#43454);
#12679=VERTEX_POINT('',#43456);
#12680=VERTEX_POINT('',#43459);
#12681=VERTEX_POINT('',#43461);
#12682=VERTEX_POINT('',#43464);
#12683=VERTEX_POINT('',#43466);
#12684=VERTEX_POINT('',#43469);
#12685=VERTEX_POINT('',#43471);
#12686=VERTEX_POINT('',#43474);
#12687=VERTEX_POINT('',#43476);
#12688=VERTEX_POINT('',#43479);
#12689=VERTEX_POINT('',#43481);
#12690=VERTEX_POINT('',#43484);
#12691=VERTEX_POINT('',#43486);
#12692=VERTEX_POINT('',#43489);
#12693=VERTEX_POINT('',#43491);
#12694=VERTEX_POINT('',#43494);
#12695=VERTEX_POINT('',#43496);
#12696=VERTEX_POINT('',#43499);
#12697=VERTEX_POINT('',#43501);
#12698=VERTEX_POINT('',#43504);
#12699=VERTEX_POINT('',#43506);
#12700=VERTEX_POINT('',#43509);
#12701=VERTEX_POINT('',#43511);
#12702=VERTEX_POINT('',#43514);
#12703=VERTEX_POINT('',#43516);
#12704=VERTEX_POINT('',#43519);
#12705=VERTEX_POINT('',#43521);
#12706=VERTEX_POINT('',#43524);
#12707=VERTEX_POINT('',#43526);
#12708=VERTEX_POINT('',#43529);
#12709=VERTEX_POINT('',#43530);
#12710=VERTEX_POINT('',#43532);
#12711=VERTEX_POINT('',#43534);
#12712=VERTEX_POINT('',#43536);
#12713=VERTEX_POINT('',#43538);
#12714=VERTEX_POINT('',#43540);
#12715=VERTEX_POINT('',#43542);
#12716=VERTEX_POINT('',#43546);
#12717=VERTEX_POINT('',#43550);
#12718=VERTEX_POINT('',#43556);
#12719=VERTEX_POINT('',#43560);
#12720=VERTEX_POINT('',#43566);
#12721=VERTEX_POINT('',#43570);
#12722=VERTEX_POINT('',#43576);
#12723=VERTEX_POINT('',#43580);
#12724=VERTEX_POINT('',#43586);
#12725=VERTEX_POINT('',#43590);
#12726=VERTEX_POINT('',#43596);
#12727=VERTEX_POINT('',#43600);
#12728=VERTEX_POINT('',#43606);
#12729=VERTEX_POINT('',#43610);
#12730=VERTEX_POINT('',#43616);
#12731=VERTEX_POINT('',#43620);
#12732=VERTEX_POINT('',#43626);
#12733=VERTEX_POINT('',#43630);
#12734=VERTEX_POINT('',#43636);
#12735=VERTEX_POINT('',#43640);
#12736=VERTEX_POINT('',#43646);
#12737=VERTEX_POINT('',#43650);
#12738=VERTEX_POINT('',#43656);
#12739=VERTEX_POINT('',#43660);
#12740=VERTEX_POINT('',#43666);
#12741=VERTEX_POINT('',#43670);
#12742=VERTEX_POINT('',#43676);
#12743=VERTEX_POINT('',#43680);
#12744=VERTEX_POINT('',#43686);
#12745=VERTEX_POINT('',#43690);
#12746=VERTEX_POINT('',#43696);
#12747=VERTEX_POINT('',#43700);
#12748=VERTEX_POINT('',#43706);
#12749=VERTEX_POINT('',#43710);
#12750=VERTEX_POINT('',#43716);
#12751=VERTEX_POINT('',#43720);
#12752=VERTEX_POINT('',#43726);
#12753=VERTEX_POINT('',#43730);
#12754=VERTEX_POINT('',#43736);
#12755=VERTEX_POINT('',#43740);
#12756=VERTEX_POINT('',#43744);
#12757=VERTEX_POINT('',#43750);
#12758=VERTEX_POINT('',#43756);
#12759=VERTEX_POINT('',#43760);
#12760=VERTEX_POINT('',#43766);
#12761=VERTEX_POINT('',#43770);
#12762=VERTEX_POINT('',#43776);
#12763=VERTEX_POINT('',#43780);
#12764=VERTEX_POINT('',#43786);
#12765=VERTEX_POINT('',#43790);
#12766=VERTEX_POINT('',#43796);
#12767=VERTEX_POINT('',#43800);
#12768=VERTEX_POINT('',#43806);
#12769=VERTEX_POINT('',#43810);
#12770=VERTEX_POINT('',#43816);
#12771=VERTEX_POINT('',#43820);
#12772=VERTEX_POINT('',#43826);
#12773=VERTEX_POINT('',#43830);
#12774=VERTEX_POINT('',#43836);
#12775=VERTEX_POINT('',#43840);
#12776=VERTEX_POINT('',#43846);
#12777=VERTEX_POINT('',#43850);
#12778=VERTEX_POINT('',#43856);
#12779=VERTEX_POINT('',#43860);
#12780=VERTEX_POINT('',#43866);
#12781=VERTEX_POINT('',#43870);
#12782=VERTEX_POINT('',#43876);
#12783=VERTEX_POINT('',#43880);
#12784=VERTEX_POINT('',#43886);
#12785=VERTEX_POINT('',#43890);
#12786=VERTEX_POINT('',#43896);
#12787=VERTEX_POINT('',#43900);
#12788=VERTEX_POINT('',#43906);
#12789=VERTEX_POINT('',#43910);
#12790=VERTEX_POINT('',#43916);
#12791=VERTEX_POINT('',#43920);
#12792=VERTEX_POINT('',#43926);
#12793=VERTEX_POINT('',#43930);
#12794=VERTEX_POINT('',#43936);
#12795=VERTEX_POINT('',#43940);
#12796=VERTEX_POINT('',#43946);
#12797=VERTEX_POINT('',#43950);
#12798=VERTEX_POINT('',#43956);
#12799=VERTEX_POINT('',#43960);
#12800=VERTEX_POINT('',#43966);
#12801=VERTEX_POINT('',#43970);
#12802=VERTEX_POINT('',#43976);
#12803=VERTEX_POINT('',#43980);
#12804=VERTEX_POINT('',#43986);
#12805=VERTEX_POINT('',#43990);
#12806=VERTEX_POINT('',#43996);
#12807=VERTEX_POINT('',#43997);
#12808=VERTEX_POINT('',#43999);
#12809=VERTEX_POINT('',#44001);
#12810=VERTEX_POINT('',#44009);
#12811=VERTEX_POINT('',#44011);
#12812=VERTEX_POINT('',#44014);
#12813=VERTEX_POINT('',#44016);
#12814=VERTEX_POINT('',#44019);
#12815=VERTEX_POINT('',#44021);
#12816=VERTEX_POINT('',#44024);
#12817=VERTEX_POINT('',#44026);
#12818=VERTEX_POINT('',#44029);
#12819=VERTEX_POINT('',#44031);
#12820=VERTEX_POINT('',#44034);
#12821=VERTEX_POINT('',#44036);
#12822=VERTEX_POINT('',#44039);
#12823=VERTEX_POINT('',#44041);
#12824=VERTEX_POINT('',#44044);
#12825=VERTEX_POINT('',#44046);
#12826=VERTEX_POINT('',#44049);
#12827=VERTEX_POINT('',#44051);
#12828=VERTEX_POINT('',#44054);
#12829=VERTEX_POINT('',#44056);
#12830=VERTEX_POINT('',#44059);
#12831=VERTEX_POINT('',#44061);
#12832=VERTEX_POINT('',#44064);
#12833=VERTEX_POINT('',#44066);
#12834=VERTEX_POINT('',#44069);
#12835=VERTEX_POINT('',#44071);
#12836=VERTEX_POINT('',#44074);
#12837=VERTEX_POINT('',#44076);
#12838=VERTEX_POINT('',#44079);
#12839=VERTEX_POINT('',#44081);
#12840=VERTEX_POINT('',#44084);
#12841=VERTEX_POINT('',#44086);
#12842=VERTEX_POINT('',#44089);
#12843=VERTEX_POINT('',#44091);
#12844=VERTEX_POINT('',#44094);
#12845=VERTEX_POINT('',#44096);
#12846=VERTEX_POINT('',#44099);
#12847=VERTEX_POINT('',#44101);
#12848=VERTEX_POINT('',#44104);
#12849=VERTEX_POINT('',#44106);
#12850=VERTEX_POINT('',#44109);
#12851=VERTEX_POINT('',#44111);
#12852=VERTEX_POINT('',#44114);
#12853=VERTEX_POINT('',#44116);
#12854=VERTEX_POINT('',#44119);
#12855=VERTEX_POINT('',#44121);
#12856=VERTEX_POINT('',#44124);
#12857=VERTEX_POINT('',#44126);
#12858=VERTEX_POINT('',#44129);
#12859=VERTEX_POINT('',#44131);
#12860=VERTEX_POINT('',#44134);
#12861=VERTEX_POINT('',#44136);
#12862=VERTEX_POINT('',#44139);
#12863=VERTEX_POINT('',#44141);
#12864=VERTEX_POINT('',#44144);
#12865=VERTEX_POINT('',#44146);
#12866=VERTEX_POINT('',#44149);
#12867=VERTEX_POINT('',#44151);
#12868=VERTEX_POINT('',#44154);
#12869=VERTEX_POINT('',#44155);
#12870=VERTEX_POINT('',#44157);
#12871=VERTEX_POINT('',#44159);
#12872=VERTEX_POINT('',#44161);
#12873=VERTEX_POINT('',#44163);
#12874=VERTEX_POINT('',#44165);
#12875=VERTEX_POINT('',#44167);
#12876=VERTEX_POINT('',#44173);
#12877=VERTEX_POINT('',#44175);
#12878=VERTEX_POINT('',#44183);
#12879=VERTEX_POINT('',#44185);
#12880=VERTEX_POINT('',#44193);
#12881=VERTEX_POINT('',#44197);
#12882=VERTEX_POINT('',#44201);
#12883=VERTEX_POINT('',#44203);
#12884=VERTEX_POINT('',#44211);
#12885=VERTEX_POINT('',#44213);
#12886=VERTEX_POINT('',#44221);
#12887=VERTEX_POINT('',#44225);
#12888=VERTEX_POINT('',#44229);
#12889=VERTEX_POINT('',#44231);
#12890=VERTEX_POINT('',#44239);
#12891=VERTEX_POINT('',#44241);
#12892=VERTEX_POINT('',#44249);
#12893=VERTEX_POINT('',#44253);
#12894=VERTEX_POINT('',#44257);
#12895=VERTEX_POINT('',#44261);
#12896=VERTEX_POINT('',#44267);
#12897=VERTEX_POINT('',#44269);
#12898=VERTEX_POINT('',#44277);
#12899=VERTEX_POINT('',#44279);
#12900=VERTEX_POINT('',#44287);
#12901=VERTEX_POINT('',#44291);
#12902=VERTEX_POINT('',#44295);
#12903=VERTEX_POINT('',#44297);
#12904=VERTEX_POINT('',#44305);
#12905=VERTEX_POINT('',#44307);
#12906=VERTEX_POINT('',#44315);
#12907=VERTEX_POINT('',#44319);
#12908=VERTEX_POINT('',#44323);
#12909=VERTEX_POINT('',#44325);
#12910=VERTEX_POINT('',#44333);
#12911=VERTEX_POINT('',#44335);
#12912=VERTEX_POINT('',#44343);
#12913=VERTEX_POINT('',#44347);
#12914=VERTEX_POINT('',#44351);
#12915=VERTEX_POINT('',#44353);
#12916=VERTEX_POINT('',#44361);
#12917=VERTEX_POINT('',#44363);
#12918=VERTEX_POINT('',#44371);
#12919=VERTEX_POINT('',#44375);
#12920=VERTEX_POINT('',#44379);
#12921=VERTEX_POINT('',#44381);
#12922=VERTEX_POINT('',#44389);
#12923=VERTEX_POINT('',#44391);
#12924=VERTEX_POINT('',#44399);
#12925=VERTEX_POINT('',#44403);
#12926=VERTEX_POINT('',#44407);
#12927=VERTEX_POINT('',#44409);
#12928=VERTEX_POINT('',#44417);
#12929=VERTEX_POINT('',#44419);
#12930=VERTEX_POINT('',#44427);
#12931=VERTEX_POINT('',#44431);
#12932=VERTEX_POINT('',#44435);
#12933=VERTEX_POINT('',#44437);
#12934=VERTEX_POINT('',#44445);
#12935=VERTEX_POINT('',#44447);
#12936=VERTEX_POINT('',#44455);
#12937=VERTEX_POINT('',#44457);
#12938=VERTEX_POINT('',#44465);
#12939=VERTEX_POINT('',#44469);
#12940=VERTEX_POINT('',#44473);
#12941=VERTEX_POINT('',#44475);
#12942=VERTEX_POINT('',#44483);
#12943=VERTEX_POINT('',#44485);
#12944=VERTEX_POINT('',#44493);
#12945=VERTEX_POINT('',#44497);
#12946=VERTEX_POINT('',#44501);
#12947=VERTEX_POINT('',#44503);
#12948=VERTEX_POINT('',#44511);
#12949=VERTEX_POINT('',#44513);
#12950=VERTEX_POINT('',#44521);
#12951=VERTEX_POINT('',#44525);
#12952=VERTEX_POINT('',#44529);
#12953=VERTEX_POINT('',#44533);
#12954=VERTEX_POINT('',#44539);
#12955=VERTEX_POINT('',#44541);
#12956=VERTEX_POINT('',#44549);
#12957=VERTEX_POINT('',#44551);
#12958=VERTEX_POINT('',#44559);
#12959=VERTEX_POINT('',#44563);
#12960=VERTEX_POINT('',#44567);
#12961=VERTEX_POINT('',#44569);
#12962=VERTEX_POINT('',#44573);
#12963=VERTEX_POINT('',#44577);
#12964=VERTEX_POINT('',#44581);
#12965=VERTEX_POINT('',#44583);
#12966=VERTEX_POINT('',#44587);
#12967=VERTEX_POINT('',#44591);
#12968=VERTEX_POINT('',#44595);
#12969=VERTEX_POINT('',#44597);
#12970=VERTEX_POINT('',#44608);
#12971=VERTEX_POINT('',#44609);
#12972=VERTEX_POINT('',#44614);
#12973=VERTEX_POINT('',#44620);
#12974=VERTEX_POINT('',#44622);
#12975=VERTEX_POINT('',#44626);
#12976=VERTEX_POINT('',#44643);
#12977=VERTEX_POINT('',#44645);
#12978=VERTEX_POINT('',#44655);
#12979=VERTEX_POINT('',#44657);
#12980=VERTEX_POINT('',#44671);
#12981=VERTEX_POINT('',#44673);
#12982=VERTEX_POINT('',#44687);
#12983=VERTEX_POINT('',#44689);
#12984=VERTEX_POINT('',#44703);
#12985=VERTEX_POINT('',#44705);
#12986=VERTEX_POINT('',#44715);
#12987=VERTEX_POINT('',#44717);
#12988=VERTEX_POINT('',#44731);
#12989=VERTEX_POINT('',#44733);
#12990=VERTEX_POINT('',#44747);
#12991=VERTEX_POINT('',#44749);
#12992=VERTEX_POINT('',#44763);
#12993=VERTEX_POINT('',#44765);
#12994=VERTEX_POINT('',#44779);
#12995=VERTEX_POINT('',#44781);
#12996=VERTEX_POINT('',#44797);
#12997=VERTEX_POINT('',#44799);
#12998=VERTEX_POINT('',#44813);
#12999=VERTEX_POINT('',#44815);
#13000=VERTEX_POINT('',#44825);
#13001=VERTEX_POINT('',#44827);
#13002=VERTEX_POINT('',#44842);
#13003=VERTEX_POINT('',#44846);
#13004=VERTEX_POINT('',#44853);
#13005=VERTEX_POINT('',#44855);
#13006=VERTEX_POINT('',#44864);
#13007=VERTEX_POINT('',#44868);
#13008=VERTEX_POINT('',#44878);
#13009=VERTEX_POINT('',#44882);
#13010=VERTEX_POINT('',#44889);
#13011=VERTEX_POINT('',#44891);
#13012=VERTEX_POINT('',#44900);
#13013=VERTEX_POINT('',#44904);
#13014=VERTEX_POINT('',#44914);
#13015=VERTEX_POINT('',#44918);
#13016=VERTEX_POINT('',#44925);
#13017=VERTEX_POINT('',#44927);
#13018=VERTEX_POINT('',#44936);
#13019=VERTEX_POINT('',#44940);
#13020=VERTEX_POINT('',#44947);
#13021=VERTEX_POINT('',#44949);
#15201=EDGE_CURVE('',#12268,#12269,#202,.T.);
#15202=EDGE_CURVE('',#12269,#12270,#2353,.T.);
#15203=EDGE_CURVE('',#12270,#12271,#2354,.F.);
#15204=EDGE_CURVE('',#12271,#12268,#2355,.T.);
#15205=EDGE_CURVE('',#12272,#12269,#2356,.T.);
#15206=EDGE_CURVE('',#12272,#12273,#2357,.T.);
#15207=EDGE_CURVE('',#12270,#12273,#2358,.T.);
#15208=EDGE_CURVE('',#12274,#12268,#10596,.T.);
#15209=EDGE_CURVE('',#12275,#12274,#203,.T.);
#15210=EDGE_CURVE('',#12275,#12276,#2359,.T.);
#15211=EDGE_CURVE('',#12276,#12277,#10597,.T.);
#15212=EDGE_CURVE('',#12277,#12278,#2360,.T.);
#15213=EDGE_CURVE('',#12279,#12278,#204,.T.);
#15214=EDGE_CURVE('',#12280,#12279,#10598,.T.);
#15215=EDGE_CURVE('',#12281,#12280,#205,.T.);
#15216=EDGE_CURVE('',#12281,#12282,#2361,.T.);
#15217=EDGE_CURVE('',#12282,#12283,#10599,.T.);
#15218=EDGE_CURVE('',#12283,#12284,#2362,.T.);
#15219=EDGE_CURVE('',#12285,#12284,#206,.T.);
#15220=EDGE_CURVE('',#12286,#12285,#10600,.T.);
#15221=EDGE_CURVE('',#12286,#12287,#2363,.T.);
#15222=EDGE_CURVE('',#12287,#12288,#10601,.T.);
#15223=EDGE_CURVE('',#12289,#12288,#207,.T.);
#15224=EDGE_CURVE('',#12289,#12290,#2364,.T.);
#15225=EDGE_CURVE('',#12290,#12291,#10602,.T.);
#15226=EDGE_CURVE('',#12291,#12292,#2365,.T.);
#15227=EDGE_CURVE('',#12293,#12292,#208,.T.);
#15228=EDGE_CURVE('',#12293,#12294,#10603,.T.);
#15229=EDGE_CURVE('',#12295,#12294,#209,.T.);
#15230=EDGE_CURVE('',#12295,#12296,#2366,.T.);
#15231=EDGE_CURVE('',#12296,#12297,#10604,.T.);
#15232=EDGE_CURVE('',#12297,#12298,#2367,.T.);
#15233=EDGE_CURVE('',#12299,#12298,#210,.T.);
#15234=EDGE_CURVE('',#12299,#12300,#10605,.T.);
#15235=EDGE_CURVE('',#12301,#12300,#211,.T.);
#15236=EDGE_CURVE('',#12301,#12302,#2368,.T.);
#15237=EDGE_CURVE('',#12302,#12303,#10606,.T.);
#15238=EDGE_CURVE('',#12303,#12304,#2369,.T.);
#15239=EDGE_CURVE('',#12305,#12304,#212,.T.);
#15240=EDGE_CURVE('',#12305,#12306,#10607,.T.);
#15241=EDGE_CURVE('',#12307,#12306,#213,.T.);
#15242=EDGE_CURVE('',#12307,#12308,#2370,.T.);
#15243=EDGE_CURVE('',#12308,#12309,#10608,.T.);
#15244=EDGE_CURVE('',#12309,#12310,#2371,.T.);
#15245=EDGE_CURVE('',#12311,#12310,#214,.T.);
#15246=EDGE_CURVE('',#12311,#12312,#10609,.T.);
#15247=EDGE_CURVE('',#12313,#12312,#215,.T.);
#15248=EDGE_CURVE('',#12313,#12314,#2372,.T.);
#15249=EDGE_CURVE('',#12314,#12315,#10610,.T.);
#15250=EDGE_CURVE('',#12315,#12316,#2373,.T.);
#15251=EDGE_CURVE('',#12317,#12316,#216,.T.);
#15252=EDGE_CURVE('',#12317,#12318,#10611,.T.);
#15253=EDGE_CURVE('',#12319,#12318,#217,.T.);
#15254=EDGE_CURVE('',#12319,#12320,#2374,.T.);
#15255=EDGE_CURVE('',#12320,#12321,#10612,.T.);
#15256=EDGE_CURVE('',#12321,#12322,#2375,.T.);
#15257=EDGE_CURVE('',#12323,#12322,#218,.T.);
#15258=EDGE_CURVE('',#12323,#12324,#10613,.T.);
#15259=EDGE_CURVE('',#12325,#12324,#219,.T.);
#15260=EDGE_CURVE('',#12325,#12326,#2376,.T.);
#15261=EDGE_CURVE('',#12326,#12327,#10614,.T.);
#15262=EDGE_CURVE('',#12327,#12328,#2377,.T.);
#15263=EDGE_CURVE('',#12329,#12328,#220,.T.);
#15264=EDGE_CURVE('',#12329,#12330,#10615,.T.);
#15265=EDGE_CURVE('',#12331,#12330,#221,.T.);
#15266=EDGE_CURVE('',#12331,#12332,#2378,.T.);
#15267=EDGE_CURVE('',#12332,#12333,#10616,.T.);
#15268=EDGE_CURVE('',#12333,#12334,#2379,.T.);
#15269=EDGE_CURVE('',#12335,#12334,#222,.T.);
#15270=EDGE_CURVE('',#12335,#12336,#10617,.T.);
#15271=EDGE_CURVE('',#12337,#12336,#223,.T.);
#15272=EDGE_CURVE('',#12337,#12338,#2380,.T.);
#15273=EDGE_CURVE('',#12338,#12339,#10618,.T.);
#15274=EDGE_CURVE('',#12339,#12340,#2381,.T.);
#15275=EDGE_CURVE('',#12341,#12340,#224,.T.);
#15276=EDGE_CURVE('',#12341,#12342,#10619,.T.);
#15277=EDGE_CURVE('',#12343,#12342,#225,.T.);
#15278=EDGE_CURVE('',#12343,#12344,#2382,.T.);
#15279=EDGE_CURVE('',#12344,#12345,#10620,.T.);
#15280=EDGE_CURVE('',#12345,#12346,#2383,.T.);
#15281=EDGE_CURVE('',#12347,#12346,#226,.T.);
#15282=EDGE_CURVE('',#12347,#12348,#10621,.T.);
#15283=EDGE_CURVE('',#12349,#12348,#227,.T.);
#15284=EDGE_CURVE('',#12349,#12350,#2384,.T.);
#15285=EDGE_CURVE('',#12350,#12351,#10622,.T.);
#15286=EDGE_CURVE('',#12351,#12352,#2385,.T.);
#15287=EDGE_CURVE('',#12353,#12352,#228,.T.);
#15288=EDGE_CURVE('',#12353,#12354,#10623,.T.);
#15289=EDGE_CURVE('',#12355,#12354,#229,.T.);
#15290=EDGE_CURVE('',#12355,#12356,#2386,.T.);
#15291=EDGE_CURVE('',#12356,#12357,#10624,.T.);
#15292=EDGE_CURVE('',#12357,#12358,#2387,.T.);
#15293=EDGE_CURVE('',#12359,#12358,#230,.T.);
#15294=EDGE_CURVE('',#12359,#12360,#10625,.T.);
#15295=EDGE_CURVE('',#12361,#12360,#231,.T.);
#15296=EDGE_CURVE('',#12361,#12362,#2388,.T.);
#15297=EDGE_CURVE('',#12362,#12363,#10626,.T.);
#15298=EDGE_CURVE('',#12363,#12364,#2389,.T.);
#15299=EDGE_CURVE('',#12365,#12364,#232,.T.);
#15300=EDGE_CURVE('',#12365,#12366,#10627,.T.);
#15301=EDGE_CURVE('',#12367,#12366,#233,.T.);
#15302=EDGE_CURVE('',#12367,#12368,#2390,.T.);
#15303=EDGE_CURVE('',#12368,#12369,#10628,.T.);
#15304=EDGE_CURVE('',#12369,#12370,#2391,.T.);
#15305=EDGE_CURVE('',#12371,#12370,#234,.T.);
#15306=EDGE_CURVE('',#12371,#12372,#10629,.T.);
#15307=EDGE_CURVE('',#12373,#12372,#235,.T.);
#15308=EDGE_CURVE('',#12373,#12374,#2392,.T.);
#15309=EDGE_CURVE('',#12374,#12375,#10630,.T.);
#15310=EDGE_CURVE('',#12375,#12376,#2393,.T.);
#15311=EDGE_CURVE('',#12377,#12376,#236,.T.);
#15312=EDGE_CURVE('',#12377,#12378,#10631,.T.);
#15313=EDGE_CURVE('',#12379,#12378,#237,.T.);
#15314=EDGE_CURVE('',#12379,#12380,#2394,.T.);
#15315=EDGE_CURVE('',#12380,#12381,#10632,.T.);
#15316=EDGE_CURVE('',#12381,#12382,#2395,.T.);
#15317=EDGE_CURVE('',#12383,#12382,#238,.T.);
#15318=EDGE_CURVE('',#12383,#12384,#10633,.T.);
#15319=EDGE_CURVE('',#12385,#12384,#239,.T.);
#15320=EDGE_CURVE('',#12385,#12386,#2396,.T.);
#15321=EDGE_CURVE('',#12386,#12387,#10634,.T.);
#15322=EDGE_CURVE('',#12387,#12388,#2397,.T.);
#15323=EDGE_CURVE('',#12389,#12388,#240,.T.);
#15324=EDGE_CURVE('',#12389,#12390,#10635,.T.);
#15325=EDGE_CURVE('',#12391,#12390,#241,.T.);
#15326=EDGE_CURVE('',#12391,#12392,#2398,.T.);
#15327=EDGE_CURVE('',#12392,#12393,#10636,.T.);
#15328=EDGE_CURVE('',#12393,#12394,#2399,.T.);
#15329=EDGE_CURVE('',#12395,#12394,#242,.T.);
#15330=EDGE_CURVE('',#12395,#12396,#10637,.T.);
#15331=EDGE_CURVE('',#12397,#12396,#243,.T.);
#15332=EDGE_CURVE('',#12397,#12398,#2400,.T.);
#15333=EDGE_CURVE('',#12398,#12399,#10638,.T.);
#15334=EDGE_CURVE('',#12399,#12400,#2401,.T.);
#15335=EDGE_CURVE('',#12401,#12400,#244,.T.);
#15336=EDGE_CURVE('',#12401,#12402,#10639,.T.);
#15337=EDGE_CURVE('',#12403,#12402,#245,.T.);
#15338=EDGE_CURVE('',#12403,#12404,#2402,.T.);
#15339=EDGE_CURVE('',#12404,#12405,#10640,.T.);
#15340=EDGE_CURVE('',#12405,#12406,#2403,.T.);
#15341=EDGE_CURVE('',#12407,#12406,#246,.T.);
#15342=EDGE_CURVE('',#12407,#12408,#10641,.T.);
#15343=EDGE_CURVE('',#12409,#12408,#247,.T.);
#15344=EDGE_CURVE('',#12409,#12410,#2404,.T.);
#15345=EDGE_CURVE('',#12410,#12411,#10642,.T.);
#15346=EDGE_CURVE('',#12411,#12412,#2405,.T.);
#15347=EDGE_CURVE('',#12413,#12412,#248,.T.);
#15348=EDGE_CURVE('',#12413,#12414,#10643,.T.);
#15349=EDGE_CURVE('',#12415,#12414,#249,.T.);
#15350=EDGE_CURVE('',#12415,#12416,#2406,.T.);
#15351=EDGE_CURVE('',#12416,#12417,#10644,.T.);
#15352=EDGE_CURVE('',#12417,#12418,#2407,.T.);
#15353=EDGE_CURVE('',#12419,#12418,#250,.T.);
#15354=EDGE_CURVE('',#12419,#12420,#10645,.T.);
#15355=EDGE_CURVE('',#12421,#12420,#251,.T.);
#15356=EDGE_CURVE('',#12421,#12422,#2408,.T.);
#15357=EDGE_CURVE('',#12422,#12423,#10646,.T.);
#15358=EDGE_CURVE('',#12423,#12424,#2409,.T.);
#15359=EDGE_CURVE('',#12425,#12424,#252,.T.);
#15360=EDGE_CURVE('',#12425,#12426,#10647,.T.);
#15361=EDGE_CURVE('',#12427,#12426,#253,.T.);
#15362=EDGE_CURVE('',#12427,#12428,#2410,.T.);
#15363=EDGE_CURVE('',#12428,#12429,#10648,.T.);
#15364=EDGE_CURVE('',#12429,#12430,#2411,.T.);
#15365=EDGE_CURVE('',#12431,#12430,#254,.T.);
#15366=EDGE_CURVE('',#12431,#12432,#10649,.T.);
#15367=EDGE_CURVE('',#12433,#12432,#255,.T.);
#15368=EDGE_CURVE('',#12433,#12434,#2412,.T.);
#15369=EDGE_CURVE('',#12434,#12435,#10650,.T.);
#15370=EDGE_CURVE('',#12435,#12436,#2413,.T.);
#15371=EDGE_CURVE('',#12437,#12436,#256,.T.);
#15372=EDGE_CURVE('',#12437,#12438,#10651,.T.);
#15373=EDGE_CURVE('',#12439,#12438,#257,.T.);
#15374=EDGE_CURVE('',#12439,#12440,#2414,.T.);
#15375=EDGE_CURVE('',#12440,#12441,#10652,.T.);
#15376=EDGE_CURVE('',#12441,#12442,#2415,.T.);
#15377=EDGE_CURVE('',#12443,#12442,#258,.T.);
#15378=EDGE_CURVE('',#12443,#12444,#10653,.T.);
#15379=EDGE_CURVE('',#12445,#12444,#259,.T.);
#15380=EDGE_CURVE('',#12445,#12446,#2416,.T.);
#15381=EDGE_CURVE('',#12446,#12447,#10654,.T.);
#15382=EDGE_CURVE('',#12447,#12448,#2417,.T.);
#15383=EDGE_CURVE('',#12449,#12448,#260,.T.);
#15384=EDGE_CURVE('',#12449,#12450,#10655,.T.);
#15385=EDGE_CURVE('',#12451,#12450,#261,.T.);
#15386=EDGE_CURVE('',#12451,#12452,#2418,.T.);
#15387=EDGE_CURVE('',#12452,#12453,#10656,.T.);
#15388=EDGE_CURVE('',#12453,#12454,#2419,.T.);
#15389=EDGE_CURVE('',#12455,#12454,#262,.T.);
#15390=EDGE_CURVE('',#12455,#12456,#10657,.T.);
#15391=EDGE_CURVE('',#12457,#12456,#263,.T.);
#15392=EDGE_CURVE('',#12457,#12458,#2420,.T.);
#15393=EDGE_CURVE('',#12458,#12459,#10658,.T.);
#15394=EDGE_CURVE('',#12459,#12460,#2421,.T.);
#15395=EDGE_CURVE('',#12461,#12460,#264,.T.);
#15396=EDGE_CURVE('',#12461,#12462,#10659,.T.);
#15397=EDGE_CURVE('',#12463,#12462,#265,.T.);
#15398=EDGE_CURVE('',#12463,#12464,#2422,.T.);
#15399=EDGE_CURVE('',#12464,#12465,#10660,.T.);
#15400=EDGE_CURVE('',#12465,#12466,#2423,.T.);
#15401=EDGE_CURVE('',#12467,#12466,#266,.T.);
#15402=EDGE_CURVE('',#12467,#12287,#10661,.T.);
#15403=EDGE_CURVE('',#12468,#12286,#10662,.T.);
#15404=EDGE_CURVE('',#12469,#12468,#267,.T.);
#15405=EDGE_CURVE('',#12469,#12470,#2424,.T.);
#15406=EDGE_CURVE('',#12470,#12471,#10663,.T.);
#15407=EDGE_CURVE('',#12471,#12472,#2425,.T.);
#15408=EDGE_CURVE('',#12473,#12472,#268,.T.);
#15409=EDGE_CURVE('',#12474,#12473,#10664,.T.);
#15410=EDGE_CURVE('',#12475,#12474,#269,.T.);
#15411=EDGE_CURVE('',#12475,#12476,#2426,.T.);
#15412=EDGE_CURVE('',#12476,#12477,#10665,.T.);
#15413=EDGE_CURVE('',#12477,#12478,#2427,.T.);
#15414=EDGE_CURVE('',#12479,#12478,#270,.T.);
#15415=EDGE_CURVE('',#12480,#12479,#10666,.T.);
#15416=EDGE_CURVE('',#12481,#12480,#271,.T.);
#15417=EDGE_CURVE('',#12481,#12482,#2428,.T.);
#15418=EDGE_CURVE('',#12482,#12483,#10667,.T.);
#15419=EDGE_CURVE('',#12483,#12484,#2429,.T.);
#15420=EDGE_CURVE('',#12485,#12484,#272,.T.);
#15421=EDGE_CURVE('',#12486,#12485,#10668,.T.);
#15422=EDGE_CURVE('',#12487,#12486,#273,.T.);
#15423=EDGE_CURVE('',#12487,#12488,#2430,.T.);
#15424=EDGE_CURVE('',#12488,#12489,#10669,.T.);
#15425=EDGE_CURVE('',#12489,#12490,#2431,.T.);
#15426=EDGE_CURVE('',#12491,#12490,#274,.T.);
#15427=EDGE_CURVE('',#12492,#12491,#10670,.T.);
#15428=EDGE_CURVE('',#12493,#12492,#275,.T.);
#15429=EDGE_CURVE('',#12493,#12494,#2432,.T.);
#15430=EDGE_CURVE('',#12494,#12495,#10671,.T.);
#15431=EDGE_CURVE('',#12495,#12496,#2433,.T.);
#15432=EDGE_CURVE('',#12497,#12496,#276,.T.);
#15433=EDGE_CURVE('',#12498,#12497,#10672,.T.);
#15434=EDGE_CURVE('',#12499,#12498,#277,.T.);
#15435=EDGE_CURVE('',#12499,#12500,#2434,.T.);
#15436=EDGE_CURVE('',#12500,#12501,#10673,.T.);
#15437=EDGE_CURVE('',#12501,#12502,#2435,.T.);
#15438=EDGE_CURVE('',#12503,#12502,#278,.T.);
#15439=EDGE_CURVE('',#12504,#12503,#10674,.T.);
#15440=EDGE_CURVE('',#12505,#12504,#279,.T.);
#15441=EDGE_CURVE('',#12505,#12506,#2436,.T.);
#15442=EDGE_CURVE('',#12506,#12507,#10675,.T.);
#15443=EDGE_CURVE('',#12507,#12508,#2437,.T.);
#15444=EDGE_CURVE('',#12509,#12508,#280,.T.);
#15445=EDGE_CURVE('',#12510,#12509,#10676,.T.);
#15446=EDGE_CURVE('',#12511,#12510,#281,.T.);
#15447=EDGE_CURVE('',#12511,#12512,#2438,.T.);
#15448=EDGE_CURVE('',#12512,#12513,#10677,.T.);
#15449=EDGE_CURVE('',#12513,#12514,#2439,.T.);
#15450=EDGE_CURVE('',#12515,#12514,#282,.T.);
#15451=EDGE_CURVE('',#12516,#12515,#10678,.T.);
#15452=EDGE_CURVE('',#12517,#12516,#283,.T.);
#15453=EDGE_CURVE('',#12517,#12518,#2440,.T.);
#15454=EDGE_CURVE('',#12518,#12519,#10679,.T.);
#15455=EDGE_CURVE('',#12519,#12520,#2441,.T.);
#15456=EDGE_CURVE('',#12521,#12520,#284,.T.);
#15457=EDGE_CURVE('',#12522,#12521,#10680,.T.);
#15458=EDGE_CURVE('',#12523,#12522,#285,.T.);
#15459=EDGE_CURVE('',#12523,#12524,#2442,.T.);
#15460=EDGE_CURVE('',#12524,#12525,#10681,.T.);
#15461=EDGE_CURVE('',#12525,#12526,#2443,.T.);
#15462=EDGE_CURVE('',#12527,#12526,#286,.T.);
#15463=EDGE_CURVE('',#12528,#12527,#10682,.T.);
#15464=EDGE_CURVE('',#12529,#12528,#287,.T.);
#15465=EDGE_CURVE('',#12529,#12530,#2444,.T.);
#15466=EDGE_CURVE('',#12530,#12531,#10683,.T.);
#15467=EDGE_CURVE('',#12531,#12532,#2445,.T.);
#15468=EDGE_CURVE('',#12533,#12532,#288,.T.);
#15469=EDGE_CURVE('',#12534,#12533,#10684,.T.);
#15470=EDGE_CURVE('',#12535,#12534,#289,.T.);
#15471=EDGE_CURVE('',#12535,#12536,#2446,.T.);
#15472=EDGE_CURVE('',#12536,#12537,#10685,.T.);
#15473=EDGE_CURVE('',#12537,#12538,#2447,.T.);
#15474=EDGE_CURVE('',#12539,#12538,#290,.T.);
#15475=EDGE_CURVE('',#12540,#12539,#10686,.T.);
#15476=EDGE_CURVE('',#12541,#12540,#291,.T.);
#15477=EDGE_CURVE('',#12541,#12542,#2448,.T.);
#15478=EDGE_CURVE('',#12542,#12543,#10687,.T.);
#15479=EDGE_CURVE('',#12543,#12544,#2449,.T.);
#15480=EDGE_CURVE('',#12545,#12544,#292,.T.);
#15481=EDGE_CURVE('',#12546,#12545,#10688,.T.);
#15482=EDGE_CURVE('',#12547,#12546,#293,.T.);
#15483=EDGE_CURVE('',#12547,#12548,#2450,.T.);
#15484=EDGE_CURVE('',#12548,#12549,#10689,.T.);
#15485=EDGE_CURVE('',#12549,#12550,#2451,.T.);
#15486=EDGE_CURVE('',#12551,#12550,#294,.T.);
#15487=EDGE_CURVE('',#12552,#12551,#10690,.T.);
#15488=EDGE_CURVE('',#12553,#12552,#295,.T.);
#15489=EDGE_CURVE('',#12553,#12554,#2452,.T.);
#15490=EDGE_CURVE('',#12554,#12555,#10691,.T.);
#15491=EDGE_CURVE('',#12555,#12556,#2453,.T.);
#15492=EDGE_CURVE('',#12557,#12556,#296,.T.);
#15493=EDGE_CURVE('',#12558,#12557,#10692,.T.);
#15494=EDGE_CURVE('',#12559,#12558,#297,.T.);
#15495=EDGE_CURVE('',#12559,#12560,#2454,.T.);
#15496=EDGE_CURVE('',#12560,#12561,#10693,.T.);
#15497=EDGE_CURVE('',#12561,#12562,#2455,.T.);
#15498=EDGE_CURVE('',#12563,#12562,#298,.T.);
#15499=EDGE_CURVE('',#12564,#12563,#10694,.T.);
#15500=EDGE_CURVE('',#12565,#12564,#299,.T.);
#15501=EDGE_CURVE('',#12565,#12566,#2456,.T.);
#15502=EDGE_CURVE('',#12566,#12567,#10695,.T.);
#15503=EDGE_CURVE('',#12567,#12568,#2457,.T.);
#15504=EDGE_CURVE('',#12569,#12568,#300,.T.);
#15505=EDGE_CURVE('',#12570,#12569,#10696,.T.);
#15506=EDGE_CURVE('',#12571,#12570,#301,.T.);
#15507=EDGE_CURVE('',#12571,#12572,#2458,.T.);
#15508=EDGE_CURVE('',#12572,#12573,#10697,.T.);
#15509=EDGE_CURVE('',#12573,#12574,#2459,.T.);
#15510=EDGE_CURVE('',#12575,#12574,#302,.T.);
#15511=EDGE_CURVE('',#12576,#12575,#10698,.T.);
#15512=EDGE_CURVE('',#12577,#12576,#303,.T.);
#15513=EDGE_CURVE('',#12577,#12578,#2460,.T.);
#15514=EDGE_CURVE('',#12578,#12579,#10699,.T.);
#15515=EDGE_CURVE('',#12579,#12580,#2461,.T.);
#15516=EDGE_CURVE('',#12581,#12580,#304,.T.);
#15517=EDGE_CURVE('',#12582,#12581,#10700,.T.);
#15518=EDGE_CURVE('',#12583,#12582,#305,.T.);
#15519=EDGE_CURVE('',#12583,#12584,#2462,.T.);
#15520=EDGE_CURVE('',#12584,#12585,#10701,.T.);
#15521=EDGE_CURVE('',#12585,#12586,#2463,.T.);
#15522=EDGE_CURVE('',#12587,#12586,#306,.T.);
#15523=EDGE_CURVE('',#12588,#12587,#10702,.T.);
#15524=EDGE_CURVE('',#12589,#12588,#307,.T.);
#15525=EDGE_CURVE('',#12589,#12590,#2464,.T.);
#15526=EDGE_CURVE('',#12590,#12591,#10703,.T.);
#15527=EDGE_CURVE('',#12591,#12592,#2465,.T.);
#15528=EDGE_CURVE('',#12593,#12592,#308,.T.);
#15529=EDGE_CURVE('',#12594,#12593,#10704,.T.);
#15530=EDGE_CURVE('',#12595,#12594,#309,.T.);
#15531=EDGE_CURVE('',#12595,#12596,#2466,.T.);
#15532=EDGE_CURVE('',#12596,#12597,#10705,.T.);
#15533=EDGE_CURVE('',#12597,#12598,#2467,.T.);
#15534=EDGE_CURVE('',#12599,#12598,#310,.T.);
#15535=EDGE_CURVE('',#12600,#12599,#10706,.T.);
#15536=EDGE_CURVE('',#12601,#12600,#311,.T.);
#15537=EDGE_CURVE('',#12601,#12602,#2468,.T.);
#15538=EDGE_CURVE('',#12602,#12603,#10707,.T.);
#15539=EDGE_CURVE('',#12603,#12604,#2469,.T.);
#15540=EDGE_CURVE('',#12605,#12604,#312,.T.);
#15541=EDGE_CURVE('',#12606,#12605,#10708,.T.);
#15542=EDGE_CURVE('',#12607,#12606,#313,.T.);
#15543=EDGE_CURVE('',#12607,#12608,#2470,.T.);
#15544=EDGE_CURVE('',#12608,#12609,#10709,.T.);
#15545=EDGE_CURVE('',#12609,#12610,#2471,.T.);
#15546=EDGE_CURVE('',#12611,#12610,#314,.T.);
#15547=EDGE_CURVE('',#12612,#12611,#10710,.T.);
#15548=EDGE_CURVE('',#12613,#12612,#315,.T.);
#15549=EDGE_CURVE('',#12613,#12614,#2472,.T.);
#15550=EDGE_CURVE('',#12614,#12615,#10711,.T.);
#15551=EDGE_CURVE('',#12615,#12616,#2473,.T.);
#15552=EDGE_CURVE('',#12617,#12616,#316,.T.);
#15553=EDGE_CURVE('',#12618,#12617,#10712,.T.);
#15554=EDGE_CURVE('',#12619,#12618,#317,.T.);
#15555=EDGE_CURVE('',#12619,#12620,#2474,.T.);
#15556=EDGE_CURVE('',#12620,#12621,#10713,.T.);
#15557=EDGE_CURVE('',#12621,#12622,#2475,.T.);
#15558=EDGE_CURVE('',#12623,#12622,#318,.T.);
#15559=EDGE_CURVE('',#12624,#12623,#10714,.T.);
#15560=EDGE_CURVE('',#12625,#12624,#319,.T.);
#15561=EDGE_CURVE('',#12625,#12626,#2476,.T.);
#15562=EDGE_CURVE('',#12626,#12627,#10715,.T.);
#15563=EDGE_CURVE('',#12627,#12628,#2477,.T.);
#15564=EDGE_CURVE('',#12629,#12628,#320,.T.);
#15565=EDGE_CURVE('',#12630,#12629,#10716,.T.);
#15566=EDGE_CURVE('',#12631,#12630,#321,.T.);
#15567=EDGE_CURVE('',#12631,#12632,#2478,.T.);
#15568=EDGE_CURVE('',#12632,#12272,#10717,.T.);
#15569=EDGE_CURVE('',#12633,#12275,#2479,.T.);
#15570=EDGE_CURVE('',#12274,#12634,#2480,.T.);
#15571=EDGE_CURVE('',#12634,#12633,#2481,.T.);
#15572=EDGE_CURVE('',#12634,#12635,#2482,.T.);
#15573=EDGE_CURVE('',#12635,#12636,#2483,.T.);
#15574=EDGE_CURVE('',#12636,#12633,#2484,.T.);
#15575=EDGE_CURVE('',#12635,#12279,#2485,.T.);
#15576=EDGE_CURVE('',#12278,#12636,#2486,.T.);
#15577=EDGE_CURVE('',#12633,#12637,#2487,.T.);
#15578=EDGE_CURVE('',#12637,#12276,#2488,.T.);
#15579=EDGE_CURVE('',#12636,#12638,#2489,.T.);
#15580=EDGE_CURVE('',#12638,#12637,#2490,.T.);
#15581=EDGE_CURVE('',#12277,#12638,#2491,.T.);
#15582=EDGE_CURVE('',#12639,#12281,#2492,.T.);
#15583=EDGE_CURVE('',#12280,#12640,#2493,.T.);
#15584=EDGE_CURVE('',#12640,#12639,#2494,.T.);
#15585=EDGE_CURVE('',#12640,#12641,#2495,.T.);
#15586=EDGE_CURVE('',#12641,#12642,#2496,.T.);
#15587=EDGE_CURVE('',#12642,#12639,#2497,.T.);
#15588=EDGE_CURVE('',#12641,#12285,#2498,.T.);
#15589=EDGE_CURVE('',#12284,#12642,#2499,.T.);
#15590=EDGE_CURVE('',#12639,#12643,#2500,.T.);
#15591=EDGE_CURVE('',#12643,#12282,#2501,.T.);
#15592=EDGE_CURVE('',#12642,#12644,#2502,.T.);
#15593=EDGE_CURVE('',#12644,#12643,#2503,.T.);
#15594=EDGE_CURVE('',#12283,#12644,#2504,.T.);
#15595=EDGE_CURVE('',#12645,#12469,#2505,.T.);
#15596=EDGE_CURVE('',#12468,#12646,#2506,.T.);
#15597=EDGE_CURVE('',#12646,#12645,#2507,.T.);
#15598=EDGE_CURVE('',#12646,#12647,#2508,.T.);
#15599=EDGE_CURVE('',#12647,#12648,#2509,.T.);
#15600=EDGE_CURVE('',#12648,#12645,#2510,.T.);
#15601=EDGE_CURVE('',#12647,#12473,#2511,.T.);
#15602=EDGE_CURVE('',#12472,#12648,#2512,.T.);
#15603=EDGE_CURVE('',#12645,#12649,#2513,.T.);
#15604=EDGE_CURVE('',#12649,#12470,#2514,.T.);
#15605=EDGE_CURVE('',#12648,#12650,#2515,.T.);
#15606=EDGE_CURVE('',#12650,#12649,#2516,.T.);
#15607=EDGE_CURVE('',#12471,#12650,#2517,.T.);
#15608=EDGE_CURVE('',#12651,#12475,#2518,.T.);
#15609=EDGE_CURVE('',#12474,#12652,#2519,.T.);
#15610=EDGE_CURVE('',#12652,#12651,#2520,.T.);
#15611=EDGE_CURVE('',#12652,#12653,#2521,.T.);
#15612=EDGE_CURVE('',#12653,#12654,#2522,.F.);
#15613=EDGE_CURVE('',#12654,#12651,#2523,.T.);
#15614=EDGE_CURVE('',#12651,#12655,#2524,.T.);
#15615=EDGE_CURVE('',#12655,#12476,#2525,.T.);
#15616=EDGE_CURVE('',#12654,#12656,#2526,.T.);
#15617=EDGE_CURVE('',#12656,#12655,#2527,.T.);
#15618=EDGE_CURVE('',#12478,#12654,#2528,.T.);
#15619=EDGE_CURVE('',#12653,#12479,#2529,.T.);
#15620=EDGE_CURVE('',#12657,#12271,#2530,.T.);
#15621=EDGE_CURVE('',#12630,#12657,#2531,.T.);
#15622=EDGE_CURVE('',#12658,#12629,#2532,.T.);
#15623=EDGE_CURVE('',#12659,#12658,#2533,.T.);
#15624=EDGE_CURVE('',#12624,#12659,#2534,.T.);
#15625=EDGE_CURVE('',#12660,#12623,#2535,.T.);
#15626=EDGE_CURVE('',#12661,#12660,#2536,.T.);
#15627=EDGE_CURVE('',#12618,#12661,#2537,.T.);
#15628=EDGE_CURVE('',#12662,#12617,#2538,.T.);
#15629=EDGE_CURVE('',#12663,#12662,#2539,.T.);
#15630=EDGE_CURVE('',#12612,#12663,#2540,.T.);
#15631=EDGE_CURVE('',#12664,#12611,#2541,.T.);
#15632=EDGE_CURVE('',#12665,#12664,#2542,.T.);
#15633=EDGE_CURVE('',#12606,#12665,#2543,.T.);
#15634=EDGE_CURVE('',#12666,#12605,#2544,.T.);
#15635=EDGE_CURVE('',#12667,#12666,#2545,.T.);
#15636=EDGE_CURVE('',#12600,#12667,#2546,.T.);
#15637=EDGE_CURVE('',#12668,#12599,#2547,.T.);
#15638=EDGE_CURVE('',#12669,#12668,#2548,.T.);
#15639=EDGE_CURVE('',#12594,#12669,#2549,.T.);
#15640=EDGE_CURVE('',#12670,#12593,#2550,.T.);
#15641=EDGE_CURVE('',#12671,#12670,#2551,.T.);
#15642=EDGE_CURVE('',#12588,#12671,#2552,.T.);
#15643=EDGE_CURVE('',#12672,#12587,#2553,.T.);
#15644=EDGE_CURVE('',#12673,#12672,#2554,.T.);
#15645=EDGE_CURVE('',#12582,#12673,#2555,.T.);
#15646=EDGE_CURVE('',#12674,#12581,#2556,.T.);
#15647=EDGE_CURVE('',#12675,#12674,#2557,.T.);
#15648=EDGE_CURVE('',#12576,#12675,#2558,.T.);
#15649=EDGE_CURVE('',#12676,#12575,#2559,.T.);
#15650=EDGE_CURVE('',#12677,#12676,#2560,.T.);
#15651=EDGE_CURVE('',#12570,#12677,#2561,.T.);
#15652=EDGE_CURVE('',#12678,#12569,#2562,.T.);
#15653=EDGE_CURVE('',#12679,#12678,#2563,.T.);
#15654=EDGE_CURVE('',#12564,#12679,#2564,.T.);
#15655=EDGE_CURVE('',#12680,#12563,#2565,.T.);
#15656=EDGE_CURVE('',#12681,#12680,#2566,.T.);
#15657=EDGE_CURVE('',#12558,#12681,#2567,.T.);
#15658=EDGE_CURVE('',#12682,#12557,#2568,.T.);
#15659=EDGE_CURVE('',#12683,#12682,#2569,.T.);
#15660=EDGE_CURVE('',#12552,#12683,#2570,.T.);
#15661=EDGE_CURVE('',#12684,#12551,#2571,.T.);
#15662=EDGE_CURVE('',#12685,#12684,#2572,.T.);
#15663=EDGE_CURVE('',#12546,#12685,#2573,.T.);
#15664=EDGE_CURVE('',#12686,#12545,#2574,.T.);
#15665=EDGE_CURVE('',#12687,#12686,#2575,.T.);
#15666=EDGE_CURVE('',#12540,#12687,#2576,.T.);
#15667=EDGE_CURVE('',#12688,#12539,#2577,.T.);
#15668=EDGE_CURVE('',#12689,#12688,#2578,.T.);
#15669=EDGE_CURVE('',#12534,#12689,#2579,.T.);
#15670=EDGE_CURVE('',#12690,#12533,#2580,.T.);
#15671=EDGE_CURVE('',#12691,#12690,#2581,.T.);
#15672=EDGE_CURVE('',#12528,#12691,#2582,.T.);
#15673=EDGE_CURVE('',#12692,#12527,#2583,.T.);
#15674=EDGE_CURVE('',#12693,#12692,#2584,.T.);
#15675=EDGE_CURVE('',#12522,#12693,#2585,.T.);
#15676=EDGE_CURVE('',#12694,#12521,#2586,.T.);
#15677=EDGE_CURVE('',#12695,#12694,#2587,.T.);
#15678=EDGE_CURVE('',#12516,#12695,#2588,.T.);
#15679=EDGE_CURVE('',#12696,#12515,#2589,.T.);
#15680=EDGE_CURVE('',#12697,#12696,#2590,.T.);
#15681=EDGE_CURVE('',#12510,#12697,#2591,.T.);
#15682=EDGE_CURVE('',#12698,#12509,#2592,.T.);
#15683=EDGE_CURVE('',#12699,#12698,#2593,.T.);
#15684=EDGE_CURVE('',#12504,#12699,#2594,.T.);
#15685=EDGE_CURVE('',#12700,#12503,#2595,.T.);
#15686=EDGE_CURVE('',#12701,#12700,#2596,.T.);
#15687=EDGE_CURVE('',#12498,#12701,#2597,.T.);
#15688=EDGE_CURVE('',#12702,#12497,#2598,.T.);
#15689=EDGE_CURVE('',#12703,#12702,#2599,.T.);
#15690=EDGE_CURVE('',#12492,#12703,#2600,.T.);
#15691=EDGE_CURVE('',#12704,#12491,#2601,.T.);
#15692=EDGE_CURVE('',#12705,#12704,#2602,.T.);
#15693=EDGE_CURVE('',#12486,#12705,#2603,.T.);
#15694=EDGE_CURVE('',#12706,#12485,#2604,.T.);
#15695=EDGE_CURVE('',#12707,#12706,#2605,.T.);
#15696=EDGE_CURVE('',#12480,#12707,#2606,.T.);
#15697=EDGE_CURVE('',#12708,#12709,#2607,.T.);
#15698=EDGE_CURVE('',#12710,#12708,#10718,.T.);
#15699=EDGE_CURVE('',#12711,#12710,#2608,.T.);
#15700=EDGE_CURVE('',#12712,#12711,#2609,.T.);
#15701=EDGE_CURVE('',#12713,#12712,#2610,.T.);
#15702=EDGE_CURVE('',#12714,#12713,#10719,.T.);
#15703=EDGE_CURVE('',#12715,#12714,#2611,.T.);
#15704=EDGE_CURVE('',#12709,#12715,#2612,.T.);
#15705=EDGE_CURVE('',#12716,#12481,#2613,.T.);
#15706=EDGE_CURVE('',#12707,#12716,#2614,.T.);
#15707=EDGE_CURVE('',#12706,#12717,#2615,.T.);
#15708=EDGE_CURVE('',#12717,#12716,#2616,.T.);
#15709=EDGE_CURVE('',#12484,#12717,#2617,.T.);
#15710=EDGE_CURVE('',#12718,#12487,#2618,.T.);
#15711=EDGE_CURVE('',#12705,#12718,#2619,.T.);
#15712=EDGE_CURVE('',#12704,#12719,#2620,.T.);
#15713=EDGE_CURVE('',#12719,#12718,#2621,.T.);
#15714=EDGE_CURVE('',#12490,#12719,#2622,.T.);
#15715=EDGE_CURVE('',#12720,#12493,#2623,.T.);
#15716=EDGE_CURVE('',#12703,#12720,#2624,.T.);
#15717=EDGE_CURVE('',#12702,#12721,#2625,.T.);
#15718=EDGE_CURVE('',#12721,#12720,#2626,.T.);
#15719=EDGE_CURVE('',#12496,#12721,#2627,.T.);
#15720=EDGE_CURVE('',#12722,#12499,#2628,.T.);
#15721=EDGE_CURVE('',#12701,#12722,#2629,.T.);
#15722=EDGE_CURVE('',#12700,#12723,#2630,.T.);
#15723=EDGE_CURVE('',#12723,#12722,#2631,.T.);
#15724=EDGE_CURVE('',#12502,#12723,#2632,.T.);
#15725=EDGE_CURVE('',#12724,#12505,#2633,.T.);
#15726=EDGE_CURVE('',#12699,#12724,#2634,.T.);
#15727=EDGE_CURVE('',#12698,#12725,#2635,.T.);
#15728=EDGE_CURVE('',#12725,#12724,#2636,.T.);
#15729=EDGE_CURVE('',#12508,#12725,#2637,.T.);
#15730=EDGE_CURVE('',#12726,#12511,#2638,.T.);
#15731=EDGE_CURVE('',#12697,#12726,#2639,.T.);
#15732=EDGE_CURVE('',#12696,#12727,#2640,.T.);
#15733=EDGE_CURVE('',#12727,#12726,#2641,.T.);
#15734=EDGE_CURVE('',#12514,#12727,#2642,.T.);
#15735=EDGE_CURVE('',#12270,#12728,#2643,.T.);
#15736=EDGE_CURVE('',#12728,#12657,#2644,.F.);
#15737=EDGE_CURVE('',#12273,#12729,#2645,.T.);
#15738=EDGE_CURVE('',#12728,#12729,#2646,.T.);
#15739=EDGE_CURVE('',#12728,#12631,#2647,.T.);
#15740=EDGE_CURVE('',#12730,#12625,#2648,.T.);
#15741=EDGE_CURVE('',#12659,#12730,#2649,.T.);
#15742=EDGE_CURVE('',#12731,#12730,#2650,.T.);
#15743=EDGE_CURVE('',#12658,#12731,#2651,.T.);
#15744=EDGE_CURVE('',#12628,#12731,#2652,.T.);
#15745=EDGE_CURVE('',#12730,#12732,#2653,.T.);
#15746=EDGE_CURVE('',#12732,#12626,#2654,.T.);
#15747=EDGE_CURVE('',#12731,#12733,#2655,.T.);
#15748=EDGE_CURVE('',#12733,#12732,#2656,.T.);
#15749=EDGE_CURVE('',#12627,#12733,#2657,.T.);
#15750=EDGE_CURVE('',#12734,#12619,#2658,.T.);
#15751=EDGE_CURVE('',#12661,#12734,#2659,.T.);
#15752=EDGE_CURVE('',#12735,#12734,#2660,.T.);
#15753=EDGE_CURVE('',#12660,#12735,#2661,.T.);
#15754=EDGE_CURVE('',#12622,#12735,#2662,.T.);
#15755=EDGE_CURVE('',#12734,#12736,#2663,.T.);
#15756=EDGE_CURVE('',#12736,#12620,#2664,.T.);
#15757=EDGE_CURVE('',#12735,#12737,#2665,.T.);
#15758=EDGE_CURVE('',#12737,#12736,#2666,.T.);
#15759=EDGE_CURVE('',#12621,#12737,#2667,.T.);
#15760=EDGE_CURVE('',#12738,#12613,#2668,.T.);
#15761=EDGE_CURVE('',#12663,#12738,#2669,.T.);
#15762=EDGE_CURVE('',#12739,#12738,#2670,.T.);
#15763=EDGE_CURVE('',#12662,#12739,#2671,.T.);
#15764=EDGE_CURVE('',#12616,#12739,#2672,.T.);
#15765=EDGE_CURVE('',#12738,#12740,#2673,.T.);
#15766=EDGE_CURVE('',#12740,#12614,#2674,.T.);
#15767=EDGE_CURVE('',#12739,#12741,#2675,.T.);
#15768=EDGE_CURVE('',#12741,#12740,#2676,.T.);
#15769=EDGE_CURVE('',#12615,#12741,#2677,.T.);
#15770=EDGE_CURVE('',#12742,#12607,#2678,.T.);
#15771=EDGE_CURVE('',#12665,#12742,#2679,.T.);
#15772=EDGE_CURVE('',#12743,#12742,#2680,.T.);
#15773=EDGE_CURVE('',#12664,#12743,#2681,.T.);
#15774=EDGE_CURVE('',#12610,#12743,#2682,.T.);
#15775=EDGE_CURVE('',#12742,#12744,#2683,.T.);
#15776=EDGE_CURVE('',#12744,#12608,#2684,.T.);
#15777=EDGE_CURVE('',#12743,#12745,#2685,.T.);
#15778=EDGE_CURVE('',#12745,#12744,#2686,.T.);
#15779=EDGE_CURVE('',#12609,#12745,#2687,.T.);
#15780=EDGE_CURVE('',#12746,#12601,#2688,.T.);
#15781=EDGE_CURVE('',#12667,#12746,#2689,.T.);
#15782=EDGE_CURVE('',#12747,#12746,#2690,.T.);
#15783=EDGE_CURVE('',#12666,#12747,#2691,.T.);
#15784=EDGE_CURVE('',#12604,#12747,#2692,.T.);
#15785=EDGE_CURVE('',#12746,#12748,#2693,.T.);
#15786=EDGE_CURVE('',#12748,#12602,#2694,.T.);
#15787=EDGE_CURVE('',#12747,#12749,#2695,.T.);
#15788=EDGE_CURVE('',#12749,#12748,#2696,.T.);
#15789=EDGE_CURVE('',#12603,#12749,#2697,.T.);
#15790=EDGE_CURVE('',#12750,#12595,#2698,.T.);
#15791=EDGE_CURVE('',#12669,#12750,#2699,.T.);
#15792=EDGE_CURVE('',#12751,#12750,#2700,.T.);
#15793=EDGE_CURVE('',#12668,#12751,#2701,.T.);
#15794=EDGE_CURVE('',#12598,#12751,#2702,.T.);
#15795=EDGE_CURVE('',#12750,#12752,#2703,.T.);
#15796=EDGE_CURVE('',#12752,#12596,#2704,.T.);
#15797=EDGE_CURVE('',#12751,#12753,#2705,.T.);
#15798=EDGE_CURVE('',#12753,#12752,#2706,.T.);
#15799=EDGE_CURVE('',#12597,#12753,#2707,.T.);
#15800=EDGE_CURVE('',#12592,#12754,#2708,.T.);
#15801=EDGE_CURVE('',#12754,#12670,#2709,.F.);
#15802=EDGE_CURVE('',#12591,#12755,#2710,.T.);
#15803=EDGE_CURVE('',#12754,#12755,#2711,.T.);
#15804=EDGE_CURVE('',#12756,#12589,#2712,.T.);
#15805=EDGE_CURVE('',#12671,#12756,#2713,.T.);
#15806=EDGE_CURVE('',#12754,#12756,#2714,.T.);
#15807=EDGE_CURVE('',#12756,#12757,#2715,.T.);
#15808=EDGE_CURVE('',#12757,#12590,#2716,.T.);
#15809=EDGE_CURVE('',#12755,#12757,#2717,.T.);
#15810=EDGE_CURVE('',#12758,#12583,#2718,.T.);
#15811=EDGE_CURVE('',#12673,#12758,#2719,.T.);
#15812=EDGE_CURVE('',#12759,#12758,#2720,.T.);
#15813=EDGE_CURVE('',#12672,#12759,#2721,.T.);
#15814=EDGE_CURVE('',#12586,#12759,#2722,.T.);
#15815=EDGE_CURVE('',#12758,#12760,#2723,.T.);
#15816=EDGE_CURVE('',#12760,#12584,#2724,.T.);
#15817=EDGE_CURVE('',#12759,#12761,#2725,.T.);
#15818=EDGE_CURVE('',#12761,#12760,#2726,.T.);
#15819=EDGE_CURVE('',#12585,#12761,#2727,.T.);
#15820=EDGE_CURVE('',#12762,#12577,#2728,.T.);
#15821=EDGE_CURVE('',#12675,#12762,#2729,.T.);
#15822=EDGE_CURVE('',#12763,#12762,#2730,.T.);
#15823=EDGE_CURVE('',#12674,#12763,#2731,.T.);
#15824=EDGE_CURVE('',#12580,#12763,#2732,.T.);
#15825=EDGE_CURVE('',#12762,#12764,#2733,.T.);
#15826=EDGE_CURVE('',#12764,#12578,#2734,.T.);
#15827=EDGE_CURVE('',#12763,#12765,#2735,.T.);
#15828=EDGE_CURVE('',#12765,#12764,#2736,.T.);
#15829=EDGE_CURVE('',#12579,#12765,#2737,.T.);
#15830=EDGE_CURVE('',#12766,#12571,#2738,.T.);
#15831=EDGE_CURVE('',#12677,#12766,#2739,.T.);
#15832=EDGE_CURVE('',#12767,#12766,#2740,.T.);
#15833=EDGE_CURVE('',#12676,#12767,#2741,.T.);
#15834=EDGE_CURVE('',#12574,#12767,#2742,.T.);
#15835=EDGE_CURVE('',#12766,#12768,#2743,.T.);
#15836=EDGE_CURVE('',#12768,#12572,#2744,.T.);
#15837=EDGE_CURVE('',#12767,#12769,#2745,.T.);
#15838=EDGE_CURVE('',#12769,#12768,#2746,.T.);
#15839=EDGE_CURVE('',#12573,#12769,#2747,.T.);
#15840=EDGE_CURVE('',#12770,#12565,#2748,.T.);
#15841=EDGE_CURVE('',#12679,#12770,#2749,.T.);
#15842=EDGE_CURVE('',#12771,#12770,#2750,.T.);
#15843=EDGE_CURVE('',#12678,#12771,#2751,.T.);
#15844=EDGE_CURVE('',#12568,#12771,#2752,.T.);
#15845=EDGE_CURVE('',#12770,#12772,#2753,.T.);
#15846=EDGE_CURVE('',#12772,#12566,#2754,.T.);
#15847=EDGE_CURVE('',#12771,#12773,#2755,.T.);
#15848=EDGE_CURVE('',#12773,#12772,#2756,.T.);
#15849=EDGE_CURVE('',#12567,#12773,#2757,.T.);
#15850=EDGE_CURVE('',#12774,#12559,#2758,.T.);
#15851=EDGE_CURVE('',#12681,#12774,#2759,.T.);
#15852=EDGE_CURVE('',#12775,#12774,#2760,.T.);
#15853=EDGE_CURVE('',#12680,#12775,#2761,.T.);
#15854=EDGE_CURVE('',#12562,#12775,#2762,.T.);
#15855=EDGE_CURVE('',#12774,#12776,#2763,.T.);
#15856=EDGE_CURVE('',#12776,#12560,#2764,.T.);
#15857=EDGE_CURVE('',#12775,#12777,#2765,.T.);
#15858=EDGE_CURVE('',#12777,#12776,#2766,.T.);
#15859=EDGE_CURVE('',#12561,#12777,#2767,.T.);
#15860=EDGE_CURVE('',#12778,#12553,#2768,.T.);
#15861=EDGE_CURVE('',#12683,#12778,#2769,.T.);
#15862=EDGE_CURVE('',#12779,#12778,#2770,.T.);
#15863=EDGE_CURVE('',#12682,#12779,#2771,.T.);
#15864=EDGE_CURVE('',#12556,#12779,#2772,.T.);
#15865=EDGE_CURVE('',#12778,#12780,#2773,.T.);
#15866=EDGE_CURVE('',#12780,#12554,#2774,.T.);
#15867=EDGE_CURVE('',#12779,#12781,#2775,.T.);
#15868=EDGE_CURVE('',#12781,#12780,#2776,.T.);
#15869=EDGE_CURVE('',#12555,#12781,#2777,.T.);
#15870=EDGE_CURVE('',#12782,#12547,#2778,.T.);
#15871=EDGE_CURVE('',#12685,#12782,#2779,.T.);
#15872=EDGE_CURVE('',#12783,#12782,#2780,.T.);
#15873=EDGE_CURVE('',#12684,#12783,#2781,.T.);
#15874=EDGE_CURVE('',#12550,#12783,#2782,.T.);
#15875=EDGE_CURVE('',#12782,#12784,#2783,.T.);
#15876=EDGE_CURVE('',#12784,#12548,#2784,.T.);
#15877=EDGE_CURVE('',#12783,#12785,#2785,.T.);
#15878=EDGE_CURVE('',#12785,#12784,#2786,.T.);
#15879=EDGE_CURVE('',#12549,#12785,#2787,.T.);
#15880=EDGE_CURVE('',#12786,#12541,#2788,.T.);
#15881=EDGE_CURVE('',#12687,#12786,#2789,.T.);
#15882=EDGE_CURVE('',#12787,#12786,#2790,.T.);
#15883=EDGE_CURVE('',#12686,#12787,#2791,.T.);
#15884=EDGE_CURVE('',#12544,#12787,#2792,.T.);
#15885=EDGE_CURVE('',#12786,#12788,#2793,.T.);
#15886=EDGE_CURVE('',#12788,#12542,#2794,.T.);
#15887=EDGE_CURVE('',#12787,#12789,#2795,.T.);
#15888=EDGE_CURVE('',#12789,#12788,#2796,.T.);
#15889=EDGE_CURVE('',#12543,#12789,#2797,.T.);
#15890=EDGE_CURVE('',#12790,#12535,#2798,.T.);
#15891=EDGE_CURVE('',#12689,#12790,#2799,.T.);
#15892=EDGE_CURVE('',#12791,#12790,#2800,.T.);
#15893=EDGE_CURVE('',#12688,#12791,#2801,.T.);
#15894=EDGE_CURVE('',#12538,#12791,#2802,.T.);
#15895=EDGE_CURVE('',#12790,#12792,#2803,.T.);
#15896=EDGE_CURVE('',#12792,#12536,#2804,.T.);
#15897=EDGE_CURVE('',#12791,#12793,#2805,.T.);
#15898=EDGE_CURVE('',#12793,#12792,#2806,.T.);
#15899=EDGE_CURVE('',#12537,#12793,#2807,.T.);
#15900=EDGE_CURVE('',#12794,#12529,#2808,.T.);
#15901=EDGE_CURVE('',#12691,#12794,#2809,.T.);
#15902=EDGE_CURVE('',#12795,#12794,#2810,.T.);
#15903=EDGE_CURVE('',#12690,#12795,#2811,.T.);
#15904=EDGE_CURVE('',#12532,#12795,#2812,.T.);
#15905=EDGE_CURVE('',#12794,#12796,#2813,.T.);
#15906=EDGE_CURVE('',#12796,#12530,#2814,.T.);
#15907=EDGE_CURVE('',#12795,#12797,#2815,.T.);
#15908=EDGE_CURVE('',#12797,#12796,#2816,.T.);
#15909=EDGE_CURVE('',#12531,#12797,#2817,.T.);
#15910=EDGE_CURVE('',#12798,#12523,#2818,.T.);
#15911=EDGE_CURVE('',#12693,#12798,#2819,.T.);
#15912=EDGE_CURVE('',#12799,#12798,#2820,.T.);
#15913=EDGE_CURVE('',#12692,#12799,#2821,.T.);
#15914=EDGE_CURVE('',#12526,#12799,#2822,.T.);
#15915=EDGE_CURVE('',#12798,#12800,#2823,.T.);
#15916=EDGE_CURVE('',#12800,#12524,#2824,.T.);
#15917=EDGE_CURVE('',#12799,#12801,#2825,.T.);
#15918=EDGE_CURVE('',#12801,#12800,#2826,.T.);
#15919=EDGE_CURVE('',#12525,#12801,#2827,.T.);
#15920=EDGE_CURVE('',#12802,#12517,#2828,.T.);
#15921=EDGE_CURVE('',#12695,#12802,#2829,.T.);
#15922=EDGE_CURVE('',#12803,#12802,#2830,.T.);
#15923=EDGE_CURVE('',#12694,#12803,#2831,.T.);
#15924=EDGE_CURVE('',#12520,#12803,#2832,.T.);
#15925=EDGE_CURVE('',#12802,#12804,#2833,.T.);
#15926=EDGE_CURVE('',#12804,#12518,#2834,.T.);
#15927=EDGE_CURVE('',#12803,#12805,#2835,.T.);
#15928=EDGE_CURVE('',#12805,#12804,#2836,.T.);
#15929=EDGE_CURVE('',#12519,#12805,#2837,.T.);
#15930=EDGE_CURVE('',#12806,#12807,#2838,.T.);
#15931=EDGE_CURVE('',#12807,#12808,#2839,.F.);
#15932=EDGE_CURVE('',#12808,#12809,#2840,.T.);
#15933=EDGE_CURVE('',#12809,#12806,#2841,.T.);
#15934=EDGE_CURVE('',#12809,#12421,#2842,.T.);
#15935=EDGE_CURVE('',#12420,#12806,#2843,.T.);
#15936=EDGE_CURVE('',#12807,#12425,#2844,.T.);
#15937=EDGE_CURVE('',#12810,#12419,#2845,.T.);
#15938=EDGE_CURVE('',#12811,#12810,#2846,.T.);
#15939=EDGE_CURVE('',#12414,#12811,#2847,.T.);
#15940=EDGE_CURVE('',#12812,#12413,#2848,.T.);
#15941=EDGE_CURVE('',#12813,#12812,#2849,.T.);
#15942=EDGE_CURVE('',#12408,#12813,#2850,.T.);
#15943=EDGE_CURVE('',#12814,#12407,#2851,.T.);
#15944=EDGE_CURVE('',#12815,#12814,#2852,.T.);
#15945=EDGE_CURVE('',#12402,#12815,#2853,.T.);
#15946=EDGE_CURVE('',#12816,#12401,#2854,.T.);
#15947=EDGE_CURVE('',#12817,#12816,#2855,.T.);
#15948=EDGE_CURVE('',#12396,#12817,#2856,.T.);
#15949=EDGE_CURVE('',#12818,#12395,#2857,.T.);
#15950=EDGE_CURVE('',#12819,#12818,#2858,.T.);
#15951=EDGE_CURVE('',#12390,#12819,#2859,.T.);
#15952=EDGE_CURVE('',#12820,#12389,#2860,.T.);
#15953=EDGE_CURVE('',#12821,#12820,#2861,.T.);
#15954=EDGE_CURVE('',#12384,#12821,#2862,.T.);
#15955=EDGE_CURVE('',#12822,#12383,#2863,.T.);
#15956=EDGE_CURVE('',#12823,#12822,#2864,.T.);
#15957=EDGE_CURVE('',#12378,#12823,#2865,.T.);
#15958=EDGE_CURVE('',#12824,#12377,#2866,.T.);
#15959=EDGE_CURVE('',#12825,#12824,#2867,.T.);
#15960=EDGE_CURVE('',#12372,#12825,#2868,.T.);
#15961=EDGE_CURVE('',#12826,#12371,#2869,.T.);
#15962=EDGE_CURVE('',#12827,#12826,#2870,.T.);
#15963=EDGE_CURVE('',#12366,#12827,#2871,.T.);
#15964=EDGE_CURVE('',#12828,#12365,#2872,.T.);
#15965=EDGE_CURVE('',#12829,#12828,#2873,.T.);
#15966=EDGE_CURVE('',#12360,#12829,#2874,.T.);
#15967=EDGE_CURVE('',#12830,#12359,#2875,.T.);
#15968=EDGE_CURVE('',#12831,#12830,#2876,.T.);
#15969=EDGE_CURVE('',#12354,#12831,#2877,.T.);
#15970=EDGE_CURVE('',#12832,#12353,#2878,.T.);
#15971=EDGE_CURVE('',#12833,#12832,#2879,.T.);
#15972=EDGE_CURVE('',#12348,#12833,#2880,.T.);
#15973=EDGE_CURVE('',#12834,#12347,#2881,.T.);
#15974=EDGE_CURVE('',#12835,#12834,#2882,.T.);
#15975=EDGE_CURVE('',#12342,#12835,#2883,.T.);
#15976=EDGE_CURVE('',#12836,#12341,#2884,.T.);
#15977=EDGE_CURVE('',#12837,#12836,#2885,.T.);
#15978=EDGE_CURVE('',#12336,#12837,#2886,.T.);
#15979=EDGE_CURVE('',#12838,#12335,#2887,.T.);
#15980=EDGE_CURVE('',#12839,#12838,#2888,.T.);
#15981=EDGE_CURVE('',#12330,#12839,#2889,.T.);
#15982=EDGE_CURVE('',#12840,#12329,#2890,.T.);
#15983=EDGE_CURVE('',#12841,#12840,#2891,.T.);
#15984=EDGE_CURVE('',#12324,#12841,#2892,.T.);
#15985=EDGE_CURVE('',#12842,#12323,#2893,.T.);
#15986=EDGE_CURVE('',#12843,#12842,#2894,.T.);
#15987=EDGE_CURVE('',#12318,#12843,#2895,.T.);
#15988=EDGE_CURVE('',#12844,#12317,#2896,.T.);
#15989=EDGE_CURVE('',#12845,#12844,#2897,.T.);
#15990=EDGE_CURVE('',#12312,#12845,#2898,.T.);
#15991=EDGE_CURVE('',#12846,#12311,#2899,.T.);
#15992=EDGE_CURVE('',#12847,#12846,#2900,.T.);
#15993=EDGE_CURVE('',#12306,#12847,#2901,.T.);
#15994=EDGE_CURVE('',#12848,#12305,#2902,.T.);
#15995=EDGE_CURVE('',#12849,#12848,#2903,.T.);
#15996=EDGE_CURVE('',#12300,#12849,#2904,.T.);
#15997=EDGE_CURVE('',#12850,#12299,#2905,.T.);
#15998=EDGE_CURVE('',#12851,#12850,#2906,.T.);
#15999=EDGE_CURVE('',#12294,#12851,#2907,.T.);
#16000=EDGE_CURVE('',#12852,#12293,#2908,.T.);
#16001=EDGE_CURVE('',#12853,#12852,#2909,.T.);
#16002=EDGE_CURVE('',#12288,#12853,#2910,.T.);
#16003=EDGE_CURVE('',#12854,#12467,#2911,.T.);
#16004=EDGE_CURVE('',#12855,#12854,#2912,.T.);
#16005=EDGE_CURVE('',#12462,#12855,#2913,.T.);
#16006=EDGE_CURVE('',#12856,#12461,#2914,.T.);
#16007=EDGE_CURVE('',#12857,#12856,#2915,.T.);
#16008=EDGE_CURVE('',#12456,#12857,#2916,.T.);
#16009=EDGE_CURVE('',#12858,#12455,#2917,.T.);
#16010=EDGE_CURVE('',#12859,#12858,#2918,.T.);
#16011=EDGE_CURVE('',#12450,#12859,#2919,.T.);
#16012=EDGE_CURVE('',#12860,#12449,#2920,.T.);
#16013=EDGE_CURVE('',#12861,#12860,#2921,.T.);
#16014=EDGE_CURVE('',#12444,#12861,#2922,.T.);
#16015=EDGE_CURVE('',#12862,#12443,#2923,.T.);
#16016=EDGE_CURVE('',#12863,#12862,#2924,.T.);
#16017=EDGE_CURVE('',#12438,#12863,#2925,.T.);
#16018=EDGE_CURVE('',#12864,#12437,#2926,.T.);
#16019=EDGE_CURVE('',#12865,#12864,#2927,.T.);
#16020=EDGE_CURVE('',#12432,#12865,#2928,.T.);
#16021=EDGE_CURVE('',#12866,#12431,#2929,.T.);
#16022=EDGE_CURVE('',#12867,#12866,#2930,.T.);
#16023=EDGE_CURVE('',#12426,#12867,#2931,.T.);
#16024=EDGE_CURVE('',#12868,#12869,#2932,.T.);
#16025=EDGE_CURVE('',#12870,#12868,#2933,.T.);
#16026=EDGE_CURVE('',#12871,#12870,#2934,.T.);
#16027=EDGE_CURVE('',#12871,#12872,#10720,.T.);
#16028=EDGE_CURVE('',#12873,#12872,#2935,.T.);
#16029=EDGE_CURVE('',#12874,#12873,#2936,.T.);
#16030=EDGE_CURVE('',#12875,#12874,#2937,.T.);
#16031=EDGE_CURVE('',#12875,#12869,#10721,.T.);
#16032=EDGE_CURVE('',#12424,#12808,#2938,.T.);
#16033=EDGE_CURVE('',#12866,#12876,#2939,.T.);
#16034=EDGE_CURVE('',#12876,#12877,#2940,.T.);
#16035=EDGE_CURVE('',#12877,#12867,#2941,.T.);
#16036=EDGE_CURVE('',#12430,#12876,#2942,.T.);
#16037=EDGE_CURVE('',#12877,#12427,#2943,.T.);
#16038=EDGE_CURVE('',#12864,#12878,#2944,.T.);
#16039=EDGE_CURVE('',#12878,#12879,#2945,.T.);
#16040=EDGE_CURVE('',#12879,#12865,#2946,.T.);
#16041=EDGE_CURVE('',#12436,#12878,#2947,.T.);
#16042=EDGE_CURVE('',#12879,#12433,#2948,.T.);
#16043=EDGE_CURVE('',#12879,#12880,#2949,.T.);
#16044=EDGE_CURVE('',#12880,#12434,#2950,.T.);
#16045=EDGE_CURVE('',#12878,#12881,#2951,.T.);
#16046=EDGE_CURVE('',#12881,#12880,#2952,.T.);
#16047=EDGE_CURVE('',#12862,#12882,#2953,.T.);
#16048=EDGE_CURVE('',#12882,#12883,#2954,.T.);
#16049=EDGE_CURVE('',#12883,#12863,#2955,.T.);
#16050=EDGE_CURVE('',#12442,#12882,#2956,.T.);
#16051=EDGE_CURVE('',#12883,#12439,#2957,.T.);
#16052=EDGE_CURVE('',#12860,#12884,#2958,.T.);
#16053=EDGE_CURVE('',#12884,#12885,#2959,.T.);
#16054=EDGE_CURVE('',#12885,#12861,#2960,.T.);
#16055=EDGE_CURVE('',#12448,#12884,#2961,.T.);
#16056=EDGE_CURVE('',#12885,#12445,#2962,.T.);
#16057=EDGE_CURVE('',#12885,#12886,#2963,.T.);
#16058=EDGE_CURVE('',#12886,#12446,#2964,.T.);
#16059=EDGE_CURVE('',#12884,#12887,#2965,.T.);
#16060=EDGE_CURVE('',#12887,#12886,#2966,.T.);
#16061=EDGE_CURVE('',#12858,#12888,#2967,.T.);
#16062=EDGE_CURVE('',#12888,#12889,#2968,.T.);
#16063=EDGE_CURVE('',#12889,#12859,#2969,.T.);
#16064=EDGE_CURVE('',#12454,#12888,#2970,.T.);
#16065=EDGE_CURVE('',#12889,#12451,#2971,.T.);
#16066=EDGE_CURVE('',#12856,#12890,#2972,.T.);
#16067=EDGE_CURVE('',#12890,#12891,#2973,.T.);
#16068=EDGE_CURVE('',#12891,#12857,#2974,.T.);
#16069=EDGE_CURVE('',#12460,#12890,#2975,.T.);
#16070=EDGE_CURVE('',#12891,#12457,#2976,.T.);
#16071=EDGE_CURVE('',#12891,#12892,#2977,.T.);
#16072=EDGE_CURVE('',#12892,#12458,#2978,.T.);
#16073=EDGE_CURVE('',#12890,#12893,#2979,.T.);
#16074=EDGE_CURVE('',#12893,#12892,#2980,.T.);
#16075=EDGE_CURVE('',#12855,#12894,#2981,.F.);
#16076=EDGE_CURVE('',#12894,#12463,#2982,.T.);
#16077=EDGE_CURVE('',#12895,#12894,#2983,.T.);
#16078=EDGE_CURVE('',#12854,#12895,#2984,.T.);
#16079=EDGE_CURVE('',#12466,#12895,#2985,.T.);
#16080=EDGE_CURVE('',#12852,#12896,#2986,.T.);
#16081=EDGE_CURVE('',#12896,#12897,#2987,.T.);
#16082=EDGE_CURVE('',#12897,#12853,#2988,.T.);
#16083=EDGE_CURVE('',#12292,#12896,#2989,.T.);
#16084=EDGE_CURVE('',#12897,#12289,#2990,.T.);
#16085=EDGE_CURVE('',#12850,#12898,#2991,.T.);
#16086=EDGE_CURVE('',#12898,#12899,#2992,.T.);
#16087=EDGE_CURVE('',#12899,#12851,#2993,.T.);
#16088=EDGE_CURVE('',#12298,#12898,#2994,.T.);
#16089=EDGE_CURVE('',#12899,#12295,#2995,.T.);
#16090=EDGE_CURVE('',#12899,#12900,#2996,.T.);
#16091=EDGE_CURVE('',#12900,#12296,#2997,.T.);
#16092=EDGE_CURVE('',#12898,#12901,#2998,.T.);
#16093=EDGE_CURVE('',#12901,#12900,#2999,.T.);
#16094=EDGE_CURVE('',#12848,#12902,#3000,.T.);
#16095=EDGE_CURVE('',#12902,#12903,#3001,.T.);
#16096=EDGE_CURVE('',#12903,#12849,#3002,.T.);
#16097=EDGE_CURVE('',#12304,#12902,#3003,.T.);
#16098=EDGE_CURVE('',#12903,#12301,#3004,.T.);
#16099=EDGE_CURVE('',#12846,#12904,#3005,.T.);
#16100=EDGE_CURVE('',#12904,#12905,#3006,.T.);
#16101=EDGE_CURVE('',#12905,#12847,#3007,.T.);
#16102=EDGE_CURVE('',#12310,#12904,#3008,.T.);
#16103=EDGE_CURVE('',#12905,#12307,#3009,.T.);
#16104=EDGE_CURVE('',#12905,#12906,#3010,.T.);
#16105=EDGE_CURVE('',#12906,#12308,#3011,.T.);
#16106=EDGE_CURVE('',#12904,#12907,#3012,.T.);
#16107=EDGE_CURVE('',#12907,#12906,#3013,.T.);
#16108=EDGE_CURVE('',#12844,#12908,#3014,.T.);
#16109=EDGE_CURVE('',#12908,#12909,#3015,.T.);
#16110=EDGE_CURVE('',#12909,#12845,#3016,.T.);
#16111=EDGE_CURVE('',#12316,#12908,#3017,.T.);
#16112=EDGE_CURVE('',#12909,#12313,#3018,.T.);
#16113=EDGE_CURVE('',#12842,#12910,#3019,.T.);
#16114=EDGE_CURVE('',#12910,#12911,#3020,.T.);
#16115=EDGE_CURVE('',#12911,#12843,#3021,.T.);
#16116=EDGE_CURVE('',#12322,#12910,#3022,.T.);
#16117=EDGE_CURVE('',#12911,#12319,#3023,.T.);
#16118=EDGE_CURVE('',#12911,#12912,#3024,.T.);
#16119=EDGE_CURVE('',#12912,#12320,#3025,.T.);
#16120=EDGE_CURVE('',#12910,#12913,#3026,.T.);
#16121=EDGE_CURVE('',#12913,#12912,#3027,.T.);
#16122=EDGE_CURVE('',#12840,#12914,#3028,.T.);
#16123=EDGE_CURVE('',#12914,#12915,#3029,.T.);
#16124=EDGE_CURVE('',#12915,#12841,#3030,.T.);
#16125=EDGE_CURVE('',#12328,#12914,#3031,.T.);
#16126=EDGE_CURVE('',#12915,#12325,#3032,.T.);
#16127=EDGE_CURVE('',#12838,#12916,#3033,.T.);
#16128=EDGE_CURVE('',#12916,#12917,#3034,.T.);
#16129=EDGE_CURVE('',#12917,#12839,#3035,.T.);
#16130=EDGE_CURVE('',#12334,#12916,#3036,.T.);
#16131=EDGE_CURVE('',#12917,#12331,#3037,.T.);
#16132=EDGE_CURVE('',#12917,#12918,#3038,.T.);
#16133=EDGE_CURVE('',#12918,#12332,#3039,.T.);
#16134=EDGE_CURVE('',#12916,#12919,#3040,.T.);
#16135=EDGE_CURVE('',#12919,#12918,#3041,.T.);
#16136=EDGE_CURVE('',#12836,#12920,#3042,.T.);
#16137=EDGE_CURVE('',#12920,#12921,#3043,.T.);
#16138=EDGE_CURVE('',#12921,#12837,#3044,.T.);
#16139=EDGE_CURVE('',#12340,#12920,#3045,.T.);
#16140=EDGE_CURVE('',#12921,#12337,#3046,.T.);
#16141=EDGE_CURVE('',#12834,#12922,#3047,.T.);
#16142=EDGE_CURVE('',#12922,#12923,#3048,.T.);
#16143=EDGE_CURVE('',#12923,#12835,#3049,.T.);
#16144=EDGE_CURVE('',#12346,#12922,#3050,.T.);
#16145=EDGE_CURVE('',#12923,#12343,#3051,.T.);
#16146=EDGE_CURVE('',#12923,#12924,#3052,.T.);
#16147=EDGE_CURVE('',#12924,#12344,#3053,.T.);
#16148=EDGE_CURVE('',#12922,#12925,#3054,.T.);
#16149=EDGE_CURVE('',#12925,#12924,#3055,.T.);
#16150=EDGE_CURVE('',#12832,#12926,#3056,.T.);
#16151=EDGE_CURVE('',#12926,#12927,#3057,.T.);
#16152=EDGE_CURVE('',#12927,#12833,#3058,.T.);
#16153=EDGE_CURVE('',#12352,#12926,#3059,.T.);
#16154=EDGE_CURVE('',#12927,#12349,#3060,.T.);
#16155=EDGE_CURVE('',#12830,#12928,#3061,.T.);
#16156=EDGE_CURVE('',#12928,#12929,#3062,.T.);
#16157=EDGE_CURVE('',#12929,#12831,#3063,.T.);
#16158=EDGE_CURVE('',#12358,#12928,#3064,.T.);
#16159=EDGE_CURVE('',#12929,#12355,#3065,.T.);
#16160=EDGE_CURVE('',#12929,#12930,#3066,.T.);
#16161=EDGE_CURVE('',#12930,#12356,#3067,.T.);
#16162=EDGE_CURVE('',#12928,#12931,#3068,.T.);
#16163=EDGE_CURVE('',#12931,#12930,#3069,.T.);
#16164=EDGE_CURVE('',#12828,#12932,#3070,.F.);
#16165=EDGE_CURVE('',#12932,#12933,#3071,.T.);
#16166=EDGE_CURVE('',#12933,#12829,#3072,.T.);
#16167=EDGE_CURVE('',#12933,#12361,#3073,.T.);
#16168=EDGE_CURVE('',#12364,#12932,#3074,.T.);
#16169=EDGE_CURVE('',#12826,#12934,#3075,.T.);
#16170=EDGE_CURVE('',#12934,#12935,#3076,.T.);
#16171=EDGE_CURVE('',#12935,#12827,#3077,.T.);
#16172=EDGE_CURVE('',#12370,#12934,#3078,.T.);
#16173=EDGE_CURVE('',#12935,#12367,#3079,.T.);
#16174=EDGE_CURVE('',#12824,#12936,#3080,.T.);
#16175=EDGE_CURVE('',#12936,#12937,#3081,.T.);
#16176=EDGE_CURVE('',#12937,#12825,#3082,.T.);
#16177=EDGE_CURVE('',#12376,#12936,#3083,.T.);
#16178=EDGE_CURVE('',#12937,#12373,#3084,.T.);
#16179=EDGE_CURVE('',#12937,#12938,#3085,.T.);
#16180=EDGE_CURVE('',#12938,#12374,#3086,.T.);
#16181=EDGE_CURVE('',#12936,#12939,#3087,.T.);
#16182=EDGE_CURVE('',#12939,#12938,#3088,.T.);
#16183=EDGE_CURVE('',#12822,#12940,#3089,.T.);
#16184=EDGE_CURVE('',#12940,#12941,#3090,.T.);
#16185=EDGE_CURVE('',#12941,#12823,#3091,.T.);
#16186=EDGE_CURVE('',#12382,#12940,#3092,.T.);
#16187=EDGE_CURVE('',#12941,#12379,#3093,.T.);
#16188=EDGE_CURVE('',#12820,#12942,#3094,.T.);
#16189=EDGE_CURVE('',#12942,#12943,#3095,.T.);
#16190=EDGE_CURVE('',#12943,#12821,#3096,.T.);
#16191=EDGE_CURVE('',#12388,#12942,#3097,.T.);
#16192=EDGE_CURVE('',#12943,#12385,#3098,.T.);
#16193=EDGE_CURVE('',#12943,#12944,#3099,.T.);
#16194=EDGE_CURVE('',#12944,#12386,#3100,.T.);
#16195=EDGE_CURVE('',#12942,#12945,#3101,.T.);
#16196=EDGE_CURVE('',#12945,#12944,#3102,.T.);
#16197=EDGE_CURVE('',#12818,#12946,#3103,.T.);
#16198=EDGE_CURVE('',#12946,#12947,#3104,.T.);
#16199=EDGE_CURVE('',#12947,#12819,#3105,.T.);
#16200=EDGE_CURVE('',#12394,#12946,#3106,.T.);
#16201=EDGE_CURVE('',#12947,#12391,#3107,.T.);
#16202=EDGE_CURVE('',#12816,#12948,#3108,.T.);
#16203=EDGE_CURVE('',#12948,#12949,#3109,.T.);
#16204=EDGE_CURVE('',#12949,#12817,#3110,.T.);
#16205=EDGE_CURVE('',#12400,#12948,#3111,.T.);
#16206=EDGE_CURVE('',#12949,#12397,#3112,.T.);
#16207=EDGE_CURVE('',#12949,#12950,#3113,.T.);
#16208=EDGE_CURVE('',#12950,#12398,#3114,.T.);
#16209=EDGE_CURVE('',#12948,#12951,#3115,.T.);
#16210=EDGE_CURVE('',#12951,#12950,#3116,.T.);
#16211=EDGE_CURVE('',#12815,#12952,#3117,.F.);
#16212=EDGE_CURVE('',#12952,#12403,#3118,.T.);
#16213=EDGE_CURVE('',#12953,#12952,#3119,.T.);
#16214=EDGE_CURVE('',#12814,#12953,#3120,.T.);
#16215=EDGE_CURVE('',#12406,#12953,#3121,.T.);
#16216=EDGE_CURVE('',#12812,#12954,#3122,.T.);
#16217=EDGE_CURVE('',#12954,#12955,#3123,.T.);
#16218=EDGE_CURVE('',#12955,#12813,#3124,.T.);
#16219=EDGE_CURVE('',#12412,#12954,#3125,.T.);
#16220=EDGE_CURVE('',#12955,#12409,#3126,.T.);
#16221=EDGE_CURVE('',#12810,#12956,#3127,.T.);
#16222=EDGE_CURVE('',#12956,#12957,#3128,.T.);
#16223=EDGE_CURVE('',#12957,#12811,#3129,.T.);
#16224=EDGE_CURVE('',#12418,#12956,#3130,.T.);
#16225=EDGE_CURVE('',#12957,#12415,#3131,.T.);
#16226=EDGE_CURVE('',#12957,#12958,#3132,.T.);
#16227=EDGE_CURVE('',#12958,#12416,#3133,.T.);
#16228=EDGE_CURVE('',#12956,#12959,#3134,.T.);
#16229=EDGE_CURVE('',#12959,#12958,#3135,.T.);
#16230=EDGE_CURVE('',#12715,#12960,#3136,.T.);
#16231=EDGE_CURVE('',#12960,#12961,#3137,.T.);
#16232=EDGE_CURVE('',#12961,#12709,#3138,.T.);
#16233=EDGE_CURVE('',#12714,#12962,#322,.T.);
#16234=EDGE_CURVE('',#12962,#12960,#3139,.T.);
#16235=EDGE_CURVE('',#12961,#12963,#3140,.T.);
#16236=EDGE_CURVE('',#12963,#12708,#323,.T.);
#16237=EDGE_CURVE('',#12964,#12961,#3141,.T.);
#16238=EDGE_CURVE('',#12965,#12964,#3142,.T.);
#16239=EDGE_CURVE('',#12963,#12965,#3143,.T.);
#16240=EDGE_CURVE('',#12966,#12960,#3144,.T.);
#16241=EDGE_CURVE('',#12964,#12966,#3145,.T.);
#16242=EDGE_CURVE('',#12967,#12962,#3146,.T.);
#16243=EDGE_CURVE('',#12966,#12967,#3147,.T.);
#16244=EDGE_CURVE('',#12968,#12713,#324,.T.);
#16245=EDGE_CURVE('',#12968,#12969,#3148,.T.);
#16246=EDGE_CURVE('',#12872,#12969,#325,.T.);
#16247=EDGE_CURVE('',#12967,#12871,#326,.T.);
#16248=EDGE_CURVE('',#12966,#12870,#3149,.T.);
#16249=EDGE_CURVE('',#12868,#12964,#3150,.T.);
#16250=EDGE_CURVE('',#12869,#12965,#327,.T.);
#16251=EDGE_CURVE('',#12970,#12971,#3151,.T.);
#16252=EDGE_CURVE('',#12971,#12875,#328,.T.);
#16253=EDGE_CURVE('',#12874,#12970,#3152,.T.);
#16254=EDGE_CURVE('',#12873,#12972,#3153,.T.);
#16255=EDGE_CURVE('',#12972,#12970,#3154,.T.);
#16256=EDGE_CURVE('',#12969,#12972,#3155,.T.);
#16257=EDGE_CURVE('',#12970,#12973,#3156,.T.);
#16258=EDGE_CURVE('',#12974,#12973,#3157,.T.);
#16259=EDGE_CURVE('',#12971,#12974,#3158,.T.);
#16260=EDGE_CURVE('',#12972,#12975,#3159,.T.);
#16261=EDGE_CURVE('',#12973,#12975,#3160,.T.);
#16262=EDGE_CURVE('',#12975,#12968,#3161,.T.);
#16263=EDGE_CURVE('',#12710,#12974,#329,.T.);
#16264=EDGE_CURVE('',#12973,#12711,#3162,.T.);
#16265=EDGE_CURVE('',#12975,#12712,#3163,.T.);
#16266=EDGE_CURVE('',#12417,#12959,#3164,.T.);
#16267=EDGE_CURVE('',#12954,#12976,#3165,.T.);
#16268=EDGE_CURVE('',#12976,#12977,#3166,.T.);
#16269=EDGE_CURVE('',#12955,#12977,#3167,.T.);
#16270=EDGE_CURVE('',#12411,#12976,#3168,.T.);
#16271=EDGE_CURVE('',#12977,#12410,#3169,.T.);
#16272=EDGE_CURVE('',#12953,#12978,#3170,.T.);
#16273=EDGE_CURVE('',#12978,#12979,#3171,.T.);
#16274=EDGE_CURVE('',#12952,#12979,#3172,.T.);
#16275=EDGE_CURVE('',#12405,#12978,#3173,.T.);
#16276=EDGE_CURVE('',#12979,#12404,#3174,.T.);
#16277=EDGE_CURVE('',#12399,#12951,#3175,.T.);
#16278=EDGE_CURVE('',#12946,#12980,#3176,.T.);
#16279=EDGE_CURVE('',#12980,#12981,#3177,.T.);
#16280=EDGE_CURVE('',#12947,#12981,#3178,.T.);
#16281=EDGE_CURVE('',#12393,#12980,#3179,.T.);
#16282=EDGE_CURVE('',#12981,#12392,#3180,.T.);
#16283=EDGE_CURVE('',#12387,#12945,#3181,.T.);
#16284=EDGE_CURVE('',#12940,#12982,#3182,.T.);
#16285=EDGE_CURVE('',#12982,#12983,#3183,.T.);
#16286=EDGE_CURVE('',#12941,#12983,#3184,.T.);
#16287=EDGE_CURVE('',#12381,#12982,#3185,.T.);
#16288=EDGE_CURVE('',#12983,#12380,#3186,.T.);
#16289=EDGE_CURVE('',#12375,#12939,#3187,.T.);
#16290=EDGE_CURVE('',#12934,#12984,#3188,.T.);
#16291=EDGE_CURVE('',#12984,#12985,#3189,.T.);
#16292=EDGE_CURVE('',#12935,#12985,#3190,.T.);
#16293=EDGE_CURVE('',#12369,#12984,#3191,.T.);
#16294=EDGE_CURVE('',#12985,#12368,#3192,.T.);
#16295=EDGE_CURVE('',#12932,#12986,#3193,.T.);
#16296=EDGE_CURVE('',#12986,#12987,#3194,.T.);
#16297=EDGE_CURVE('',#12933,#12987,#3195,.T.);
#16298=EDGE_CURVE('',#12363,#12986,#3196,.T.);
#16299=EDGE_CURVE('',#12987,#12362,#3197,.T.);
#16300=EDGE_CURVE('',#12357,#12931,#3198,.T.);
#16301=EDGE_CURVE('',#12926,#12988,#3199,.T.);
#16302=EDGE_CURVE('',#12988,#12989,#3200,.T.);
#16303=EDGE_CURVE('',#12927,#12989,#3201,.T.);
#16304=EDGE_CURVE('',#12351,#12988,#3202,.T.);
#16305=EDGE_CURVE('',#12989,#12350,#3203,.T.);
#16306=EDGE_CURVE('',#12345,#12925,#3204,.T.);
#16307=EDGE_CURVE('',#12920,#12990,#3205,.T.);
#16308=EDGE_CURVE('',#12990,#12991,#3206,.T.);
#16309=EDGE_CURVE('',#12921,#12991,#3207,.T.);
#16310=EDGE_CURVE('',#12339,#12990,#3208,.T.);
#16311=EDGE_CURVE('',#12991,#12338,#3209,.T.);
#16312=EDGE_CURVE('',#12333,#12919,#3210,.T.);
#16313=EDGE_CURVE('',#12914,#12992,#3211,.T.);
#16314=EDGE_CURVE('',#12992,#12993,#3212,.T.);
#16315=EDGE_CURVE('',#12915,#12993,#3213,.T.);
#16316=EDGE_CURVE('',#12327,#12992,#3214,.T.);
#16317=EDGE_CURVE('',#12993,#12326,#3215,.T.);
#16318=EDGE_CURVE('',#12321,#12913,#3216,.T.);
#16319=EDGE_CURVE('',#12908,#12994,#3217,.T.);
#16320=EDGE_CURVE('',#12994,#12995,#3218,.T.);
#16321=EDGE_CURVE('',#12909,#12995,#3219,.T.);
#16322=EDGE_CURVE('',#12315,#12994,#3220,.T.);
#16323=EDGE_CURVE('',#12995,#12314,#3221,.T.);
#16324=EDGE_CURVE('',#12309,#12907,#3222,.T.);
#16325=EDGE_CURVE('',#12729,#12632,#3223,.T.);
#16326=EDGE_CURVE('',#12902,#12996,#3224,.T.);
#16327=EDGE_CURVE('',#12996,#12997,#3225,.T.);
#16328=EDGE_CURVE('',#12903,#12997,#3226,.T.);
#16329=EDGE_CURVE('',#12303,#12996,#3227,.T.);
#16330=EDGE_CURVE('',#12997,#12302,#3228,.T.);
#16331=EDGE_CURVE('',#12297,#12901,#3229,.T.);
#16332=EDGE_CURVE('',#12896,#12998,#3230,.T.);
#16333=EDGE_CURVE('',#12998,#12999,#3231,.T.);
#16334=EDGE_CURVE('',#12897,#12999,#3232,.T.);
#16335=EDGE_CURVE('',#12291,#12998,#3233,.T.);
#16336=EDGE_CURVE('',#12999,#12290,#3234,.T.);
#16337=EDGE_CURVE('',#12895,#13000,#3235,.T.);
#16338=EDGE_CURVE('',#13000,#13001,#3236,.T.);
#16339=EDGE_CURVE('',#12894,#13001,#3237,.T.);
#16340=EDGE_CURVE('',#12465,#13000,#3238,.T.);
#16341=EDGE_CURVE('',#13001,#12464,#3239,.T.);
#16342=EDGE_CURVE('',#12477,#12656,#3240,.T.);
#16343=EDGE_CURVE('',#12459,#12893,#3241,.T.);
#16344=EDGE_CURVE('',#12716,#13002,#3242,.T.);
#16345=EDGE_CURVE('',#13002,#12482,#3243,.T.);
#16346=EDGE_CURVE('',#13003,#13002,#3244,.T.);
#16347=EDGE_CURVE('',#12483,#13003,#3245,.T.);
#16348=EDGE_CURVE('',#12717,#13003,#3246,.T.);
#16349=EDGE_CURVE('',#12888,#13004,#3247,.T.);
#16350=EDGE_CURVE('',#13004,#13005,#3248,.T.);
#16351=EDGE_CURVE('',#12889,#13005,#3249,.T.);
#16352=EDGE_CURVE('',#12453,#13004,#3250,.T.);
#16353=EDGE_CURVE('',#13005,#12452,#3251,.T.);
#16354=EDGE_CURVE('',#12718,#13006,#3252,.T.);
#16355=EDGE_CURVE('',#13006,#12488,#3253,.T.);
#16356=EDGE_CURVE('',#13007,#13006,#3254,.T.);
#16357=EDGE_CURVE('',#12489,#13007,#3255,.T.);
#16358=EDGE_CURVE('',#12719,#13007,#3256,.T.);
#16359=EDGE_CURVE('',#12447,#12887,#3257,.T.);
#16360=EDGE_CURVE('',#12720,#13008,#3258,.T.);
#16361=EDGE_CURVE('',#13008,#12494,#3259,.T.);
#16362=EDGE_CURVE('',#13009,#13008,#3260,.T.);
#16363=EDGE_CURVE('',#12495,#13009,#3261,.T.);
#16364=EDGE_CURVE('',#12721,#13009,#3262,.T.);
#16365=EDGE_CURVE('',#12882,#13010,#3263,.T.);
#16366=EDGE_CURVE('',#13010,#13011,#3264,.T.);
#16367=EDGE_CURVE('',#12883,#13011,#3265,.T.);
#16368=EDGE_CURVE('',#12441,#13010,#3266,.T.);
#16369=EDGE_CURVE('',#13011,#12440,#3267,.T.);
#16370=EDGE_CURVE('',#12722,#13012,#3268,.T.);
#16371=EDGE_CURVE('',#13012,#12500,#3269,.T.);
#16372=EDGE_CURVE('',#13013,#13012,#3270,.T.);
#16373=EDGE_CURVE('',#12501,#13013,#3271,.T.);
#16374=EDGE_CURVE('',#12723,#13013,#3272,.T.);
#16375=EDGE_CURVE('',#12435,#12881,#3273,.T.);
#16376=EDGE_CURVE('',#12724,#13014,#3274,.T.);
#16377=EDGE_CURVE('',#13014,#12506,#3275,.T.);
#16378=EDGE_CURVE('',#13015,#13014,#3276,.T.);
#16379=EDGE_CURVE('',#12507,#13015,#3277,.T.);
#16380=EDGE_CURVE('',#12725,#13015,#3278,.T.);
#16381=EDGE_CURVE('',#12876,#13016,#3279,.T.);
#16382=EDGE_CURVE('',#13016,#13017,#3280,.T.);
#16383=EDGE_CURVE('',#12877,#13017,#3281,.T.);
#16384=EDGE_CURVE('',#12429,#13016,#3282,.T.);
#16385=EDGE_CURVE('',#13017,#12428,#3283,.T.);
#16386=EDGE_CURVE('',#12726,#13018,#3284,.T.);
#16387=EDGE_CURVE('',#13018,#12512,#3285,.T.);
#16388=EDGE_CURVE('',#13019,#13018,#3286,.T.);
#16389=EDGE_CURVE('',#12513,#13019,#3287,.T.);
#16390=EDGE_CURVE('',#12727,#13019,#3288,.T.);
#16391=EDGE_CURVE('',#13020,#12422,#3289,.T.);
#16392=EDGE_CURVE('',#13021,#13020,#3290,.T.);
#16393=EDGE_CURVE('',#12423,#13021,#3291,.T.);
#16394=EDGE_CURVE('',#12808,#13021,#3292,.T.);
#16395=EDGE_CURVE('',#12809,#13020,#3293,.T.);
#20394=ORIENTED_EDGE('',*,*,#15201,.T.);
#20395=ORIENTED_EDGE('',*,*,#15202,.T.);
#20396=ORIENTED_EDGE('',*,*,#15203,.T.);
#20397=ORIENTED_EDGE('',*,*,#15204,.T.);
#20398=ORIENTED_EDGE('',*,*,#15202,.F.);
#20399=ORIENTED_EDGE('',*,*,#15205,.F.);
#20400=ORIENTED_EDGE('',*,*,#15206,.T.);
#20401=ORIENTED_EDGE('',*,*,#15207,.F.);
#20402=ORIENTED_EDGE('',*,*,#15201,.F.);
#20403=ORIENTED_EDGE('',*,*,#15208,.F.);
#20404=ORIENTED_EDGE('',*,*,#15209,.F.);
#20405=ORIENTED_EDGE('',*,*,#15210,.T.);
#20406=ORIENTED_EDGE('',*,*,#15211,.T.);
#20407=ORIENTED_EDGE('',*,*,#15212,.T.);
#20408=ORIENTED_EDGE('',*,*,#15213,.F.);
#20409=ORIENTED_EDGE('',*,*,#15214,.F.);
#20410=ORIENTED_EDGE('',*,*,#15215,.F.);
#20411=ORIENTED_EDGE('',*,*,#15216,.T.);
#20412=ORIENTED_EDGE('',*,*,#15217,.T.);
#20413=ORIENTED_EDGE('',*,*,#15218,.T.);
#20414=ORIENTED_EDGE('',*,*,#15219,.F.);
#20415=ORIENTED_EDGE('',*,*,#15220,.F.);
#20416=ORIENTED_EDGE('',*,*,#15221,.T.);
#20417=ORIENTED_EDGE('',*,*,#15222,.T.);
#20418=ORIENTED_EDGE('',*,*,#15223,.F.);
#20419=ORIENTED_EDGE('',*,*,#15224,.T.);
#20420=ORIENTED_EDGE('',*,*,#15225,.T.);
#20421=ORIENTED_EDGE('',*,*,#15226,.T.);
#20422=ORIENTED_EDGE('',*,*,#15227,.F.);
#20423=ORIENTED_EDGE('',*,*,#15228,.T.);
#20424=ORIENTED_EDGE('',*,*,#15229,.F.);
#20425=ORIENTED_EDGE('',*,*,#15230,.T.);
#20426=ORIENTED_EDGE('',*,*,#15231,.T.);
#20427=ORIENTED_EDGE('',*,*,#15232,.T.);
#20428=ORIENTED_EDGE('',*,*,#15233,.F.);
#20429=ORIENTED_EDGE('',*,*,#15234,.T.);
#20430=ORIENTED_EDGE('',*,*,#15235,.F.);
#20431=ORIENTED_EDGE('',*,*,#15236,.T.);
#20432=ORIENTED_EDGE('',*,*,#15237,.T.);
#20433=ORIENTED_EDGE('',*,*,#15238,.T.);
#20434=ORIENTED_EDGE('',*,*,#15239,.F.);
#20435=ORIENTED_EDGE('',*,*,#15240,.T.);
#20436=ORIENTED_EDGE('',*,*,#15241,.F.);
#20437=ORIENTED_EDGE('',*,*,#15242,.T.);
#20438=ORIENTED_EDGE('',*,*,#15243,.T.);
#20439=ORIENTED_EDGE('',*,*,#15244,.T.);
#20440=ORIENTED_EDGE('',*,*,#15245,.F.);
#20441=ORIENTED_EDGE('',*,*,#15246,.T.);
#20442=ORIENTED_EDGE('',*,*,#15247,.F.);
#20443=ORIENTED_EDGE('',*,*,#15248,.T.);
#20444=ORIENTED_EDGE('',*,*,#15249,.T.);
#20445=ORIENTED_EDGE('',*,*,#15250,.T.);
#20446=ORIENTED_EDGE('',*,*,#15251,.F.);
#20447=ORIENTED_EDGE('',*,*,#15252,.T.);
#20448=ORIENTED_EDGE('',*,*,#15253,.F.);
#20449=ORIENTED_EDGE('',*,*,#15254,.T.);
#20450=ORIENTED_EDGE('',*,*,#15255,.T.);
#20451=ORIENTED_EDGE('',*,*,#15256,.T.);
#20452=ORIENTED_EDGE('',*,*,#15257,.F.);
#20453=ORIENTED_EDGE('',*,*,#15258,.T.);
#20454=ORIENTED_EDGE('',*,*,#15259,.F.);
#20455=ORIENTED_EDGE('',*,*,#15260,.T.);
#20456=ORIENTED_EDGE('',*,*,#15261,.T.);
#20457=ORIENTED_EDGE('',*,*,#15262,.T.);
#20458=ORIENTED_EDGE('',*,*,#15263,.F.);
#20459=ORIENTED_EDGE('',*,*,#15264,.T.);
#20460=ORIENTED_EDGE('',*,*,#15265,.F.);
#20461=ORIENTED_EDGE('',*,*,#15266,.T.);
#20462=ORIENTED_EDGE('',*,*,#15267,.T.);
#20463=ORIENTED_EDGE('',*,*,#15268,.T.);
#20464=ORIENTED_EDGE('',*,*,#15269,.F.);
#20465=ORIENTED_EDGE('',*,*,#15270,.T.);
#20466=ORIENTED_EDGE('',*,*,#15271,.F.);
#20467=ORIENTED_EDGE('',*,*,#15272,.T.);
#20468=ORIENTED_EDGE('',*,*,#15273,.T.);
#20469=ORIENTED_EDGE('',*,*,#15274,.T.);
#20470=ORIENTED_EDGE('',*,*,#15275,.F.);
#20471=ORIENTED_EDGE('',*,*,#15276,.T.);
#20472=ORIENTED_EDGE('',*,*,#15277,.F.);
#20473=ORIENTED_EDGE('',*,*,#15278,.T.);
#20474=ORIENTED_EDGE('',*,*,#15279,.T.);
#20475=ORIENTED_EDGE('',*,*,#15280,.T.);
#20476=ORIENTED_EDGE('',*,*,#15281,.F.);
#20477=ORIENTED_EDGE('',*,*,#15282,.T.);
#20478=ORIENTED_EDGE('',*,*,#15283,.F.);
#20479=ORIENTED_EDGE('',*,*,#15284,.T.);
#20480=ORIENTED_EDGE('',*,*,#15285,.T.);
#20481=ORIENTED_EDGE('',*,*,#15286,.T.);
#20482=ORIENTED_EDGE('',*,*,#15287,.F.);
#20483=ORIENTED_EDGE('',*,*,#15288,.T.);
#20484=ORIENTED_EDGE('',*,*,#15289,.F.);
#20485=ORIENTED_EDGE('',*,*,#15290,.T.);
#20486=ORIENTED_EDGE('',*,*,#15291,.T.);
#20487=ORIENTED_EDGE('',*,*,#15292,.T.);
#20488=ORIENTED_EDGE('',*,*,#15293,.F.);
#20489=ORIENTED_EDGE('',*,*,#15294,.T.);
#20490=ORIENTED_EDGE('',*,*,#15295,.F.);
#20491=ORIENTED_EDGE('',*,*,#15296,.T.);
#20492=ORIENTED_EDGE('',*,*,#15297,.T.);
#20493=ORIENTED_EDGE('',*,*,#15298,.T.);
#20494=ORIENTED_EDGE('',*,*,#15299,.F.);
#20495=ORIENTED_EDGE('',*,*,#15300,.T.);
#20496=ORIENTED_EDGE('',*,*,#15301,.F.);
#20497=ORIENTED_EDGE('',*,*,#15302,.T.);
#20498=ORIENTED_EDGE('',*,*,#15303,.T.);
#20499=ORIENTED_EDGE('',*,*,#15304,.T.);
#20500=ORIENTED_EDGE('',*,*,#15305,.F.);
#20501=ORIENTED_EDGE('',*,*,#15306,.T.);
#20502=ORIENTED_EDGE('',*,*,#15307,.F.);
#20503=ORIENTED_EDGE('',*,*,#15308,.T.);
#20504=ORIENTED_EDGE('',*,*,#15309,.T.);
#20505=ORIENTED_EDGE('',*,*,#15310,.T.);
#20506=ORIENTED_EDGE('',*,*,#15311,.F.);
#20507=ORIENTED_EDGE('',*,*,#15312,.T.);
#20508=ORIENTED_EDGE('',*,*,#15313,.F.);
#20509=ORIENTED_EDGE('',*,*,#15314,.T.);
#20510=ORIENTED_EDGE('',*,*,#15315,.T.);
#20511=ORIENTED_EDGE('',*,*,#15316,.T.);
#20512=ORIENTED_EDGE('',*,*,#15317,.F.);
#20513=ORIENTED_EDGE('',*,*,#15318,.T.);
#20514=ORIENTED_EDGE('',*,*,#15319,.F.);
#20515=ORIENTED_EDGE('',*,*,#15320,.T.);
#20516=ORIENTED_EDGE('',*,*,#15321,.T.);
#20517=ORIENTED_EDGE('',*,*,#15322,.T.);
#20518=ORIENTED_EDGE('',*,*,#15323,.F.);
#20519=ORIENTED_EDGE('',*,*,#15324,.T.);
#20520=ORIENTED_EDGE('',*,*,#15325,.F.);
#20521=ORIENTED_EDGE('',*,*,#15326,.T.);
#20522=ORIENTED_EDGE('',*,*,#15327,.T.);
#20523=ORIENTED_EDGE('',*,*,#15328,.T.);
#20524=ORIENTED_EDGE('',*,*,#15329,.F.);
#20525=ORIENTED_EDGE('',*,*,#15330,.T.);
#20526=ORIENTED_EDGE('',*,*,#15331,.F.);
#20527=ORIENTED_EDGE('',*,*,#15332,.T.);
#20528=ORIENTED_EDGE('',*,*,#15333,.T.);
#20529=ORIENTED_EDGE('',*,*,#15334,.T.);
#20530=ORIENTED_EDGE('',*,*,#15335,.F.);
#20531=ORIENTED_EDGE('',*,*,#15336,.T.);
#20532=ORIENTED_EDGE('',*,*,#15337,.F.);
#20533=ORIENTED_EDGE('',*,*,#15338,.T.);
#20534=ORIENTED_EDGE('',*,*,#15339,.T.);
#20535=ORIENTED_EDGE('',*,*,#15340,.T.);
#20536=ORIENTED_EDGE('',*,*,#15341,.F.);
#20537=ORIENTED_EDGE('',*,*,#15342,.T.);
#20538=ORIENTED_EDGE('',*,*,#15343,.F.);
#20539=ORIENTED_EDGE('',*,*,#15344,.T.);
#20540=ORIENTED_EDGE('',*,*,#15345,.T.);
#20541=ORIENTED_EDGE('',*,*,#15346,.T.);
#20542=ORIENTED_EDGE('',*,*,#15347,.F.);
#20543=ORIENTED_EDGE('',*,*,#15348,.T.);
#20544=ORIENTED_EDGE('',*,*,#15349,.F.);
#20545=ORIENTED_EDGE('',*,*,#15350,.T.);
#20546=ORIENTED_EDGE('',*,*,#15351,.T.);
#20547=ORIENTED_EDGE('',*,*,#15352,.T.);
#20548=ORIENTED_EDGE('',*,*,#15353,.F.);
#20549=ORIENTED_EDGE('',*,*,#15354,.T.);
#20550=ORIENTED_EDGE('',*,*,#15355,.F.);
#20551=ORIENTED_EDGE('',*,*,#15356,.T.);
#20552=ORIENTED_EDGE('',*,*,#15357,.T.);
#20553=ORIENTED_EDGE('',*,*,#15358,.T.);
#20554=ORIENTED_EDGE('',*,*,#15359,.F.);
#20555=ORIENTED_EDGE('',*,*,#15360,.T.);
#20556=ORIENTED_EDGE('',*,*,#15361,.F.);
#20557=ORIENTED_EDGE('',*,*,#15362,.T.);
#20558=ORIENTED_EDGE('',*,*,#15363,.T.);
#20559=ORIENTED_EDGE('',*,*,#15364,.T.);
#20560=ORIENTED_EDGE('',*,*,#15365,.F.);
#20561=ORIENTED_EDGE('',*,*,#15366,.T.);
#20562=ORIENTED_EDGE('',*,*,#15367,.F.);
#20563=ORIENTED_EDGE('',*,*,#15368,.T.);
#20564=ORIENTED_EDGE('',*,*,#15369,.T.);
#20565=ORIENTED_EDGE('',*,*,#15370,.T.);
#20566=ORIENTED_EDGE('',*,*,#15371,.F.);
#20567=ORIENTED_EDGE('',*,*,#15372,.T.);
#20568=ORIENTED_EDGE('',*,*,#15373,.F.);
#20569=ORIENTED_EDGE('',*,*,#15374,.T.);
#20570=ORIENTED_EDGE('',*,*,#15375,.T.);
#20571=ORIENTED_EDGE('',*,*,#15376,.T.);
#20572=ORIENTED_EDGE('',*,*,#15377,.F.);
#20573=ORIENTED_EDGE('',*,*,#15378,.T.);
#20574=ORIENTED_EDGE('',*,*,#15379,.F.);
#20575=ORIENTED_EDGE('',*,*,#15380,.T.);
#20576=ORIENTED_EDGE('',*,*,#15381,.T.);
#20577=ORIENTED_EDGE('',*,*,#15382,.T.);
#20578=ORIENTED_EDGE('',*,*,#15383,.F.);
#20579=ORIENTED_EDGE('',*,*,#15384,.T.);
#20580=ORIENTED_EDGE('',*,*,#15385,.F.);
#20581=ORIENTED_EDGE('',*,*,#15386,.T.);
#20582=ORIENTED_EDGE('',*,*,#15387,.T.);
#20583=ORIENTED_EDGE('',*,*,#15388,.T.);
#20584=ORIENTED_EDGE('',*,*,#15389,.F.);
#20585=ORIENTED_EDGE('',*,*,#15390,.T.);
#20586=ORIENTED_EDGE('',*,*,#15391,.F.);
#20587=ORIENTED_EDGE('',*,*,#15392,.T.);
#20588=ORIENTED_EDGE('',*,*,#15393,.T.);
#20589=ORIENTED_EDGE('',*,*,#15394,.T.);
#20590=ORIENTED_EDGE('',*,*,#15395,.F.);
#20591=ORIENTED_EDGE('',*,*,#15396,.T.);
#20592=ORIENTED_EDGE('',*,*,#15397,.F.);
#20593=ORIENTED_EDGE('',*,*,#15398,.T.);
#20594=ORIENTED_EDGE('',*,*,#15399,.T.);
#20595=ORIENTED_EDGE('',*,*,#15400,.T.);
#20596=ORIENTED_EDGE('',*,*,#15401,.F.);
#20597=ORIENTED_EDGE('',*,*,#15402,.T.);
#20598=ORIENTED_EDGE('',*,*,#15221,.F.);
#20599=ORIENTED_EDGE('',*,*,#15403,.F.);
#20600=ORIENTED_EDGE('',*,*,#15404,.F.);
#20601=ORIENTED_EDGE('',*,*,#15405,.T.);
#20602=ORIENTED_EDGE('',*,*,#15406,.T.);
#20603=ORIENTED_EDGE('',*,*,#15407,.T.);
#20604=ORIENTED_EDGE('',*,*,#15408,.F.);
#20605=ORIENTED_EDGE('',*,*,#15409,.F.);
#20606=ORIENTED_EDGE('',*,*,#15410,.F.);
#20607=ORIENTED_EDGE('',*,*,#15411,.T.);
#20608=ORIENTED_EDGE('',*,*,#15412,.T.);
#20609=ORIENTED_EDGE('',*,*,#15413,.T.);
#20610=ORIENTED_EDGE('',*,*,#15414,.F.);
#20611=ORIENTED_EDGE('',*,*,#15415,.F.);
#20612=ORIENTED_EDGE('',*,*,#15416,.F.);
#20613=ORIENTED_EDGE('',*,*,#15417,.T.);
#20614=ORIENTED_EDGE('',*,*,#15418,.T.);
#20615=ORIENTED_EDGE('',*,*,#15419,.T.);
#20616=ORIENTED_EDGE('',*,*,#15420,.F.);
#20617=ORIENTED_EDGE('',*,*,#15421,.F.);
#20618=ORIENTED_EDGE('',*,*,#15422,.F.);
#20619=ORIENTED_EDGE('',*,*,#15423,.T.);
#20620=ORIENTED_EDGE('',*,*,#15424,.T.);
#20621=ORIENTED_EDGE('',*,*,#15425,.T.);
#20622=ORIENTED_EDGE('',*,*,#15426,.F.);
#20623=ORIENTED_EDGE('',*,*,#15427,.F.);
#20624=ORIENTED_EDGE('',*,*,#15428,.F.);
#20625=ORIENTED_EDGE('',*,*,#15429,.T.);
#20626=ORIENTED_EDGE('',*,*,#15430,.T.);
#20627=ORIENTED_EDGE('',*,*,#15431,.T.);
#20628=ORIENTED_EDGE('',*,*,#15432,.F.);
#20629=ORIENTED_EDGE('',*,*,#15433,.F.);
#20630=ORIENTED_EDGE('',*,*,#15434,.F.);
#20631=ORIENTED_EDGE('',*,*,#15435,.T.);
#20632=ORIENTED_EDGE('',*,*,#15436,.T.);
#20633=ORIENTED_EDGE('',*,*,#15437,.T.);
#20634=ORIENTED_EDGE('',*,*,#15438,.F.);
#20635=ORIENTED_EDGE('',*,*,#15439,.F.);
#20636=ORIENTED_EDGE('',*,*,#15440,.F.);
#20637=ORIENTED_EDGE('',*,*,#15441,.T.);
#20638=ORIENTED_EDGE('',*,*,#15442,.T.);
#20639=ORIENTED_EDGE('',*,*,#15443,.T.);
#20640=ORIENTED_EDGE('',*,*,#15444,.F.);
#20641=ORIENTED_EDGE('',*,*,#15445,.F.);
#20642=ORIENTED_EDGE('',*,*,#15446,.F.);
#20643=ORIENTED_EDGE('',*,*,#15447,.T.);
#20644=ORIENTED_EDGE('',*,*,#15448,.T.);
#20645=ORIENTED_EDGE('',*,*,#15449,.T.);
#20646=ORIENTED_EDGE('',*,*,#15450,.F.);
#20647=ORIENTED_EDGE('',*,*,#15451,.F.);
#20648=ORIENTED_EDGE('',*,*,#15452,.F.);
#20649=ORIENTED_EDGE('',*,*,#15453,.T.);
#20650=ORIENTED_EDGE('',*,*,#15454,.T.);
#20651=ORIENTED_EDGE('',*,*,#15455,.T.);
#20652=ORIENTED_EDGE('',*,*,#15456,.F.);
#20653=ORIENTED_EDGE('',*,*,#15457,.F.);
#20654=ORIENTED_EDGE('',*,*,#15458,.F.);
#20655=ORIENTED_EDGE('',*,*,#15459,.T.);
#20656=ORIENTED_EDGE('',*,*,#15460,.T.);
#20657=ORIENTED_EDGE('',*,*,#15461,.T.);
#20658=ORIENTED_EDGE('',*,*,#15462,.F.);
#20659=ORIENTED_EDGE('',*,*,#15463,.F.);
#20660=ORIENTED_EDGE('',*,*,#15464,.F.);
#20661=ORIENTED_EDGE('',*,*,#15465,.T.);
#20662=ORIENTED_EDGE('',*,*,#15466,.T.);
#20663=ORIENTED_EDGE('',*,*,#15467,.T.);
#20664=ORIENTED_EDGE('',*,*,#15468,.F.);
#20665=ORIENTED_EDGE('',*,*,#15469,.F.);
#20666=ORIENTED_EDGE('',*,*,#15470,.F.);
#20667=ORIENTED_EDGE('',*,*,#15471,.T.);
#20668=ORIENTED_EDGE('',*,*,#15472,.T.);
#20669=ORIENTED_EDGE('',*,*,#15473,.T.);
#20670=ORIENTED_EDGE('',*,*,#15474,.F.);
#20671=ORIENTED_EDGE('',*,*,#15475,.F.);
#20672=ORIENTED_EDGE('',*,*,#15476,.F.);
#20673=ORIENTED_EDGE('',*,*,#15477,.T.);
#20674=ORIENTED_EDGE('',*,*,#15478,.T.);
#20675=ORIENTED_EDGE('',*,*,#15479,.T.);
#20676=ORIENTED_EDGE('',*,*,#15480,.F.);
#20677=ORIENTED_EDGE('',*,*,#15481,.F.);
#20678=ORIENTED_EDGE('',*,*,#15482,.F.);
#20679=ORIENTED_EDGE('',*,*,#15483,.T.);
#20680=ORIENTED_EDGE('',*,*,#15484,.T.);
#20681=ORIENTED_EDGE('',*,*,#15485,.T.);
#20682=ORIENTED_EDGE('',*,*,#15486,.F.);
#20683=ORIENTED_EDGE('',*,*,#15487,.F.);
#20684=ORIENTED_EDGE('',*,*,#15488,.F.);
#20685=ORIENTED_EDGE('',*,*,#15489,.T.);
#20686=ORIENTED_EDGE('',*,*,#15490,.T.);
#20687=ORIENTED_EDGE('',*,*,#15491,.T.);
#20688=ORIENTED_EDGE('',*,*,#15492,.F.);
#20689=ORIENTED_EDGE('',*,*,#15493,.F.);
#20690=ORIENTED_EDGE('',*,*,#15494,.F.);
#20691=ORIENTED_EDGE('',*,*,#15495,.T.);
#20692=ORIENTED_EDGE('',*,*,#15496,.T.);
#20693=ORIENTED_EDGE('',*,*,#15497,.T.);
#20694=ORIENTED_EDGE('',*,*,#15498,.F.);
#20695=ORIENTED_EDGE('',*,*,#15499,.F.);
#20696=ORIENTED_EDGE('',*,*,#15500,.F.);
#20697=ORIENTED_EDGE('',*,*,#15501,.T.);
#20698=ORIENTED_EDGE('',*,*,#15502,.T.);
#20699=ORIENTED_EDGE('',*,*,#15503,.T.);
#20700=ORIENTED_EDGE('',*,*,#15504,.F.);
#20701=ORIENTED_EDGE('',*,*,#15505,.F.);
#20702=ORIENTED_EDGE('',*,*,#15506,.F.);
#20703=ORIENTED_EDGE('',*,*,#15507,.T.);
#20704=ORIENTED_EDGE('',*,*,#15508,.T.);
#20705=ORIENTED_EDGE('',*,*,#15509,.T.);
#20706=ORIENTED_EDGE('',*,*,#15510,.F.);
#20707=ORIENTED_EDGE('',*,*,#15511,.F.);
#20708=ORIENTED_EDGE('',*,*,#15512,.F.);
#20709=ORIENTED_EDGE('',*,*,#15513,.T.);
#20710=ORIENTED_EDGE('',*,*,#15514,.T.);
#20711=ORIENTED_EDGE('',*,*,#15515,.T.);
#20712=ORIENTED_EDGE('',*,*,#15516,.F.);
#20713=ORIENTED_EDGE('',*,*,#15517,.F.);
#20714=ORIENTED_EDGE('',*,*,#15518,.F.);
#20715=ORIENTED_EDGE('',*,*,#15519,.T.);
#20716=ORIENTED_EDGE('',*,*,#15520,.T.);
#20717=ORIENTED_EDGE('',*,*,#15521,.T.);
#20718=ORIENTED_EDGE('',*,*,#15522,.F.);
#20719=ORIENTED_EDGE('',*,*,#15523,.F.);
#20720=ORIENTED_EDGE('',*,*,#15524,.F.);
#20721=ORIENTED_EDGE('',*,*,#15525,.T.);
#20722=ORIENTED_EDGE('',*,*,#15526,.T.);
#20723=ORIENTED_EDGE('',*,*,#15527,.T.);
#20724=ORIENTED_EDGE('',*,*,#15528,.F.);
#20725=ORIENTED_EDGE('',*,*,#15529,.F.);
#20726=ORIENTED_EDGE('',*,*,#15530,.F.);
#20727=ORIENTED_EDGE('',*,*,#15531,.T.);
#20728=ORIENTED_EDGE('',*,*,#15532,.T.);
#20729=ORIENTED_EDGE('',*,*,#15533,.T.);
#20730=ORIENTED_EDGE('',*,*,#15534,.F.);
#20731=ORIENTED_EDGE('',*,*,#15535,.F.);
#20732=ORIENTED_EDGE('',*,*,#15536,.F.);
#20733=ORIENTED_EDGE('',*,*,#15537,.T.);
#20734=ORIENTED_EDGE('',*,*,#15538,.T.);
#20735=ORIENTED_EDGE('',*,*,#15539,.T.);
#20736=ORIENTED_EDGE('',*,*,#15540,.F.);
#20737=ORIENTED_EDGE('',*,*,#15541,.F.);
#20738=ORIENTED_EDGE('',*,*,#15542,.F.);
#20739=ORIENTED_EDGE('',*,*,#15543,.T.);
#20740=ORIENTED_EDGE('',*,*,#15544,.T.);
#20741=ORIENTED_EDGE('',*,*,#15545,.T.);
#20742=ORIENTED_EDGE('',*,*,#15546,.F.);
#20743=ORIENTED_EDGE('',*,*,#15547,.F.);
#20744=ORIENTED_EDGE('',*,*,#15548,.F.);
#20745=ORIENTED_EDGE('',*,*,#15549,.T.);
#20746=ORIENTED_EDGE('',*,*,#15550,.T.);
#20747=ORIENTED_EDGE('',*,*,#15551,.T.);
#20748=ORIENTED_EDGE('',*,*,#15552,.F.);
#20749=ORIENTED_EDGE('',*,*,#15553,.F.);
#20750=ORIENTED_EDGE('',*,*,#15554,.F.);
#20751=ORIENTED_EDGE('',*,*,#15555,.T.);
#20752=ORIENTED_EDGE('',*,*,#15556,.T.);
#20753=ORIENTED_EDGE('',*,*,#15557,.T.);
#20754=ORIENTED_EDGE('',*,*,#15558,.F.);
#20755=ORIENTED_EDGE('',*,*,#15559,.F.);
#20756=ORIENTED_EDGE('',*,*,#15560,.F.);
#20757=ORIENTED_EDGE('',*,*,#15561,.T.);
#20758=ORIENTED_EDGE('',*,*,#15562,.T.);
#20759=ORIENTED_EDGE('',*,*,#15563,.T.);
#20760=ORIENTED_EDGE('',*,*,#15564,.F.);
#20761=ORIENTED_EDGE('',*,*,#15565,.F.);
#20762=ORIENTED_EDGE('',*,*,#15566,.F.);
#20763=ORIENTED_EDGE('',*,*,#15567,.T.);
#20764=ORIENTED_EDGE('',*,*,#15568,.T.);
#20765=ORIENTED_EDGE('',*,*,#15205,.T.);
#20766=ORIENTED_EDGE('',*,*,#15569,.T.);
#20767=ORIENTED_EDGE('',*,*,#15209,.T.);
#20768=ORIENTED_EDGE('',*,*,#15570,.T.);
#20769=ORIENTED_EDGE('',*,*,#15571,.T.);
#20770=ORIENTED_EDGE('',*,*,#15572,.T.);
#20771=ORIENTED_EDGE('',*,*,#15573,.T.);
#20772=ORIENTED_EDGE('',*,*,#15574,.T.);
#20773=ORIENTED_EDGE('',*,*,#15571,.F.);
#20774=ORIENTED_EDGE('',*,*,#15575,.T.);
#20775=ORIENTED_EDGE('',*,*,#15213,.T.);
#20776=ORIENTED_EDGE('',*,*,#15576,.T.);
#20777=ORIENTED_EDGE('',*,*,#15573,.F.);
#20778=ORIENTED_EDGE('',*,*,#15569,.F.);
#20779=ORIENTED_EDGE('',*,*,#15577,.T.);
#20780=ORIENTED_EDGE('',*,*,#15578,.T.);
#20781=ORIENTED_EDGE('',*,*,#15210,.F.);
#20782=ORIENTED_EDGE('',*,*,#15574,.F.);
#20783=ORIENTED_EDGE('',*,*,#15579,.T.);
#20784=ORIENTED_EDGE('',*,*,#15580,.T.);
#20785=ORIENTED_EDGE('',*,*,#15577,.F.);
#20786=ORIENTED_EDGE('',*,*,#15576,.F.);
#20787=ORIENTED_EDGE('',*,*,#15212,.F.);
#20788=ORIENTED_EDGE('',*,*,#15581,.T.);
#20789=ORIENTED_EDGE('',*,*,#15579,.F.);
#20790=ORIENTED_EDGE('',*,*,#15582,.T.);
#20791=ORIENTED_EDGE('',*,*,#15215,.T.);
#20792=ORIENTED_EDGE('',*,*,#15583,.T.);
#20793=ORIENTED_EDGE('',*,*,#15584,.T.);
#20794=ORIENTED_EDGE('',*,*,#15585,.T.);
#20795=ORIENTED_EDGE('',*,*,#15586,.T.);
#20796=ORIENTED_EDGE('',*,*,#15587,.T.);
#20797=ORIENTED_EDGE('',*,*,#15584,.F.);
#20798=ORIENTED_EDGE('',*,*,#15588,.T.);
#20799=ORIENTED_EDGE('',*,*,#15219,.T.);
#20800=ORIENTED_EDGE('',*,*,#15589,.T.);
#20801=ORIENTED_EDGE('',*,*,#15586,.F.);
#20802=ORIENTED_EDGE('',*,*,#15582,.F.);
#20803=ORIENTED_EDGE('',*,*,#15590,.T.);
#20804=ORIENTED_EDGE('',*,*,#15591,.T.);
#20805=ORIENTED_EDGE('',*,*,#15216,.F.);
#20806=ORIENTED_EDGE('',*,*,#15587,.F.);
#20807=ORIENTED_EDGE('',*,*,#15592,.T.);
#20808=ORIENTED_EDGE('',*,*,#15593,.T.);
#20809=ORIENTED_EDGE('',*,*,#15590,.F.);
#20810=ORIENTED_EDGE('',*,*,#15589,.F.);
#20811=ORIENTED_EDGE('',*,*,#15218,.F.);
#20812=ORIENTED_EDGE('',*,*,#15594,.T.);
#20813=ORIENTED_EDGE('',*,*,#15592,.F.);
#20814=ORIENTED_EDGE('',*,*,#15595,.T.);
#20815=ORIENTED_EDGE('',*,*,#15404,.T.);
#20816=ORIENTED_EDGE('',*,*,#15596,.T.);
#20817=ORIENTED_EDGE('',*,*,#15597,.T.);
#20818=ORIENTED_EDGE('',*,*,#15598,.T.);
#20819=ORIENTED_EDGE('',*,*,#15599,.T.);
#20820=ORIENTED_EDGE('',*,*,#15600,.T.);
#20821=ORIENTED_EDGE('',*,*,#15597,.F.);
#20822=ORIENTED_EDGE('',*,*,#15601,.T.);
#20823=ORIENTED_EDGE('',*,*,#15408,.T.);
#20824=ORIENTED_EDGE('',*,*,#15602,.T.);
#20825=ORIENTED_EDGE('',*,*,#15599,.F.);
#20826=ORIENTED_EDGE('',*,*,#15595,.F.);
#20827=ORIENTED_EDGE('',*,*,#15603,.T.);
#20828=ORIENTED_EDGE('',*,*,#15604,.T.);
#20829=ORIENTED_EDGE('',*,*,#15405,.F.);
#20830=ORIENTED_EDGE('',*,*,#15600,.F.);
#20831=ORIENTED_EDGE('',*,*,#15605,.T.);
#20832=ORIENTED_EDGE('',*,*,#15606,.T.);
#20833=ORIENTED_EDGE('',*,*,#15603,.F.);
#20834=ORIENTED_EDGE('',*,*,#15602,.F.);
#20835=ORIENTED_EDGE('',*,*,#15407,.F.);
#20836=ORIENTED_EDGE('',*,*,#15607,.T.);
#20837=ORIENTED_EDGE('',*,*,#15605,.F.);
#20838=ORIENTED_EDGE('',*,*,#15608,.T.);
#20839=ORIENTED_EDGE('',*,*,#15410,.T.);
#20840=ORIENTED_EDGE('',*,*,#15609,.T.);
#20841=ORIENTED_EDGE('',*,*,#15610,.T.);
#20842=ORIENTED_EDGE('',*,*,#15611,.T.);
#20843=ORIENTED_EDGE('',*,*,#15612,.T.);
#20844=ORIENTED_EDGE('',*,*,#15613,.T.);
#20845=ORIENTED_EDGE('',*,*,#15610,.F.);
#20846=ORIENTED_EDGE('',*,*,#15608,.F.);
#20847=ORIENTED_EDGE('',*,*,#15614,.T.);
#20848=ORIENTED_EDGE('',*,*,#15615,.T.);
#20849=ORIENTED_EDGE('',*,*,#15411,.F.);
#20850=ORIENTED_EDGE('',*,*,#15613,.F.);
#20851=ORIENTED_EDGE('',*,*,#15616,.T.);
#20852=ORIENTED_EDGE('',*,*,#15617,.T.);
#20853=ORIENTED_EDGE('',*,*,#15614,.F.);
#20854=ORIENTED_EDGE('',*,*,#15414,.T.);
#20855=ORIENTED_EDGE('',*,*,#15618,.T.);
#20856=ORIENTED_EDGE('',*,*,#15612,.F.);
#20857=ORIENTED_EDGE('',*,*,#15619,.T.);
#20858=ORIENTED_EDGE('',*,*,#15620,.F.);
#20859=ORIENTED_EDGE('',*,*,#15621,.F.);
#20860=ORIENTED_EDGE('',*,*,#15565,.T.);
#20861=ORIENTED_EDGE('',*,*,#15622,.F.);
#20862=ORIENTED_EDGE('',*,*,#15623,.F.);
#20863=ORIENTED_EDGE('',*,*,#15624,.F.);
#20864=ORIENTED_EDGE('',*,*,#15559,.T.);
#20865=ORIENTED_EDGE('',*,*,#15625,.F.);
#20866=ORIENTED_EDGE('',*,*,#15626,.F.);
#20867=ORIENTED_EDGE('',*,*,#15627,.F.);
#20868=ORIENTED_EDGE('',*,*,#15553,.T.);
#20869=ORIENTED_EDGE('',*,*,#15628,.F.);
#20870=ORIENTED_EDGE('',*,*,#15629,.F.);
#20871=ORIENTED_EDGE('',*,*,#15630,.F.);
#20872=ORIENTED_EDGE('',*,*,#15547,.T.);
#20873=ORIENTED_EDGE('',*,*,#15631,.F.);
#20874=ORIENTED_EDGE('',*,*,#15632,.F.);
#20875=ORIENTED_EDGE('',*,*,#15633,.F.);
#20876=ORIENTED_EDGE('',*,*,#15541,.T.);
#20877=ORIENTED_EDGE('',*,*,#15634,.F.);
#20878=ORIENTED_EDGE('',*,*,#15635,.F.);
#20879=ORIENTED_EDGE('',*,*,#15636,.F.);
#20880=ORIENTED_EDGE('',*,*,#15535,.T.);
#20881=ORIENTED_EDGE('',*,*,#15637,.F.);
#20882=ORIENTED_EDGE('',*,*,#15638,.F.);
#20883=ORIENTED_EDGE('',*,*,#15639,.F.);
#20884=ORIENTED_EDGE('',*,*,#15529,.T.);
#20885=ORIENTED_EDGE('',*,*,#15640,.F.);
#20886=ORIENTED_EDGE('',*,*,#15641,.F.);
#20887=ORIENTED_EDGE('',*,*,#15642,.F.);
#20888=ORIENTED_EDGE('',*,*,#15523,.T.);
#20889=ORIENTED_EDGE('',*,*,#15643,.F.);
#20890=ORIENTED_EDGE('',*,*,#15644,.F.);
#20891=ORIENTED_EDGE('',*,*,#15645,.F.);
#20892=ORIENTED_EDGE('',*,*,#15517,.T.);
#20893=ORIENTED_EDGE('',*,*,#15646,.F.);
#20894=ORIENTED_EDGE('',*,*,#15647,.F.);
#20895=ORIENTED_EDGE('',*,*,#15648,.F.);
#20896=ORIENTED_EDGE('',*,*,#15511,.T.);
#20897=ORIENTED_EDGE('',*,*,#15649,.F.);
#20898=ORIENTED_EDGE('',*,*,#15650,.F.);
#20899=ORIENTED_EDGE('',*,*,#15651,.F.);
#20900=ORIENTED_EDGE('',*,*,#15505,.T.);
#20901=ORIENTED_EDGE('',*,*,#15652,.F.);
#20902=ORIENTED_EDGE('',*,*,#15653,.F.);
#20903=ORIENTED_EDGE('',*,*,#15654,.F.);
#20904=ORIENTED_EDGE('',*,*,#15499,.T.);
#20905=ORIENTED_EDGE('',*,*,#15655,.F.);
#20906=ORIENTED_EDGE('',*,*,#15656,.F.);
#20907=ORIENTED_EDGE('',*,*,#15657,.F.);
#20908=ORIENTED_EDGE('',*,*,#15493,.T.);
#20909=ORIENTED_EDGE('',*,*,#15658,.F.);
#20910=ORIENTED_EDGE('',*,*,#15659,.F.);
#20911=ORIENTED_EDGE('',*,*,#15660,.F.);
#20912=ORIENTED_EDGE('',*,*,#15487,.T.);
#20913=ORIENTED_EDGE('',*,*,#15661,.F.);
#20914=ORIENTED_EDGE('',*,*,#15662,.F.);
#20915=ORIENTED_EDGE('',*,*,#15663,.F.);
#20916=ORIENTED_EDGE('',*,*,#15481,.T.);
#20917=ORIENTED_EDGE('',*,*,#15664,.F.);
#20918=ORIENTED_EDGE('',*,*,#15665,.F.);
#20919=ORIENTED_EDGE('',*,*,#15666,.F.);
#20920=ORIENTED_EDGE('',*,*,#15475,.T.);
#20921=ORIENTED_EDGE('',*,*,#15667,.F.);
#20922=ORIENTED_EDGE('',*,*,#15668,.F.);
#20923=ORIENTED_EDGE('',*,*,#15669,.F.);
#20924=ORIENTED_EDGE('',*,*,#15469,.T.);
#20925=ORIENTED_EDGE('',*,*,#15670,.F.);
#20926=ORIENTED_EDGE('',*,*,#15671,.F.);
#20927=ORIENTED_EDGE('',*,*,#15672,.F.);
#20928=ORIENTED_EDGE('',*,*,#15463,.T.);
#20929=ORIENTED_EDGE('',*,*,#15673,.F.);
#20930=ORIENTED_EDGE('',*,*,#15674,.F.);
#20931=ORIENTED_EDGE('',*,*,#15675,.F.);
#20932=ORIENTED_EDGE('',*,*,#15457,.T.);
#20933=ORIENTED_EDGE('',*,*,#15676,.F.);
#20934=ORIENTED_EDGE('',*,*,#15677,.F.);
#20935=ORIENTED_EDGE('',*,*,#15678,.F.);
#20936=ORIENTED_EDGE('',*,*,#15451,.T.);
#20937=ORIENTED_EDGE('',*,*,#15679,.F.);
#20938=ORIENTED_EDGE('',*,*,#15680,.F.);
#20939=ORIENTED_EDGE('',*,*,#15681,.F.);
#20940=ORIENTED_EDGE('',*,*,#15445,.T.);
#20941=ORIENTED_EDGE('',*,*,#15682,.F.);
#20942=ORIENTED_EDGE('',*,*,#15683,.F.);
#20943=ORIENTED_EDGE('',*,*,#15684,.F.);
#20944=ORIENTED_EDGE('',*,*,#15439,.T.);
#20945=ORIENTED_EDGE('',*,*,#15685,.F.);
#20946=ORIENTED_EDGE('',*,*,#15686,.F.);
#20947=ORIENTED_EDGE('',*,*,#15687,.F.);
#20948=ORIENTED_EDGE('',*,*,#15433,.T.);
#20949=ORIENTED_EDGE('',*,*,#15688,.F.);
#20950=ORIENTED_EDGE('',*,*,#15689,.F.);
#20951=ORIENTED_EDGE('',*,*,#15690,.F.);
#20952=ORIENTED_EDGE('',*,*,#15427,.T.);
#20953=ORIENTED_EDGE('',*,*,#15691,.F.);
#20954=ORIENTED_EDGE('',*,*,#15692,.F.);
#20955=ORIENTED_EDGE('',*,*,#15693,.F.);
#20956=ORIENTED_EDGE('',*,*,#15421,.T.);
#20957=ORIENTED_EDGE('',*,*,#15694,.F.);
#20958=ORIENTED_EDGE('',*,*,#15695,.F.);
#20959=ORIENTED_EDGE('',*,*,#15696,.F.);
#20960=ORIENTED_EDGE('',*,*,#15415,.T.);
#20961=ORIENTED_EDGE('',*,*,#15619,.F.);
#20962=ORIENTED_EDGE('',*,*,#15611,.F.);
#20963=ORIENTED_EDGE('',*,*,#15609,.F.);
#20964=ORIENTED_EDGE('',*,*,#15409,.T.);
#20965=ORIENTED_EDGE('',*,*,#15601,.F.);
#20966=ORIENTED_EDGE('',*,*,#15598,.F.);
#20967=ORIENTED_EDGE('',*,*,#15596,.F.);
#20968=ORIENTED_EDGE('',*,*,#15403,.T.);
#20969=ORIENTED_EDGE('',*,*,#15220,.T.);
#20970=ORIENTED_EDGE('',*,*,#15588,.F.);
#20971=ORIENTED_EDGE('',*,*,#15585,.F.);
#20972=ORIENTED_EDGE('',*,*,#15583,.F.);
#20973=ORIENTED_EDGE('',*,*,#15214,.T.);
#20974=ORIENTED_EDGE('',*,*,#15575,.F.);
#20975=ORIENTED_EDGE('',*,*,#15572,.F.);
#20976=ORIENTED_EDGE('',*,*,#15570,.F.);
#20977=ORIENTED_EDGE('',*,*,#15208,.T.);
#20978=ORIENTED_EDGE('',*,*,#15204,.F.);
#20979=ORIENTED_EDGE('',*,*,#15697,.F.);
#20980=ORIENTED_EDGE('',*,*,#15698,.F.);
#20981=ORIENTED_EDGE('',*,*,#15699,.F.);
#20982=ORIENTED_EDGE('',*,*,#15700,.F.);
#20983=ORIENTED_EDGE('',*,*,#15701,.F.);
#20984=ORIENTED_EDGE('',*,*,#15702,.F.);
#20985=ORIENTED_EDGE('',*,*,#15703,.F.);
#20986=ORIENTED_EDGE('',*,*,#15704,.F.);
#20987=ORIENTED_EDGE('',*,*,#15705,.T.);
#20988=ORIENTED_EDGE('',*,*,#15416,.T.);
#20989=ORIENTED_EDGE('',*,*,#15696,.T.);
#20990=ORIENTED_EDGE('',*,*,#15706,.T.);
#20991=ORIENTED_EDGE('',*,*,#15695,.T.);
#20992=ORIENTED_EDGE('',*,*,#15707,.T.);
#20993=ORIENTED_EDGE('',*,*,#15708,.T.);
#20994=ORIENTED_EDGE('',*,*,#15706,.F.);
#20995=ORIENTED_EDGE('',*,*,#15694,.T.);
#20996=ORIENTED_EDGE('',*,*,#15420,.T.);
#20997=ORIENTED_EDGE('',*,*,#15709,.T.);
#20998=ORIENTED_EDGE('',*,*,#15707,.F.);
#20999=ORIENTED_EDGE('',*,*,#15710,.T.);
#21000=ORIENTED_EDGE('',*,*,#15422,.T.);
#21001=ORIENTED_EDGE('',*,*,#15693,.T.);
#21002=ORIENTED_EDGE('',*,*,#15711,.T.);
#21003=ORIENTED_EDGE('',*,*,#15692,.T.);
#21004=ORIENTED_EDGE('',*,*,#15712,.T.);
#21005=ORIENTED_EDGE('',*,*,#15713,.T.);
#21006=ORIENTED_EDGE('',*,*,#15711,.F.);
#21007=ORIENTED_EDGE('',*,*,#15691,.T.);
#21008=ORIENTED_EDGE('',*,*,#15426,.T.);
#21009=ORIENTED_EDGE('',*,*,#15714,.T.);
#21010=ORIENTED_EDGE('',*,*,#15712,.F.);
#21011=ORIENTED_EDGE('',*,*,#15715,.T.);
#21012=ORIENTED_EDGE('',*,*,#15428,.T.);
#21013=ORIENTED_EDGE('',*,*,#15690,.T.);
#21014=ORIENTED_EDGE('',*,*,#15716,.T.);
#21015=ORIENTED_EDGE('',*,*,#15689,.T.);
#21016=ORIENTED_EDGE('',*,*,#15717,.T.);
#21017=ORIENTED_EDGE('',*,*,#15718,.T.);
#21018=ORIENTED_EDGE('',*,*,#15716,.F.);
#21019=ORIENTED_EDGE('',*,*,#15688,.T.);
#21020=ORIENTED_EDGE('',*,*,#15432,.T.);
#21021=ORIENTED_EDGE('',*,*,#15719,.T.);
#21022=ORIENTED_EDGE('',*,*,#15717,.F.);
#21023=ORIENTED_EDGE('',*,*,#15720,.T.);
#21024=ORIENTED_EDGE('',*,*,#15434,.T.);
#21025=ORIENTED_EDGE('',*,*,#15687,.T.);
#21026=ORIENTED_EDGE('',*,*,#15721,.T.);
#21027=ORIENTED_EDGE('',*,*,#15686,.T.);
#21028=ORIENTED_EDGE('',*,*,#15722,.T.);
#21029=ORIENTED_EDGE('',*,*,#15723,.T.);
#21030=ORIENTED_EDGE('',*,*,#15721,.F.);
#21031=ORIENTED_EDGE('',*,*,#15685,.T.);
#21032=ORIENTED_EDGE('',*,*,#15438,.T.);
#21033=ORIENTED_EDGE('',*,*,#15724,.T.);
#21034=ORIENTED_EDGE('',*,*,#15722,.F.);
#21035=ORIENTED_EDGE('',*,*,#15725,.T.);
#21036=ORIENTED_EDGE('',*,*,#15440,.T.);
#21037=ORIENTED_EDGE('',*,*,#15684,.T.);
#21038=ORIENTED_EDGE('',*,*,#15726,.T.);
#21039=ORIENTED_EDGE('',*,*,#15683,.T.);
#21040=ORIENTED_EDGE('',*,*,#15727,.T.);
#21041=ORIENTED_EDGE('',*,*,#15728,.T.);
#21042=ORIENTED_EDGE('',*,*,#15726,.F.);
#21043=ORIENTED_EDGE('',*,*,#15682,.T.);
#21044=ORIENTED_EDGE('',*,*,#15444,.T.);
#21045=ORIENTED_EDGE('',*,*,#15729,.T.);
#21046=ORIENTED_EDGE('',*,*,#15727,.F.);
#21047=ORIENTED_EDGE('',*,*,#15730,.T.);
#21048=ORIENTED_EDGE('',*,*,#15446,.T.);
#21049=ORIENTED_EDGE('',*,*,#15681,.T.);
#21050=ORIENTED_EDGE('',*,*,#15731,.T.);
#21051=ORIENTED_EDGE('',*,*,#15680,.T.);
#21052=ORIENTED_EDGE('',*,*,#15732,.T.);
#21053=ORIENTED_EDGE('',*,*,#15733,.T.);
#21054=ORIENTED_EDGE('',*,*,#15731,.F.);
#21055=ORIENTED_EDGE('',*,*,#15679,.T.);
#21056=ORIENTED_EDGE('',*,*,#15450,.T.);
#21057=ORIENTED_EDGE('',*,*,#15734,.T.);
#21058=ORIENTED_EDGE('',*,*,#15732,.F.);
#21059=ORIENTED_EDGE('',*,*,#15735,.T.);
#21060=ORIENTED_EDGE('',*,*,#15736,.T.);
#21061=ORIENTED_EDGE('',*,*,#15620,.T.);
#21062=ORIENTED_EDGE('',*,*,#15203,.F.);
#21063=ORIENTED_EDGE('',*,*,#15735,.F.);
#21064=ORIENTED_EDGE('',*,*,#15207,.T.);
#21065=ORIENTED_EDGE('',*,*,#15737,.T.);
#21066=ORIENTED_EDGE('',*,*,#15738,.F.);
#21067=ORIENTED_EDGE('',*,*,#15566,.T.);
#21068=ORIENTED_EDGE('',*,*,#15621,.T.);
#21069=ORIENTED_EDGE('',*,*,#15736,.F.);
#21070=ORIENTED_EDGE('',*,*,#15739,.T.);
#21071=ORIENTED_EDGE('',*,*,#15740,.T.);
#21072=ORIENTED_EDGE('',*,*,#15560,.T.);
#21073=ORIENTED_EDGE('',*,*,#15624,.T.);
#21074=ORIENTED_EDGE('',*,*,#15741,.T.);
#21075=ORIENTED_EDGE('',*,*,#15742,.T.);
#21076=ORIENTED_EDGE('',*,*,#15741,.F.);
#21077=ORIENTED_EDGE('',*,*,#15623,.T.);
#21078=ORIENTED_EDGE('',*,*,#15743,.T.);
#21079=ORIENTED_EDGE('',*,*,#15622,.T.);
#21080=ORIENTED_EDGE('',*,*,#15564,.T.);
#21081=ORIENTED_EDGE('',*,*,#15744,.T.);
#21082=ORIENTED_EDGE('',*,*,#15743,.F.);
#21083=ORIENTED_EDGE('',*,*,#15740,.F.);
#21084=ORIENTED_EDGE('',*,*,#15745,.T.);
#21085=ORIENTED_EDGE('',*,*,#15746,.T.);
#21086=ORIENTED_EDGE('',*,*,#15561,.F.);
#21087=ORIENTED_EDGE('',*,*,#15742,.F.);
#21088=ORIENTED_EDGE('',*,*,#15747,.T.);
#21089=ORIENTED_EDGE('',*,*,#15748,.T.);
#21090=ORIENTED_EDGE('',*,*,#15745,.F.);
#21091=ORIENTED_EDGE('',*,*,#15744,.F.);
#21092=ORIENTED_EDGE('',*,*,#15563,.F.);
#21093=ORIENTED_EDGE('',*,*,#15749,.T.);
#21094=ORIENTED_EDGE('',*,*,#15747,.F.);
#21095=ORIENTED_EDGE('',*,*,#15750,.T.);
#21096=ORIENTED_EDGE('',*,*,#15554,.T.);
#21097=ORIENTED_EDGE('',*,*,#15627,.T.);
#21098=ORIENTED_EDGE('',*,*,#15751,.T.);
#21099=ORIENTED_EDGE('',*,*,#15752,.T.);
#21100=ORIENTED_EDGE('',*,*,#15751,.F.);
#21101=ORIENTED_EDGE('',*,*,#15626,.T.);
#21102=ORIENTED_EDGE('',*,*,#15753,.T.);
#21103=ORIENTED_EDGE('',*,*,#15625,.T.);
#21104=ORIENTED_EDGE('',*,*,#15558,.T.);
#21105=ORIENTED_EDGE('',*,*,#15754,.T.);
#21106=ORIENTED_EDGE('',*,*,#15753,.F.);
#21107=ORIENTED_EDGE('',*,*,#15750,.F.);
#21108=ORIENTED_EDGE('',*,*,#15755,.T.);
#21109=ORIENTED_EDGE('',*,*,#15756,.T.);
#21110=ORIENTED_EDGE('',*,*,#15555,.F.);
#21111=ORIENTED_EDGE('',*,*,#15752,.F.);
#21112=ORIENTED_EDGE('',*,*,#15757,.T.);
#21113=ORIENTED_EDGE('',*,*,#15758,.T.);
#21114=ORIENTED_EDGE('',*,*,#15755,.F.);
#21115=ORIENTED_EDGE('',*,*,#15754,.F.);
#21116=ORIENTED_EDGE('',*,*,#15557,.F.);
#21117=ORIENTED_EDGE('',*,*,#15759,.T.);
#21118=ORIENTED_EDGE('',*,*,#15757,.F.);
#21119=ORIENTED_EDGE('',*,*,#15760,.T.);
#21120=ORIENTED_EDGE('',*,*,#15548,.T.);
#21121=ORIENTED_EDGE('',*,*,#15630,.T.);
#21122=ORIENTED_EDGE('',*,*,#15761,.T.);
#21123=ORIENTED_EDGE('',*,*,#15762,.T.);
#21124=ORIENTED_EDGE('',*,*,#15761,.F.);
#21125=ORIENTED_EDGE('',*,*,#15629,.T.);
#21126=ORIENTED_EDGE('',*,*,#15763,.T.);
#21127=ORIENTED_EDGE('',*,*,#15628,.T.);
#21128=ORIENTED_EDGE('',*,*,#15552,.T.);
#21129=ORIENTED_EDGE('',*,*,#15764,.T.);
#21130=ORIENTED_EDGE('',*,*,#15763,.F.);
#21131=ORIENTED_EDGE('',*,*,#15760,.F.);
#21132=ORIENTED_EDGE('',*,*,#15765,.T.);
#21133=ORIENTED_EDGE('',*,*,#15766,.T.);
#21134=ORIENTED_EDGE('',*,*,#15549,.F.);
#21135=ORIENTED_EDGE('',*,*,#15762,.F.);
#21136=ORIENTED_EDGE('',*,*,#15767,.T.);
#21137=ORIENTED_EDGE('',*,*,#15768,.T.);
#21138=ORIENTED_EDGE('',*,*,#15765,.F.);
#21139=ORIENTED_EDGE('',*,*,#15764,.F.);
#21140=ORIENTED_EDGE('',*,*,#15551,.F.);
#21141=ORIENTED_EDGE('',*,*,#15769,.T.);
#21142=ORIENTED_EDGE('',*,*,#15767,.F.);
#21143=ORIENTED_EDGE('',*,*,#15770,.T.);
#21144=ORIENTED_EDGE('',*,*,#15542,.T.);
#21145=ORIENTED_EDGE('',*,*,#15633,.T.);
#21146=ORIENTED_EDGE('',*,*,#15771,.T.);
#21147=ORIENTED_EDGE('',*,*,#15772,.T.);
#21148=ORIENTED_EDGE('',*,*,#15771,.F.);
#21149=ORIENTED_EDGE('',*,*,#15632,.T.);
#21150=ORIENTED_EDGE('',*,*,#15773,.T.);
#21151=ORIENTED_EDGE('',*,*,#15631,.T.);
#21152=ORIENTED_EDGE('',*,*,#15546,.T.);
#21153=ORIENTED_EDGE('',*,*,#15774,.T.);
#21154=ORIENTED_EDGE('',*,*,#15773,.F.);
#21155=ORIENTED_EDGE('',*,*,#15770,.F.);
#21156=ORIENTED_EDGE('',*,*,#15775,.T.);
#21157=ORIENTED_EDGE('',*,*,#15776,.T.);
#21158=ORIENTED_EDGE('',*,*,#15543,.F.);
#21159=ORIENTED_EDGE('',*,*,#15772,.F.);
#21160=ORIENTED_EDGE('',*,*,#15777,.T.);
#21161=ORIENTED_EDGE('',*,*,#15778,.T.);
#21162=ORIENTED_EDGE('',*,*,#15775,.F.);
#21163=ORIENTED_EDGE('',*,*,#15774,.F.);
#21164=ORIENTED_EDGE('',*,*,#15545,.F.);
#21165=ORIENTED_EDGE('',*,*,#15779,.T.);
#21166=ORIENTED_EDGE('',*,*,#15777,.F.);
#21167=ORIENTED_EDGE('',*,*,#15780,.T.);
#21168=ORIENTED_EDGE('',*,*,#15536,.T.);
#21169=ORIENTED_EDGE('',*,*,#15636,.T.);
#21170=ORIENTED_EDGE('',*,*,#15781,.T.);
#21171=ORIENTED_EDGE('',*,*,#15782,.T.);
#21172=ORIENTED_EDGE('',*,*,#15781,.F.);
#21173=ORIENTED_EDGE('',*,*,#15635,.T.);
#21174=ORIENTED_EDGE('',*,*,#15783,.T.);
#21175=ORIENTED_EDGE('',*,*,#15634,.T.);
#21176=ORIENTED_EDGE('',*,*,#15540,.T.);
#21177=ORIENTED_EDGE('',*,*,#15784,.T.);
#21178=ORIENTED_EDGE('',*,*,#15783,.F.);
#21179=ORIENTED_EDGE('',*,*,#15780,.F.);
#21180=ORIENTED_EDGE('',*,*,#15785,.T.);
#21181=ORIENTED_EDGE('',*,*,#15786,.T.);
#21182=ORIENTED_EDGE('',*,*,#15537,.F.);
#21183=ORIENTED_EDGE('',*,*,#15782,.F.);
#21184=ORIENTED_EDGE('',*,*,#15787,.T.);
#21185=ORIENTED_EDGE('',*,*,#15788,.T.);
#21186=ORIENTED_EDGE('',*,*,#15785,.F.);
#21187=ORIENTED_EDGE('',*,*,#15784,.F.);
#21188=ORIENTED_EDGE('',*,*,#15539,.F.);
#21189=ORIENTED_EDGE('',*,*,#15789,.T.);
#21190=ORIENTED_EDGE('',*,*,#15787,.F.);
#21191=ORIENTED_EDGE('',*,*,#15790,.T.);
#21192=ORIENTED_EDGE('',*,*,#15530,.T.);
#21193=ORIENTED_EDGE('',*,*,#15639,.T.);
#21194=ORIENTED_EDGE('',*,*,#15791,.T.);
#21195=ORIENTED_EDGE('',*,*,#15792,.T.);
#21196=ORIENTED_EDGE('',*,*,#15791,.F.);
#21197=ORIENTED_EDGE('',*,*,#15638,.T.);
#21198=ORIENTED_EDGE('',*,*,#15793,.T.);
#21199=ORIENTED_EDGE('',*,*,#15637,.T.);
#21200=ORIENTED_EDGE('',*,*,#15534,.T.);
#21201=ORIENTED_EDGE('',*,*,#15794,.T.);
#21202=ORIENTED_EDGE('',*,*,#15793,.F.);
#21203=ORIENTED_EDGE('',*,*,#15790,.F.);
#21204=ORIENTED_EDGE('',*,*,#15795,.T.);
#21205=ORIENTED_EDGE('',*,*,#15796,.T.);
#21206=ORIENTED_EDGE('',*,*,#15531,.F.);
#21207=ORIENTED_EDGE('',*,*,#15792,.F.);
#21208=ORIENTED_EDGE('',*,*,#15797,.T.);
#21209=ORIENTED_EDGE('',*,*,#15798,.T.);
#21210=ORIENTED_EDGE('',*,*,#15795,.F.);
#21211=ORIENTED_EDGE('',*,*,#15794,.F.);
#21212=ORIENTED_EDGE('',*,*,#15533,.F.);
#21213=ORIENTED_EDGE('',*,*,#15799,.T.);
#21214=ORIENTED_EDGE('',*,*,#15797,.F.);
#21215=ORIENTED_EDGE('',*,*,#15528,.T.);
#21216=ORIENTED_EDGE('',*,*,#15800,.T.);
#21217=ORIENTED_EDGE('',*,*,#15801,.T.);
#21218=ORIENTED_EDGE('',*,*,#15640,.T.);
#21219=ORIENTED_EDGE('',*,*,#15800,.F.);
#21220=ORIENTED_EDGE('',*,*,#15527,.F.);
#21221=ORIENTED_EDGE('',*,*,#15802,.T.);
#21222=ORIENTED_EDGE('',*,*,#15803,.F.);
#21223=ORIENTED_EDGE('',*,*,#15804,.T.);
#21224=ORIENTED_EDGE('',*,*,#15524,.T.);
#21225=ORIENTED_EDGE('',*,*,#15642,.T.);
#21226=ORIENTED_EDGE('',*,*,#15805,.T.);
#21227=ORIENTED_EDGE('',*,*,#15641,.T.);
#21228=ORIENTED_EDGE('',*,*,#15801,.F.);
#21229=ORIENTED_EDGE('',*,*,#15806,.T.);
#21230=ORIENTED_EDGE('',*,*,#15805,.F.);
#21231=ORIENTED_EDGE('',*,*,#15804,.F.);
#21232=ORIENTED_EDGE('',*,*,#15807,.T.);
#21233=ORIENTED_EDGE('',*,*,#15808,.T.);
#21234=ORIENTED_EDGE('',*,*,#15525,.F.);
#21235=ORIENTED_EDGE('',*,*,#15806,.F.);
#21236=ORIENTED_EDGE('',*,*,#15803,.T.);
#21237=ORIENTED_EDGE('',*,*,#15809,.T.);
#21238=ORIENTED_EDGE('',*,*,#15807,.F.);
#21239=ORIENTED_EDGE('',*,*,#15810,.T.);
#21240=ORIENTED_EDGE('',*,*,#15518,.T.);
#21241=ORIENTED_EDGE('',*,*,#15645,.T.);
#21242=ORIENTED_EDGE('',*,*,#15811,.T.);
#21243=ORIENTED_EDGE('',*,*,#15812,.T.);
#21244=ORIENTED_EDGE('',*,*,#15811,.F.);
#21245=ORIENTED_EDGE('',*,*,#15644,.T.);
#21246=ORIENTED_EDGE('',*,*,#15813,.T.);
#21247=ORIENTED_EDGE('',*,*,#15643,.T.);
#21248=ORIENTED_EDGE('',*,*,#15522,.T.);
#21249=ORIENTED_EDGE('',*,*,#15814,.T.);
#21250=ORIENTED_EDGE('',*,*,#15813,.F.);
#21251=ORIENTED_EDGE('',*,*,#15810,.F.);
#21252=ORIENTED_EDGE('',*,*,#15815,.T.);
#21253=ORIENTED_EDGE('',*,*,#15816,.T.);
#21254=ORIENTED_EDGE('',*,*,#15519,.F.);
#21255=ORIENTED_EDGE('',*,*,#15812,.F.);
#21256=ORIENTED_EDGE('',*,*,#15817,.T.);
#21257=ORIENTED_EDGE('',*,*,#15818,.T.);
#21258=ORIENTED_EDGE('',*,*,#15815,.F.);
#21259=ORIENTED_EDGE('',*,*,#15814,.F.);
#21260=ORIENTED_EDGE('',*,*,#15521,.F.);
#21261=ORIENTED_EDGE('',*,*,#15819,.T.);
#21262=ORIENTED_EDGE('',*,*,#15817,.F.);
#21263=ORIENTED_EDGE('',*,*,#15820,.T.);
#21264=ORIENTED_EDGE('',*,*,#15512,.T.);
#21265=ORIENTED_EDGE('',*,*,#15648,.T.);
#21266=ORIENTED_EDGE('',*,*,#15821,.T.);
#21267=ORIENTED_EDGE('',*,*,#15822,.T.);
#21268=ORIENTED_EDGE('',*,*,#15821,.F.);
#21269=ORIENTED_EDGE('',*,*,#15647,.T.);
#21270=ORIENTED_EDGE('',*,*,#15823,.T.);
#21271=ORIENTED_EDGE('',*,*,#15646,.T.);
#21272=ORIENTED_EDGE('',*,*,#15516,.T.);
#21273=ORIENTED_EDGE('',*,*,#15824,.T.);
#21274=ORIENTED_EDGE('',*,*,#15823,.F.);
#21275=ORIENTED_EDGE('',*,*,#15820,.F.);
#21276=ORIENTED_EDGE('',*,*,#15825,.T.);
#21277=ORIENTED_EDGE('',*,*,#15826,.T.);
#21278=ORIENTED_EDGE('',*,*,#15513,.F.);
#21279=ORIENTED_EDGE('',*,*,#15822,.F.);
#21280=ORIENTED_EDGE('',*,*,#15827,.T.);
#21281=ORIENTED_EDGE('',*,*,#15828,.T.);
#21282=ORIENTED_EDGE('',*,*,#15825,.F.);
#21283=ORIENTED_EDGE('',*,*,#15824,.F.);
#21284=ORIENTED_EDGE('',*,*,#15515,.F.);
#21285=ORIENTED_EDGE('',*,*,#15829,.T.);
#21286=ORIENTED_EDGE('',*,*,#15827,.F.);
#21287=ORIENTED_EDGE('',*,*,#15830,.T.);
#21288=ORIENTED_EDGE('',*,*,#15506,.T.);
#21289=ORIENTED_EDGE('',*,*,#15651,.T.);
#21290=ORIENTED_EDGE('',*,*,#15831,.T.);
#21291=ORIENTED_EDGE('',*,*,#15832,.T.);
#21292=ORIENTED_EDGE('',*,*,#15831,.F.);
#21293=ORIENTED_EDGE('',*,*,#15650,.T.);
#21294=ORIENTED_EDGE('',*,*,#15833,.T.);
#21295=ORIENTED_EDGE('',*,*,#15649,.T.);
#21296=ORIENTED_EDGE('',*,*,#15510,.T.);
#21297=ORIENTED_EDGE('',*,*,#15834,.T.);
#21298=ORIENTED_EDGE('',*,*,#15833,.F.);
#21299=ORIENTED_EDGE('',*,*,#15830,.F.);
#21300=ORIENTED_EDGE('',*,*,#15835,.T.);
#21301=ORIENTED_EDGE('',*,*,#15836,.T.);
#21302=ORIENTED_EDGE('',*,*,#15507,.F.);
#21303=ORIENTED_EDGE('',*,*,#15832,.F.);
#21304=ORIENTED_EDGE('',*,*,#15837,.T.);
#21305=ORIENTED_EDGE('',*,*,#15838,.T.);
#21306=ORIENTED_EDGE('',*,*,#15835,.F.);
#21307=ORIENTED_EDGE('',*,*,#15834,.F.);
#21308=ORIENTED_EDGE('',*,*,#15509,.F.);
#21309=ORIENTED_EDGE('',*,*,#15839,.T.);
#21310=ORIENTED_EDGE('',*,*,#15837,.F.);
#21311=ORIENTED_EDGE('',*,*,#15840,.T.);
#21312=ORIENTED_EDGE('',*,*,#15500,.T.);
#21313=ORIENTED_EDGE('',*,*,#15654,.T.);
#21314=ORIENTED_EDGE('',*,*,#15841,.T.);
#21315=ORIENTED_EDGE('',*,*,#15842,.T.);
#21316=ORIENTED_EDGE('',*,*,#15841,.F.);
#21317=ORIENTED_EDGE('',*,*,#15653,.T.);
#21318=ORIENTED_EDGE('',*,*,#15843,.T.);
#21319=ORIENTED_EDGE('',*,*,#15652,.T.);
#21320=ORIENTED_EDGE('',*,*,#15504,.T.);
#21321=ORIENTED_EDGE('',*,*,#15844,.T.);
#21322=ORIENTED_EDGE('',*,*,#15843,.F.);
#21323=ORIENTED_EDGE('',*,*,#15840,.F.);
#21324=ORIENTED_EDGE('',*,*,#15845,.T.);
#21325=ORIENTED_EDGE('',*,*,#15846,.T.);
#21326=ORIENTED_EDGE('',*,*,#15501,.F.);
#21327=ORIENTED_EDGE('',*,*,#15842,.F.);
#21328=ORIENTED_EDGE('',*,*,#15847,.T.);
#21329=ORIENTED_EDGE('',*,*,#15848,.T.);
#21330=ORIENTED_EDGE('',*,*,#15845,.F.);
#21331=ORIENTED_EDGE('',*,*,#15844,.F.);
#21332=ORIENTED_EDGE('',*,*,#15503,.F.);
#21333=ORIENTED_EDGE('',*,*,#15849,.T.);
#21334=ORIENTED_EDGE('',*,*,#15847,.F.);
#21335=ORIENTED_EDGE('',*,*,#15850,.T.);
#21336=ORIENTED_EDGE('',*,*,#15494,.T.);
#21337=ORIENTED_EDGE('',*,*,#15657,.T.);
#21338=ORIENTED_EDGE('',*,*,#15851,.T.);
#21339=ORIENTED_EDGE('',*,*,#15852,.T.);
#21340=ORIENTED_EDGE('',*,*,#15851,.F.);
#21341=ORIENTED_EDGE('',*,*,#15656,.T.);
#21342=ORIENTED_EDGE('',*,*,#15853,.T.);
#21343=ORIENTED_EDGE('',*,*,#15655,.T.);
#21344=ORIENTED_EDGE('',*,*,#15498,.T.);
#21345=ORIENTED_EDGE('',*,*,#15854,.T.);
#21346=ORIENTED_EDGE('',*,*,#15853,.F.);
#21347=ORIENTED_EDGE('',*,*,#15850,.F.);
#21348=ORIENTED_EDGE('',*,*,#15855,.T.);
#21349=ORIENTED_EDGE('',*,*,#15856,.T.);
#21350=ORIENTED_EDGE('',*,*,#15495,.F.);
#21351=ORIENTED_EDGE('',*,*,#15852,.F.);
#21352=ORIENTED_EDGE('',*,*,#15857,.T.);
#21353=ORIENTED_EDGE('',*,*,#15858,.T.);
#21354=ORIENTED_EDGE('',*,*,#15855,.F.);
#21355=ORIENTED_EDGE('',*,*,#15854,.F.);
#21356=ORIENTED_EDGE('',*,*,#15497,.F.);
#21357=ORIENTED_EDGE('',*,*,#15859,.T.);
#21358=ORIENTED_EDGE('',*,*,#15857,.F.);
#21359=ORIENTED_EDGE('',*,*,#15860,.T.);
#21360=ORIENTED_EDGE('',*,*,#15488,.T.);
#21361=ORIENTED_EDGE('',*,*,#15660,.T.);
#21362=ORIENTED_EDGE('',*,*,#15861,.T.);
#21363=ORIENTED_EDGE('',*,*,#15862,.T.);
#21364=ORIENTED_EDGE('',*,*,#15861,.F.);
#21365=ORIENTED_EDGE('',*,*,#15659,.T.);
#21366=ORIENTED_EDGE('',*,*,#15863,.T.);
#21367=ORIENTED_EDGE('',*,*,#15658,.T.);
#21368=ORIENTED_EDGE('',*,*,#15492,.T.);
#21369=ORIENTED_EDGE('',*,*,#15864,.T.);
#21370=ORIENTED_EDGE('',*,*,#15863,.F.);
#21371=ORIENTED_EDGE('',*,*,#15860,.F.);
#21372=ORIENTED_EDGE('',*,*,#15865,.T.);
#21373=ORIENTED_EDGE('',*,*,#15866,.T.);
#21374=ORIENTED_EDGE('',*,*,#15489,.F.);
#21375=ORIENTED_EDGE('',*,*,#15862,.F.);
#21376=ORIENTED_EDGE('',*,*,#15867,.T.);
#21377=ORIENTED_EDGE('',*,*,#15868,.T.);
#21378=ORIENTED_EDGE('',*,*,#15865,.F.);
#21379=ORIENTED_EDGE('',*,*,#15864,.F.);
#21380=ORIENTED_EDGE('',*,*,#15491,.F.);
#21381=ORIENTED_EDGE('',*,*,#15869,.T.);
#21382=ORIENTED_EDGE('',*,*,#15867,.F.);
#21383=ORIENTED_EDGE('',*,*,#15870,.T.);
#21384=ORIENTED_EDGE('',*,*,#15482,.T.);
#21385=ORIENTED_EDGE('',*,*,#15663,.T.);
#21386=ORIENTED_EDGE('',*,*,#15871,.T.);
#21387=ORIENTED_EDGE('',*,*,#15872,.T.);
#21388=ORIENTED_EDGE('',*,*,#15871,.F.);
#21389=ORIENTED_EDGE('',*,*,#15662,.T.);
#21390=ORIENTED_EDGE('',*,*,#15873,.T.);
#21391=ORIENTED_EDGE('',*,*,#15661,.T.);
#21392=ORIENTED_EDGE('',*,*,#15486,.T.);
#21393=ORIENTED_EDGE('',*,*,#15874,.T.);
#21394=ORIENTED_EDGE('',*,*,#15873,.F.);
#21395=ORIENTED_EDGE('',*,*,#15870,.F.);
#21396=ORIENTED_EDGE('',*,*,#15875,.T.);
#21397=ORIENTED_EDGE('',*,*,#15876,.T.);
#21398=ORIENTED_EDGE('',*,*,#15483,.F.);
#21399=ORIENTED_EDGE('',*,*,#15872,.F.);
#21400=ORIENTED_EDGE('',*,*,#15877,.T.);
#21401=ORIENTED_EDGE('',*,*,#15878,.T.);
#21402=ORIENTED_EDGE('',*,*,#15875,.F.);
#21403=ORIENTED_EDGE('',*,*,#15874,.F.);
#21404=ORIENTED_EDGE('',*,*,#15485,.F.);
#21405=ORIENTED_EDGE('',*,*,#15879,.T.);
#21406=ORIENTED_EDGE('',*,*,#15877,.F.);
#21407=ORIENTED_EDGE('',*,*,#15880,.T.);
#21408=ORIENTED_EDGE('',*,*,#15476,.T.);
#21409=ORIENTED_EDGE('',*,*,#15666,.T.);
#21410=ORIENTED_EDGE('',*,*,#15881,.T.);
#21411=ORIENTED_EDGE('',*,*,#15882,.T.);
#21412=ORIENTED_EDGE('',*,*,#15881,.F.);
#21413=ORIENTED_EDGE('',*,*,#15665,.T.);
#21414=ORIENTED_EDGE('',*,*,#15883,.T.);
#21415=ORIENTED_EDGE('',*,*,#15664,.T.);
#21416=ORIENTED_EDGE('',*,*,#15480,.T.);
#21417=ORIENTED_EDGE('',*,*,#15884,.T.);
#21418=ORIENTED_EDGE('',*,*,#15883,.F.);
#21419=ORIENTED_EDGE('',*,*,#15880,.F.);
#21420=ORIENTED_EDGE('',*,*,#15885,.T.);
#21421=ORIENTED_EDGE('',*,*,#15886,.T.);
#21422=ORIENTED_EDGE('',*,*,#15477,.F.);
#21423=ORIENTED_EDGE('',*,*,#15882,.F.);
#21424=ORIENTED_EDGE('',*,*,#15887,.T.);
#21425=ORIENTED_EDGE('',*,*,#15888,.T.);
#21426=ORIENTED_EDGE('',*,*,#15885,.F.);
#21427=ORIENTED_EDGE('',*,*,#15884,.F.);
#21428=ORIENTED_EDGE('',*,*,#15479,.F.);
#21429=ORIENTED_EDGE('',*,*,#15889,.T.);
#21430=ORIENTED_EDGE('',*,*,#15887,.F.);
#21431=ORIENTED_EDGE('',*,*,#15890,.T.);
#21432=ORIENTED_EDGE('',*,*,#15470,.T.);
#21433=ORIENTED_EDGE('',*,*,#15669,.T.);
#21434=ORIENTED_EDGE('',*,*,#15891,.T.);
#21435=ORIENTED_EDGE('',*,*,#15892,.T.);
#21436=ORIENTED_EDGE('',*,*,#15891,.F.);
#21437=ORIENTED_EDGE('',*,*,#15668,.T.);
#21438=ORIENTED_EDGE('',*,*,#15893,.T.);
#21439=ORIENTED_EDGE('',*,*,#15667,.T.);
#21440=ORIENTED_EDGE('',*,*,#15474,.T.);
#21441=ORIENTED_EDGE('',*,*,#15894,.T.);
#21442=ORIENTED_EDGE('',*,*,#15893,.F.);
#21443=ORIENTED_EDGE('',*,*,#15890,.F.);
#21444=ORIENTED_EDGE('',*,*,#15895,.T.);
#21445=ORIENTED_EDGE('',*,*,#15896,.T.);
#21446=ORIENTED_EDGE('',*,*,#15471,.F.);
#21447=ORIENTED_EDGE('',*,*,#15892,.F.);
#21448=ORIENTED_EDGE('',*,*,#15897,.T.);
#21449=ORIENTED_EDGE('',*,*,#15898,.T.);
#21450=ORIENTED_EDGE('',*,*,#15895,.F.);
#21451=ORIENTED_EDGE('',*,*,#15894,.F.);
#21452=ORIENTED_EDGE('',*,*,#15473,.F.);
#21453=ORIENTED_EDGE('',*,*,#15899,.T.);
#21454=ORIENTED_EDGE('',*,*,#15897,.F.);
#21455=ORIENTED_EDGE('',*,*,#15900,.T.);
#21456=ORIENTED_EDGE('',*,*,#15464,.T.);
#21457=ORIENTED_EDGE('',*,*,#15672,.T.);
#21458=ORIENTED_EDGE('',*,*,#15901,.T.);
#21459=ORIENTED_EDGE('',*,*,#15902,.T.);
#21460=ORIENTED_EDGE('',*,*,#15901,.F.);
#21461=ORIENTED_EDGE('',*,*,#15671,.T.);
#21462=ORIENTED_EDGE('',*,*,#15903,.T.);
#21463=ORIENTED_EDGE('',*,*,#15670,.T.);
#21464=ORIENTED_EDGE('',*,*,#15468,.T.);
#21465=ORIENTED_EDGE('',*,*,#15904,.T.);
#21466=ORIENTED_EDGE('',*,*,#15903,.F.);
#21467=ORIENTED_EDGE('',*,*,#15900,.F.);
#21468=ORIENTED_EDGE('',*,*,#15905,.T.);
#21469=ORIENTED_EDGE('',*,*,#15906,.T.);
#21470=ORIENTED_EDGE('',*,*,#15465,.F.);
#21471=ORIENTED_EDGE('',*,*,#15902,.F.);
#21472=ORIENTED_EDGE('',*,*,#15907,.T.);
#21473=ORIENTED_EDGE('',*,*,#15908,.T.);
#21474=ORIENTED_EDGE('',*,*,#15905,.F.);
#21475=ORIENTED_EDGE('',*,*,#15904,.F.);
#21476=ORIENTED_EDGE('',*,*,#15467,.F.);
#21477=ORIENTED_EDGE('',*,*,#15909,.T.);
#21478=ORIENTED_EDGE('',*,*,#15907,.F.);
#21479=ORIENTED_EDGE('',*,*,#15910,.T.);
#21480=ORIENTED_EDGE('',*,*,#15458,.T.);
#21481=ORIENTED_EDGE('',*,*,#15675,.T.);
#21482=ORIENTED_EDGE('',*,*,#15911,.T.);
#21483=ORIENTED_EDGE('',*,*,#15912,.T.);
#21484=ORIENTED_EDGE('',*,*,#15911,.F.);
#21485=ORIENTED_EDGE('',*,*,#15674,.T.);
#21486=ORIENTED_EDGE('',*,*,#15913,.T.);
#21487=ORIENTED_EDGE('',*,*,#15673,.T.);
#21488=ORIENTED_EDGE('',*,*,#15462,.T.);
#21489=ORIENTED_EDGE('',*,*,#15914,.T.);
#21490=ORIENTED_EDGE('',*,*,#15913,.F.);
#21491=ORIENTED_EDGE('',*,*,#15910,.F.);
#21492=ORIENTED_EDGE('',*,*,#15915,.T.);
#21493=ORIENTED_EDGE('',*,*,#15916,.T.);
#21494=ORIENTED_EDGE('',*,*,#15459,.F.);
#21495=ORIENTED_EDGE('',*,*,#15912,.F.);
#21496=ORIENTED_EDGE('',*,*,#15917,.T.);
#21497=ORIENTED_EDGE('',*,*,#15918,.T.);
#21498=ORIENTED_EDGE('',*,*,#15915,.F.);
#21499=ORIENTED_EDGE('',*,*,#15914,.F.);
#21500=ORIENTED_EDGE('',*,*,#15461,.F.);
#21501=ORIENTED_EDGE('',*,*,#15919,.T.);
#21502=ORIENTED_EDGE('',*,*,#15917,.F.);
#21503=ORIENTED_EDGE('',*,*,#15920,.T.);
#21504=ORIENTED_EDGE('',*,*,#15452,.T.);
#21505=ORIENTED_EDGE('',*,*,#15678,.T.);
#21506=ORIENTED_EDGE('',*,*,#15921,.T.);
#21507=ORIENTED_EDGE('',*,*,#15922,.T.);
#21508=ORIENTED_EDGE('',*,*,#15921,.F.);
#21509=ORIENTED_EDGE('',*,*,#15677,.T.);
#21510=ORIENTED_EDGE('',*,*,#15923,.T.);
#21511=ORIENTED_EDGE('',*,*,#15676,.T.);
#21512=ORIENTED_EDGE('',*,*,#15456,.T.);
#21513=ORIENTED_EDGE('',*,*,#15924,.T.);
#21514=ORIENTED_EDGE('',*,*,#15923,.F.);
#21515=ORIENTED_EDGE('',*,*,#15920,.F.);
#21516=ORIENTED_EDGE('',*,*,#15925,.T.);
#21517=ORIENTED_EDGE('',*,*,#15926,.T.);
#21518=ORIENTED_EDGE('',*,*,#15453,.F.);
#21519=ORIENTED_EDGE('',*,*,#15922,.F.);
#21520=ORIENTED_EDGE('',*,*,#15927,.T.);
#21521=ORIENTED_EDGE('',*,*,#15928,.T.);
#21522=ORIENTED_EDGE('',*,*,#15925,.F.);
#21523=ORIENTED_EDGE('',*,*,#15924,.F.);
#21524=ORIENTED_EDGE('',*,*,#15455,.F.);
#21525=ORIENTED_EDGE('',*,*,#15929,.T.);
#21526=ORIENTED_EDGE('',*,*,#15927,.F.);
#21527=ORIENTED_EDGE('',*,*,#15930,.T.);
#21528=ORIENTED_EDGE('',*,*,#15931,.T.);
#21529=ORIENTED_EDGE('',*,*,#15932,.T.);
#21530=ORIENTED_EDGE('',*,*,#15933,.T.);
#21531=ORIENTED_EDGE('',*,*,#15934,.T.);
#21532=ORIENTED_EDGE('',*,*,#15355,.T.);
#21533=ORIENTED_EDGE('',*,*,#15935,.T.);
#21534=ORIENTED_EDGE('',*,*,#15933,.F.);
#21535=ORIENTED_EDGE('',*,*,#15936,.F.);
#21536=ORIENTED_EDGE('',*,*,#15930,.F.);
#21537=ORIENTED_EDGE('',*,*,#15935,.F.);
#21538=ORIENTED_EDGE('',*,*,#15354,.F.);
#21539=ORIENTED_EDGE('',*,*,#15937,.F.);
#21540=ORIENTED_EDGE('',*,*,#15938,.F.);
#21541=ORIENTED_EDGE('',*,*,#15939,.F.);
#21542=ORIENTED_EDGE('',*,*,#15348,.F.);
#21543=ORIENTED_EDGE('',*,*,#15940,.F.);
#21544=ORIENTED_EDGE('',*,*,#15941,.F.);
#21545=ORIENTED_EDGE('',*,*,#15942,.F.);
#21546=ORIENTED_EDGE('',*,*,#15342,.F.);
#21547=ORIENTED_EDGE('',*,*,#15943,.F.);
#21548=ORIENTED_EDGE('',*,*,#15944,.F.);
#21549=ORIENTED_EDGE('',*,*,#15945,.F.);
#21550=ORIENTED_EDGE('',*,*,#15336,.F.);
#21551=ORIENTED_EDGE('',*,*,#15946,.F.);
#21552=ORIENTED_EDGE('',*,*,#15947,.F.);
#21553=ORIENTED_EDGE('',*,*,#15948,.F.);
#21554=ORIENTED_EDGE('',*,*,#15330,.F.);
#21555=ORIENTED_EDGE('',*,*,#15949,.F.);
#21556=ORIENTED_EDGE('',*,*,#15950,.F.);
#21557=ORIENTED_EDGE('',*,*,#15951,.F.);
#21558=ORIENTED_EDGE('',*,*,#15324,.F.);
#21559=ORIENTED_EDGE('',*,*,#15952,.F.);
#21560=ORIENTED_EDGE('',*,*,#15953,.F.);
#21561=ORIENTED_EDGE('',*,*,#15954,.F.);
#21562=ORIENTED_EDGE('',*,*,#15318,.F.);
#21563=ORIENTED_EDGE('',*,*,#15955,.F.);
#21564=ORIENTED_EDGE('',*,*,#15956,.F.);
#21565=ORIENTED_EDGE('',*,*,#15957,.F.);
#21566=ORIENTED_EDGE('',*,*,#15312,.F.);
#21567=ORIENTED_EDGE('',*,*,#15958,.F.);
#21568=ORIENTED_EDGE('',*,*,#15959,.F.);
#21569=ORIENTED_EDGE('',*,*,#15960,.F.);
#21570=ORIENTED_EDGE('',*,*,#15306,.F.);
#21571=ORIENTED_EDGE('',*,*,#15961,.F.);
#21572=ORIENTED_EDGE('',*,*,#15962,.F.);
#21573=ORIENTED_EDGE('',*,*,#15963,.F.);
#21574=ORIENTED_EDGE('',*,*,#15300,.F.);
#21575=ORIENTED_EDGE('',*,*,#15964,.F.);
#21576=ORIENTED_EDGE('',*,*,#15965,.F.);
#21577=ORIENTED_EDGE('',*,*,#15966,.F.);
#21578=ORIENTED_EDGE('',*,*,#15294,.F.);
#21579=ORIENTED_EDGE('',*,*,#15967,.F.);
#21580=ORIENTED_EDGE('',*,*,#15968,.F.);
#21581=ORIENTED_EDGE('',*,*,#15969,.F.);
#21582=ORIENTED_EDGE('',*,*,#15288,.F.);
#21583=ORIENTED_EDGE('',*,*,#15970,.F.);
#21584=ORIENTED_EDGE('',*,*,#15971,.F.);
#21585=ORIENTED_EDGE('',*,*,#15972,.F.);
#21586=ORIENTED_EDGE('',*,*,#15282,.F.);
#21587=ORIENTED_EDGE('',*,*,#15973,.F.);
#21588=ORIENTED_EDGE('',*,*,#15974,.F.);
#21589=ORIENTED_EDGE('',*,*,#15975,.F.);
#21590=ORIENTED_EDGE('',*,*,#15276,.F.);
#21591=ORIENTED_EDGE('',*,*,#15976,.F.);
#21592=ORIENTED_EDGE('',*,*,#15977,.F.);
#21593=ORIENTED_EDGE('',*,*,#15978,.F.);
#21594=ORIENTED_EDGE('',*,*,#15270,.F.);
#21595=ORIENTED_EDGE('',*,*,#15979,.F.);
#21596=ORIENTED_EDGE('',*,*,#15980,.F.);
#21597=ORIENTED_EDGE('',*,*,#15981,.F.);
#21598=ORIENTED_EDGE('',*,*,#15264,.F.);
#21599=ORIENTED_EDGE('',*,*,#15982,.F.);
#21600=ORIENTED_EDGE('',*,*,#15983,.F.);
#21601=ORIENTED_EDGE('',*,*,#15984,.F.);
#21602=ORIENTED_EDGE('',*,*,#15258,.F.);
#21603=ORIENTED_EDGE('',*,*,#15985,.F.);
#21604=ORIENTED_EDGE('',*,*,#15986,.F.);
#21605=ORIENTED_EDGE('',*,*,#15987,.F.);
#21606=ORIENTED_EDGE('',*,*,#15252,.F.);
#21607=ORIENTED_EDGE('',*,*,#15988,.F.);
#21608=ORIENTED_EDGE('',*,*,#15989,.F.);
#21609=ORIENTED_EDGE('',*,*,#15990,.F.);
#21610=ORIENTED_EDGE('',*,*,#15246,.F.);
#21611=ORIENTED_EDGE('',*,*,#15991,.F.);
#21612=ORIENTED_EDGE('',*,*,#15992,.F.);
#21613=ORIENTED_EDGE('',*,*,#15993,.F.);
#21614=ORIENTED_EDGE('',*,*,#15240,.F.);
#21615=ORIENTED_EDGE('',*,*,#15994,.F.);
#21616=ORIENTED_EDGE('',*,*,#15995,.F.);
#21617=ORIENTED_EDGE('',*,*,#15996,.F.);
#21618=ORIENTED_EDGE('',*,*,#15234,.F.);
#21619=ORIENTED_EDGE('',*,*,#15997,.F.);
#21620=ORIENTED_EDGE('',*,*,#15998,.F.);
#21621=ORIENTED_EDGE('',*,*,#15999,.F.);
#21622=ORIENTED_EDGE('',*,*,#15228,.F.);
#21623=ORIENTED_EDGE('',*,*,#16000,.F.);
#21624=ORIENTED_EDGE('',*,*,#16001,.F.);
#21625=ORIENTED_EDGE('',*,*,#16002,.F.);
#21626=ORIENTED_EDGE('',*,*,#15222,.F.);
#21627=ORIENTED_EDGE('',*,*,#15402,.F.);
#21628=ORIENTED_EDGE('',*,*,#16003,.F.);
#21629=ORIENTED_EDGE('',*,*,#16004,.F.);
#21630=ORIENTED_EDGE('',*,*,#16005,.F.);
#21631=ORIENTED_EDGE('',*,*,#15396,.F.);
#21632=ORIENTED_EDGE('',*,*,#16006,.F.);
#21633=ORIENTED_EDGE('',*,*,#16007,.F.);
#21634=ORIENTED_EDGE('',*,*,#16008,.F.);
#21635=ORIENTED_EDGE('',*,*,#15390,.F.);
#21636=ORIENTED_EDGE('',*,*,#16009,.F.);
#21637=ORIENTED_EDGE('',*,*,#16010,.F.);
#21638=ORIENTED_EDGE('',*,*,#16011,.F.);
#21639=ORIENTED_EDGE('',*,*,#15384,.F.);
#21640=ORIENTED_EDGE('',*,*,#16012,.F.);
#21641=ORIENTED_EDGE('',*,*,#16013,.F.);
#21642=ORIENTED_EDGE('',*,*,#16014,.F.);
#21643=ORIENTED_EDGE('',*,*,#15378,.F.);
#21644=ORIENTED_EDGE('',*,*,#16015,.F.);
#21645=ORIENTED_EDGE('',*,*,#16016,.F.);
#21646=ORIENTED_EDGE('',*,*,#16017,.F.);
#21647=ORIENTED_EDGE('',*,*,#15372,.F.);
#21648=ORIENTED_EDGE('',*,*,#16018,.F.);
#21649=ORIENTED_EDGE('',*,*,#16019,.F.);
#21650=ORIENTED_EDGE('',*,*,#16020,.F.);
#21651=ORIENTED_EDGE('',*,*,#15366,.F.);
#21652=ORIENTED_EDGE('',*,*,#16021,.F.);
#21653=ORIENTED_EDGE('',*,*,#16022,.F.);
#21654=ORIENTED_EDGE('',*,*,#16023,.F.);
#21655=ORIENTED_EDGE('',*,*,#15360,.F.);
#21656=ORIENTED_EDGE('',*,*,#16024,.F.);
#21657=ORIENTED_EDGE('',*,*,#16025,.F.);
#21658=ORIENTED_EDGE('',*,*,#16026,.F.);
#21659=ORIENTED_EDGE('',*,*,#16027,.T.);
#21660=ORIENTED_EDGE('',*,*,#16028,.F.);
#21661=ORIENTED_EDGE('',*,*,#16029,.F.);
#21662=ORIENTED_EDGE('',*,*,#16030,.F.);
#21663=ORIENTED_EDGE('',*,*,#16031,.T.);
#21664=ORIENTED_EDGE('',*,*,#15359,.T.);
#21665=ORIENTED_EDGE('',*,*,#16032,.T.);
#21666=ORIENTED_EDGE('',*,*,#15931,.F.);
#21667=ORIENTED_EDGE('',*,*,#15936,.T.);
#21668=ORIENTED_EDGE('',*,*,#16022,.T.);
#21669=ORIENTED_EDGE('',*,*,#16033,.T.);
#21670=ORIENTED_EDGE('',*,*,#16034,.T.);
#21671=ORIENTED_EDGE('',*,*,#16035,.T.);
#21672=ORIENTED_EDGE('',*,*,#16021,.T.);
#21673=ORIENTED_EDGE('',*,*,#15365,.T.);
#21674=ORIENTED_EDGE('',*,*,#16036,.T.);
#21675=ORIENTED_EDGE('',*,*,#16033,.F.);
#21676=ORIENTED_EDGE('',*,*,#16037,.T.);
#21677=ORIENTED_EDGE('',*,*,#15361,.T.);
#21678=ORIENTED_EDGE('',*,*,#16023,.T.);
#21679=ORIENTED_EDGE('',*,*,#16035,.F.);
#21680=ORIENTED_EDGE('',*,*,#16019,.T.);
#21681=ORIENTED_EDGE('',*,*,#16038,.T.);
#21682=ORIENTED_EDGE('',*,*,#16039,.T.);
#21683=ORIENTED_EDGE('',*,*,#16040,.T.);
#21684=ORIENTED_EDGE('',*,*,#16018,.T.);
#21685=ORIENTED_EDGE('',*,*,#15371,.T.);
#21686=ORIENTED_EDGE('',*,*,#16041,.T.);
#21687=ORIENTED_EDGE('',*,*,#16038,.F.);
#21688=ORIENTED_EDGE('',*,*,#16042,.T.);
#21689=ORIENTED_EDGE('',*,*,#15367,.T.);
#21690=ORIENTED_EDGE('',*,*,#16020,.T.);
#21691=ORIENTED_EDGE('',*,*,#16040,.F.);
#21692=ORIENTED_EDGE('',*,*,#16042,.F.);
#21693=ORIENTED_EDGE('',*,*,#16043,.T.);
#21694=ORIENTED_EDGE('',*,*,#16044,.T.);
#21695=ORIENTED_EDGE('',*,*,#15368,.F.);
#21696=ORIENTED_EDGE('',*,*,#16039,.F.);
#21697=ORIENTED_EDGE('',*,*,#16045,.T.);
#21698=ORIENTED_EDGE('',*,*,#16046,.T.);
#21699=ORIENTED_EDGE('',*,*,#16043,.F.);
#21700=ORIENTED_EDGE('',*,*,#16016,.T.);
#21701=ORIENTED_EDGE('',*,*,#16047,.T.);
#21702=ORIENTED_EDGE('',*,*,#16048,.T.);
#21703=ORIENTED_EDGE('',*,*,#16049,.T.);
#21704=ORIENTED_EDGE('',*,*,#16015,.T.);
#21705=ORIENTED_EDGE('',*,*,#15377,.T.);
#21706=ORIENTED_EDGE('',*,*,#16050,.T.);
#21707=ORIENTED_EDGE('',*,*,#16047,.F.);
#21708=ORIENTED_EDGE('',*,*,#16051,.T.);
#21709=ORIENTED_EDGE('',*,*,#15373,.T.);
#21710=ORIENTED_EDGE('',*,*,#16017,.T.);
#21711=ORIENTED_EDGE('',*,*,#16049,.F.);
#21712=ORIENTED_EDGE('',*,*,#16013,.T.);
#21713=ORIENTED_EDGE('',*,*,#16052,.T.);
#21714=ORIENTED_EDGE('',*,*,#16053,.T.);
#21715=ORIENTED_EDGE('',*,*,#16054,.T.);
#21716=ORIENTED_EDGE('',*,*,#16012,.T.);
#21717=ORIENTED_EDGE('',*,*,#15383,.T.);
#21718=ORIENTED_EDGE('',*,*,#16055,.T.);
#21719=ORIENTED_EDGE('',*,*,#16052,.F.);
#21720=ORIENTED_EDGE('',*,*,#16056,.T.);
#21721=ORIENTED_EDGE('',*,*,#15379,.T.);
#21722=ORIENTED_EDGE('',*,*,#16014,.T.);
#21723=ORIENTED_EDGE('',*,*,#16054,.F.);
#21724=ORIENTED_EDGE('',*,*,#16056,.F.);
#21725=ORIENTED_EDGE('',*,*,#16057,.T.);
#21726=ORIENTED_EDGE('',*,*,#16058,.T.);
#21727=ORIENTED_EDGE('',*,*,#15380,.F.);
#21728=ORIENTED_EDGE('',*,*,#16053,.F.);
#21729=ORIENTED_EDGE('',*,*,#16059,.T.);
#21730=ORIENTED_EDGE('',*,*,#16060,.T.);
#21731=ORIENTED_EDGE('',*,*,#16057,.F.);
#21732=ORIENTED_EDGE('',*,*,#16010,.T.);
#21733=ORIENTED_EDGE('',*,*,#16061,.T.);
#21734=ORIENTED_EDGE('',*,*,#16062,.T.);
#21735=ORIENTED_EDGE('',*,*,#16063,.T.);
#21736=ORIENTED_EDGE('',*,*,#16009,.T.);
#21737=ORIENTED_EDGE('',*,*,#15389,.T.);
#21738=ORIENTED_EDGE('',*,*,#16064,.T.);
#21739=ORIENTED_EDGE('',*,*,#16061,.F.);
#21740=ORIENTED_EDGE('',*,*,#16065,.T.);
#21741=ORIENTED_EDGE('',*,*,#15385,.T.);
#21742=ORIENTED_EDGE('',*,*,#16011,.T.);
#21743=ORIENTED_EDGE('',*,*,#16063,.F.);
#21744=ORIENTED_EDGE('',*,*,#16007,.T.);
#21745=ORIENTED_EDGE('',*,*,#16066,.T.);
#21746=ORIENTED_EDGE('',*,*,#16067,.T.);
#21747=ORIENTED_EDGE('',*,*,#16068,.T.);
#21748=ORIENTED_EDGE('',*,*,#16006,.T.);
#21749=ORIENTED_EDGE('',*,*,#15395,.T.);
#21750=ORIENTED_EDGE('',*,*,#16069,.T.);
#21751=ORIENTED_EDGE('',*,*,#16066,.F.);
#21752=ORIENTED_EDGE('',*,*,#16070,.T.);
#21753=ORIENTED_EDGE('',*,*,#15391,.T.);
#21754=ORIENTED_EDGE('',*,*,#16008,.T.);
#21755=ORIENTED_EDGE('',*,*,#16068,.F.);
#21756=ORIENTED_EDGE('',*,*,#16070,.F.);
#21757=ORIENTED_EDGE('',*,*,#16071,.T.);
#21758=ORIENTED_EDGE('',*,*,#16072,.T.);
#21759=ORIENTED_EDGE('',*,*,#15392,.F.);
#21760=ORIENTED_EDGE('',*,*,#16067,.F.);
#21761=ORIENTED_EDGE('',*,*,#16073,.T.);
#21762=ORIENTED_EDGE('',*,*,#16074,.T.);
#21763=ORIENTED_EDGE('',*,*,#16071,.F.);
#21764=ORIENTED_EDGE('',*,*,#15397,.T.);
#21765=ORIENTED_EDGE('',*,*,#16005,.T.);
#21766=ORIENTED_EDGE('',*,*,#16075,.T.);
#21767=ORIENTED_EDGE('',*,*,#16076,.T.);
#21768=ORIENTED_EDGE('',*,*,#16077,.T.);
#21769=ORIENTED_EDGE('',*,*,#16075,.F.);
#21770=ORIENTED_EDGE('',*,*,#16004,.T.);
#21771=ORIENTED_EDGE('',*,*,#16078,.T.);
#21772=ORIENTED_EDGE('',*,*,#16003,.T.);
#21773=ORIENTED_EDGE('',*,*,#15401,.T.);
#21774=ORIENTED_EDGE('',*,*,#16079,.T.);
#21775=ORIENTED_EDGE('',*,*,#16078,.F.);
#21776=ORIENTED_EDGE('',*,*,#16001,.T.);
#21777=ORIENTED_EDGE('',*,*,#16080,.T.);
#21778=ORIENTED_EDGE('',*,*,#16081,.T.);
#21779=ORIENTED_EDGE('',*,*,#16082,.T.);
#21780=ORIENTED_EDGE('',*,*,#16000,.T.);
#21781=ORIENTED_EDGE('',*,*,#15227,.T.);
#21782=ORIENTED_EDGE('',*,*,#16083,.T.);
#21783=ORIENTED_EDGE('',*,*,#16080,.F.);
#21784=ORIENTED_EDGE('',*,*,#16084,.T.);
#21785=ORIENTED_EDGE('',*,*,#15223,.T.);
#21786=ORIENTED_EDGE('',*,*,#16002,.T.);
#21787=ORIENTED_EDGE('',*,*,#16082,.F.);
#21788=ORIENTED_EDGE('',*,*,#15998,.T.);
#21789=ORIENTED_EDGE('',*,*,#16085,.T.);
#21790=ORIENTED_EDGE('',*,*,#16086,.T.);
#21791=ORIENTED_EDGE('',*,*,#16087,.T.);
#21792=ORIENTED_EDGE('',*,*,#15997,.T.);
#21793=ORIENTED_EDGE('',*,*,#15233,.T.);
#21794=ORIENTED_EDGE('',*,*,#16088,.T.);
#21795=ORIENTED_EDGE('',*,*,#16085,.F.);
#21796=ORIENTED_EDGE('',*,*,#16089,.T.);
#21797=ORIENTED_EDGE('',*,*,#15229,.T.);
#21798=ORIENTED_EDGE('',*,*,#15999,.T.);
#21799=ORIENTED_EDGE('',*,*,#16087,.F.);
#21800=ORIENTED_EDGE('',*,*,#16089,.F.);
#21801=ORIENTED_EDGE('',*,*,#16090,.T.);
#21802=ORIENTED_EDGE('',*,*,#16091,.T.);
#21803=ORIENTED_EDGE('',*,*,#15230,.F.);
#21804=ORIENTED_EDGE('',*,*,#16086,.F.);
#21805=ORIENTED_EDGE('',*,*,#16092,.T.);
#21806=ORIENTED_EDGE('',*,*,#16093,.T.);
#21807=ORIENTED_EDGE('',*,*,#16090,.F.);
#21808=ORIENTED_EDGE('',*,*,#15995,.T.);
#21809=ORIENTED_EDGE('',*,*,#16094,.T.);
#21810=ORIENTED_EDGE('',*,*,#16095,.T.);
#21811=ORIENTED_EDGE('',*,*,#16096,.T.);
#21812=ORIENTED_EDGE('',*,*,#15994,.T.);
#21813=ORIENTED_EDGE('',*,*,#15239,.T.);
#21814=ORIENTED_EDGE('',*,*,#16097,.T.);
#21815=ORIENTED_EDGE('',*,*,#16094,.F.);
#21816=ORIENTED_EDGE('',*,*,#16098,.T.);
#21817=ORIENTED_EDGE('',*,*,#15235,.T.);
#21818=ORIENTED_EDGE('',*,*,#15996,.T.);
#21819=ORIENTED_EDGE('',*,*,#16096,.F.);
#21820=ORIENTED_EDGE('',*,*,#15992,.T.);
#21821=ORIENTED_EDGE('',*,*,#16099,.T.);
#21822=ORIENTED_EDGE('',*,*,#16100,.T.);
#21823=ORIENTED_EDGE('',*,*,#16101,.T.);
#21824=ORIENTED_EDGE('',*,*,#15991,.T.);
#21825=ORIENTED_EDGE('',*,*,#15245,.T.);
#21826=ORIENTED_EDGE('',*,*,#16102,.T.);
#21827=ORIENTED_EDGE('',*,*,#16099,.F.);
#21828=ORIENTED_EDGE('',*,*,#16103,.T.);
#21829=ORIENTED_EDGE('',*,*,#15241,.T.);
#21830=ORIENTED_EDGE('',*,*,#15993,.T.);
#21831=ORIENTED_EDGE('',*,*,#16101,.F.);
#21832=ORIENTED_EDGE('',*,*,#16103,.F.);
#21833=ORIENTED_EDGE('',*,*,#16104,.T.);
#21834=ORIENTED_EDGE('',*,*,#16105,.T.);
#21835=ORIENTED_EDGE('',*,*,#15242,.F.);
#21836=ORIENTED_EDGE('',*,*,#16100,.F.);
#21837=ORIENTED_EDGE('',*,*,#16106,.T.);
#21838=ORIENTED_EDGE('',*,*,#16107,.T.);
#21839=ORIENTED_EDGE('',*,*,#16104,.F.);
#21840=ORIENTED_EDGE('',*,*,#15989,.T.);
#21841=ORIENTED_EDGE('',*,*,#16108,.T.);
#21842=ORIENTED_EDGE('',*,*,#16109,.T.);
#21843=ORIENTED_EDGE('',*,*,#16110,.T.);
#21844=ORIENTED_EDGE('',*,*,#15988,.T.);
#21845=ORIENTED_EDGE('',*,*,#15251,.T.);
#21846=ORIENTED_EDGE('',*,*,#16111,.T.);
#21847=ORIENTED_EDGE('',*,*,#16108,.F.);
#21848=ORIENTED_EDGE('',*,*,#16112,.T.);
#21849=ORIENTED_EDGE('',*,*,#15247,.T.);
#21850=ORIENTED_EDGE('',*,*,#15990,.T.);
#21851=ORIENTED_EDGE('',*,*,#16110,.F.);
#21852=ORIENTED_EDGE('',*,*,#15986,.T.);
#21853=ORIENTED_EDGE('',*,*,#16113,.T.);
#21854=ORIENTED_EDGE('',*,*,#16114,.T.);
#21855=ORIENTED_EDGE('',*,*,#16115,.T.);
#21856=ORIENTED_EDGE('',*,*,#15985,.T.);
#21857=ORIENTED_EDGE('',*,*,#15257,.T.);
#21858=ORIENTED_EDGE('',*,*,#16116,.T.);
#21859=ORIENTED_EDGE('',*,*,#16113,.F.);
#21860=ORIENTED_EDGE('',*,*,#16117,.T.);
#21861=ORIENTED_EDGE('',*,*,#15253,.T.);
#21862=ORIENTED_EDGE('',*,*,#15987,.T.);
#21863=ORIENTED_EDGE('',*,*,#16115,.F.);
#21864=ORIENTED_EDGE('',*,*,#16117,.F.);
#21865=ORIENTED_EDGE('',*,*,#16118,.T.);
#21866=ORIENTED_EDGE('',*,*,#16119,.T.);
#21867=ORIENTED_EDGE('',*,*,#15254,.F.);
#21868=ORIENTED_EDGE('',*,*,#16114,.F.);
#21869=ORIENTED_EDGE('',*,*,#16120,.T.);
#21870=ORIENTED_EDGE('',*,*,#16121,.T.);
#21871=ORIENTED_EDGE('',*,*,#16118,.F.);
#21872=ORIENTED_EDGE('',*,*,#15983,.T.);
#21873=ORIENTED_EDGE('',*,*,#16122,.T.);
#21874=ORIENTED_EDGE('',*,*,#16123,.T.);
#21875=ORIENTED_EDGE('',*,*,#16124,.T.);
#21876=ORIENTED_EDGE('',*,*,#15982,.T.);
#21877=ORIENTED_EDGE('',*,*,#15263,.T.);
#21878=ORIENTED_EDGE('',*,*,#16125,.T.);
#21879=ORIENTED_EDGE('',*,*,#16122,.F.);
#21880=ORIENTED_EDGE('',*,*,#16126,.T.);
#21881=ORIENTED_EDGE('',*,*,#15259,.T.);
#21882=ORIENTED_EDGE('',*,*,#15984,.T.);
#21883=ORIENTED_EDGE('',*,*,#16124,.F.);
#21884=ORIENTED_EDGE('',*,*,#15980,.T.);
#21885=ORIENTED_EDGE('',*,*,#16127,.T.);
#21886=ORIENTED_EDGE('',*,*,#16128,.T.);
#21887=ORIENTED_EDGE('',*,*,#16129,.T.);
#21888=ORIENTED_EDGE('',*,*,#15979,.T.);
#21889=ORIENTED_EDGE('',*,*,#15269,.T.);
#21890=ORIENTED_EDGE('',*,*,#16130,.T.);
#21891=ORIENTED_EDGE('',*,*,#16127,.F.);
#21892=ORIENTED_EDGE('',*,*,#16131,.T.);
#21893=ORIENTED_EDGE('',*,*,#15265,.T.);
#21894=ORIENTED_EDGE('',*,*,#15981,.T.);
#21895=ORIENTED_EDGE('',*,*,#16129,.F.);
#21896=ORIENTED_EDGE('',*,*,#16131,.F.);
#21897=ORIENTED_EDGE('',*,*,#16132,.T.);
#21898=ORIENTED_EDGE('',*,*,#16133,.T.);
#21899=ORIENTED_EDGE('',*,*,#15266,.F.);
#21900=ORIENTED_EDGE('',*,*,#16128,.F.);
#21901=ORIENTED_EDGE('',*,*,#16134,.T.);
#21902=ORIENTED_EDGE('',*,*,#16135,.T.);
#21903=ORIENTED_EDGE('',*,*,#16132,.F.);
#21904=ORIENTED_EDGE('',*,*,#15977,.T.);
#21905=ORIENTED_EDGE('',*,*,#16136,.T.);
#21906=ORIENTED_EDGE('',*,*,#16137,.T.);
#21907=ORIENTED_EDGE('',*,*,#16138,.T.);
#21908=ORIENTED_EDGE('',*,*,#15976,.T.);
#21909=ORIENTED_EDGE('',*,*,#15275,.T.);
#21910=ORIENTED_EDGE('',*,*,#16139,.T.);
#21911=ORIENTED_EDGE('',*,*,#16136,.F.);
#21912=ORIENTED_EDGE('',*,*,#16140,.T.);
#21913=ORIENTED_EDGE('',*,*,#15271,.T.);
#21914=ORIENTED_EDGE('',*,*,#15978,.T.);
#21915=ORIENTED_EDGE('',*,*,#16138,.F.);
#21916=ORIENTED_EDGE('',*,*,#15974,.T.);
#21917=ORIENTED_EDGE('',*,*,#16141,.T.);
#21918=ORIENTED_EDGE('',*,*,#16142,.T.);
#21919=ORIENTED_EDGE('',*,*,#16143,.T.);
#21920=ORIENTED_EDGE('',*,*,#15973,.T.);
#21921=ORIENTED_EDGE('',*,*,#15281,.T.);
#21922=ORIENTED_EDGE('',*,*,#16144,.T.);
#21923=ORIENTED_EDGE('',*,*,#16141,.F.);
#21924=ORIENTED_EDGE('',*,*,#16145,.T.);
#21925=ORIENTED_EDGE('',*,*,#15277,.T.);
#21926=ORIENTED_EDGE('',*,*,#15975,.T.);
#21927=ORIENTED_EDGE('',*,*,#16143,.F.);
#21928=ORIENTED_EDGE('',*,*,#16145,.F.);
#21929=ORIENTED_EDGE('',*,*,#16146,.T.);
#21930=ORIENTED_EDGE('',*,*,#16147,.T.);
#21931=ORIENTED_EDGE('',*,*,#15278,.F.);
#21932=ORIENTED_EDGE('',*,*,#16142,.F.);
#21933=ORIENTED_EDGE('',*,*,#16148,.T.);
#21934=ORIENTED_EDGE('',*,*,#16149,.T.);
#21935=ORIENTED_EDGE('',*,*,#16146,.F.);
#21936=ORIENTED_EDGE('',*,*,#15971,.T.);
#21937=ORIENTED_EDGE('',*,*,#16150,.T.);
#21938=ORIENTED_EDGE('',*,*,#16151,.T.);
#21939=ORIENTED_EDGE('',*,*,#16152,.T.);
#21940=ORIENTED_EDGE('',*,*,#15970,.T.);
#21941=ORIENTED_EDGE('',*,*,#15287,.T.);
#21942=ORIENTED_EDGE('',*,*,#16153,.T.);
#21943=ORIENTED_EDGE('',*,*,#16150,.F.);
#21944=ORIENTED_EDGE('',*,*,#16154,.T.);
#21945=ORIENTED_EDGE('',*,*,#15283,.T.);
#21946=ORIENTED_EDGE('',*,*,#15972,.T.);
#21947=ORIENTED_EDGE('',*,*,#16152,.F.);
#21948=ORIENTED_EDGE('',*,*,#15968,.T.);
#21949=ORIENTED_EDGE('',*,*,#16155,.T.);
#21950=ORIENTED_EDGE('',*,*,#16156,.T.);
#21951=ORIENTED_EDGE('',*,*,#16157,.T.);
#21952=ORIENTED_EDGE('',*,*,#15967,.T.);
#21953=ORIENTED_EDGE('',*,*,#15293,.T.);
#21954=ORIENTED_EDGE('',*,*,#16158,.T.);
#21955=ORIENTED_EDGE('',*,*,#16155,.F.);
#21956=ORIENTED_EDGE('',*,*,#16159,.T.);
#21957=ORIENTED_EDGE('',*,*,#15289,.T.);
#21958=ORIENTED_EDGE('',*,*,#15969,.T.);
#21959=ORIENTED_EDGE('',*,*,#16157,.F.);
#21960=ORIENTED_EDGE('',*,*,#16159,.F.);
#21961=ORIENTED_EDGE('',*,*,#16160,.T.);
#21962=ORIENTED_EDGE('',*,*,#16161,.T.);
#21963=ORIENTED_EDGE('',*,*,#15290,.F.);
#21964=ORIENTED_EDGE('',*,*,#16156,.F.);
#21965=ORIENTED_EDGE('',*,*,#16162,.T.);
#21966=ORIENTED_EDGE('',*,*,#16163,.T.);
#21967=ORIENTED_EDGE('',*,*,#16160,.F.);
#21968=ORIENTED_EDGE('',*,*,#15965,.T.);
#21969=ORIENTED_EDGE('',*,*,#16164,.T.);
#21970=ORIENTED_EDGE('',*,*,#16165,.T.);
#21971=ORIENTED_EDGE('',*,*,#16166,.T.);
#21972=ORIENTED_EDGE('',*,*,#16167,.T.);
#21973=ORIENTED_EDGE('',*,*,#15295,.T.);
#21974=ORIENTED_EDGE('',*,*,#15966,.T.);
#21975=ORIENTED_EDGE('',*,*,#16166,.F.);
#21976=ORIENTED_EDGE('',*,*,#15299,.T.);
#21977=ORIENTED_EDGE('',*,*,#16168,.T.);
#21978=ORIENTED_EDGE('',*,*,#16164,.F.);
#21979=ORIENTED_EDGE('',*,*,#15964,.T.);
#21980=ORIENTED_EDGE('',*,*,#15962,.T.);
#21981=ORIENTED_EDGE('',*,*,#16169,.T.);
#21982=ORIENTED_EDGE('',*,*,#16170,.T.);
#21983=ORIENTED_EDGE('',*,*,#16171,.T.);
#21984=ORIENTED_EDGE('',*,*,#15961,.T.);
#21985=ORIENTED_EDGE('',*,*,#15305,.T.);
#21986=ORIENTED_EDGE('',*,*,#16172,.T.);
#21987=ORIENTED_EDGE('',*,*,#16169,.F.);
#21988=ORIENTED_EDGE('',*,*,#16173,.T.);
#21989=ORIENTED_EDGE('',*,*,#15301,.T.);
#21990=ORIENTED_EDGE('',*,*,#15963,.T.);
#21991=ORIENTED_EDGE('',*,*,#16171,.F.);
#21992=ORIENTED_EDGE('',*,*,#15959,.T.);
#21993=ORIENTED_EDGE('',*,*,#16174,.T.);
#21994=ORIENTED_EDGE('',*,*,#16175,.T.);
#21995=ORIENTED_EDGE('',*,*,#16176,.T.);
#21996=ORIENTED_EDGE('',*,*,#15958,.T.);
#21997=ORIENTED_EDGE('',*,*,#15311,.T.);
#21998=ORIENTED_EDGE('',*,*,#16177,.T.);
#21999=ORIENTED_EDGE('',*,*,#16174,.F.);
#22000=ORIENTED_EDGE('',*,*,#16178,.T.);
#22001=ORIENTED_EDGE('',*,*,#15307,.T.);
#22002=ORIENTED_EDGE('',*,*,#15960,.T.);
#22003=ORIENTED_EDGE('',*,*,#16176,.F.);
#22004=ORIENTED_EDGE('',*,*,#16178,.F.);
#22005=ORIENTED_EDGE('',*,*,#16179,.T.);
#22006=ORIENTED_EDGE('',*,*,#16180,.T.);
#22007=ORIENTED_EDGE('',*,*,#15308,.F.);
#22008=ORIENTED_EDGE('',*,*,#16175,.F.);
#22009=ORIENTED_EDGE('',*,*,#16181,.T.);
#22010=ORIENTED_EDGE('',*,*,#16182,.T.);
#22011=ORIENTED_EDGE('',*,*,#16179,.F.);
#22012=ORIENTED_EDGE('',*,*,#15956,.T.);
#22013=ORIENTED_EDGE('',*,*,#16183,.T.);
#22014=ORIENTED_EDGE('',*,*,#16184,.T.);
#22015=ORIENTED_EDGE('',*,*,#16185,.T.);
#22016=ORIENTED_EDGE('',*,*,#15955,.T.);
#22017=ORIENTED_EDGE('',*,*,#15317,.T.);
#22018=ORIENTED_EDGE('',*,*,#16186,.T.);
#22019=ORIENTED_EDGE('',*,*,#16183,.F.);
#22020=ORIENTED_EDGE('',*,*,#16187,.T.);
#22021=ORIENTED_EDGE('',*,*,#15313,.T.);
#22022=ORIENTED_EDGE('',*,*,#15957,.T.);
#22023=ORIENTED_EDGE('',*,*,#16185,.F.);
#22024=ORIENTED_EDGE('',*,*,#15953,.T.);
#22025=ORIENTED_EDGE('',*,*,#16188,.T.);
#22026=ORIENTED_EDGE('',*,*,#16189,.T.);
#22027=ORIENTED_EDGE('',*,*,#16190,.T.);
#22028=ORIENTED_EDGE('',*,*,#15952,.T.);
#22029=ORIENTED_EDGE('',*,*,#15323,.T.);
#22030=ORIENTED_EDGE('',*,*,#16191,.T.);
#22031=ORIENTED_EDGE('',*,*,#16188,.F.);
#22032=ORIENTED_EDGE('',*,*,#16192,.T.);
#22033=ORIENTED_EDGE('',*,*,#15319,.T.);
#22034=ORIENTED_EDGE('',*,*,#15954,.T.);
#22035=ORIENTED_EDGE('',*,*,#16190,.F.);
#22036=ORIENTED_EDGE('',*,*,#16192,.F.);
#22037=ORIENTED_EDGE('',*,*,#16193,.T.);
#22038=ORIENTED_EDGE('',*,*,#16194,.T.);
#22039=ORIENTED_EDGE('',*,*,#15320,.F.);
#22040=ORIENTED_EDGE('',*,*,#16189,.F.);
#22041=ORIENTED_EDGE('',*,*,#16195,.T.);
#22042=ORIENTED_EDGE('',*,*,#16196,.T.);
#22043=ORIENTED_EDGE('',*,*,#16193,.F.);
#22044=ORIENTED_EDGE('',*,*,#15950,.T.);
#22045=ORIENTED_EDGE('',*,*,#16197,.T.);
#22046=ORIENTED_EDGE('',*,*,#16198,.T.);
#22047=ORIENTED_EDGE('',*,*,#16199,.T.);
#22048=ORIENTED_EDGE('',*,*,#15949,.T.);
#22049=ORIENTED_EDGE('',*,*,#15329,.T.);
#22050=ORIENTED_EDGE('',*,*,#16200,.T.);
#22051=ORIENTED_EDGE('',*,*,#16197,.F.);
#22052=ORIENTED_EDGE('',*,*,#16201,.T.);
#22053=ORIENTED_EDGE('',*,*,#15325,.T.);
#22054=ORIENTED_EDGE('',*,*,#15951,.T.);
#22055=ORIENTED_EDGE('',*,*,#16199,.F.);
#22056=ORIENTED_EDGE('',*,*,#15947,.T.);
#22057=ORIENTED_EDGE('',*,*,#16202,.T.);
#22058=ORIENTED_EDGE('',*,*,#16203,.T.);
#22059=ORIENTED_EDGE('',*,*,#16204,.T.);
#22060=ORIENTED_EDGE('',*,*,#15946,.T.);
#22061=ORIENTED_EDGE('',*,*,#15335,.T.);
#22062=ORIENTED_EDGE('',*,*,#16205,.T.);
#22063=ORIENTED_EDGE('',*,*,#16202,.F.);
#22064=ORIENTED_EDGE('',*,*,#16206,.T.);
#22065=ORIENTED_EDGE('',*,*,#15331,.T.);
#22066=ORIENTED_EDGE('',*,*,#15948,.T.);
#22067=ORIENTED_EDGE('',*,*,#16204,.F.);
#22068=ORIENTED_EDGE('',*,*,#16206,.F.);
#22069=ORIENTED_EDGE('',*,*,#16207,.T.);
#22070=ORIENTED_EDGE('',*,*,#16208,.T.);
#22071=ORIENTED_EDGE('',*,*,#15332,.F.);
#22072=ORIENTED_EDGE('',*,*,#16203,.F.);
#22073=ORIENTED_EDGE('',*,*,#16209,.T.);
#22074=ORIENTED_EDGE('',*,*,#16210,.T.);
#22075=ORIENTED_EDGE('',*,*,#16207,.F.);
#22076=ORIENTED_EDGE('',*,*,#15337,.T.);
#22077=ORIENTED_EDGE('',*,*,#15945,.T.);
#22078=ORIENTED_EDGE('',*,*,#16211,.T.);
#22079=ORIENTED_EDGE('',*,*,#16212,.T.);
#22080=ORIENTED_EDGE('',*,*,#16213,.T.);
#22081=ORIENTED_EDGE('',*,*,#16211,.F.);
#22082=ORIENTED_EDGE('',*,*,#15944,.T.);
#22083=ORIENTED_EDGE('',*,*,#16214,.T.);
#22084=ORIENTED_EDGE('',*,*,#15943,.T.);
#22085=ORIENTED_EDGE('',*,*,#15341,.T.);
#22086=ORIENTED_EDGE('',*,*,#16215,.T.);
#22087=ORIENTED_EDGE('',*,*,#16214,.F.);
#22088=ORIENTED_EDGE('',*,*,#15941,.T.);
#22089=ORIENTED_EDGE('',*,*,#16216,.T.);
#22090=ORIENTED_EDGE('',*,*,#16217,.T.);
#22091=ORIENTED_EDGE('',*,*,#16218,.T.);
#22092=ORIENTED_EDGE('',*,*,#15940,.T.);
#22093=ORIENTED_EDGE('',*,*,#15347,.T.);
#22094=ORIENTED_EDGE('',*,*,#16219,.T.);
#22095=ORIENTED_EDGE('',*,*,#16216,.F.);
#22096=ORIENTED_EDGE('',*,*,#16220,.T.);
#22097=ORIENTED_EDGE('',*,*,#15343,.T.);
#22098=ORIENTED_EDGE('',*,*,#15942,.T.);
#22099=ORIENTED_EDGE('',*,*,#16218,.F.);
#22100=ORIENTED_EDGE('',*,*,#15938,.T.);
#22101=ORIENTED_EDGE('',*,*,#16221,.T.);
#22102=ORIENTED_EDGE('',*,*,#16222,.T.);
#22103=ORIENTED_EDGE('',*,*,#16223,.T.);
#22104=ORIENTED_EDGE('',*,*,#15937,.T.);
#22105=ORIENTED_EDGE('',*,*,#15353,.T.);
#22106=ORIENTED_EDGE('',*,*,#16224,.T.);
#22107=ORIENTED_EDGE('',*,*,#16221,.F.);
#22108=ORIENTED_EDGE('',*,*,#16225,.T.);
#22109=ORIENTED_EDGE('',*,*,#15349,.T.);
#22110=ORIENTED_EDGE('',*,*,#15939,.T.);
#22111=ORIENTED_EDGE('',*,*,#16223,.F.);
#22112=ORIENTED_EDGE('',*,*,#16225,.F.);
#22113=ORIENTED_EDGE('',*,*,#16226,.T.);
#22114=ORIENTED_EDGE('',*,*,#16227,.T.);
#22115=ORIENTED_EDGE('',*,*,#15350,.F.);
#22116=ORIENTED_EDGE('',*,*,#16222,.F.);
#22117=ORIENTED_EDGE('',*,*,#16228,.T.);
#22118=ORIENTED_EDGE('',*,*,#16229,.T.);
#22119=ORIENTED_EDGE('',*,*,#16226,.F.);
#22120=ORIENTED_EDGE('',*,*,#15704,.T.);
#22121=ORIENTED_EDGE('',*,*,#16230,.T.);
#22122=ORIENTED_EDGE('',*,*,#16231,.T.);
#22123=ORIENTED_EDGE('',*,*,#16232,.T.);
#22124=ORIENTED_EDGE('',*,*,#15703,.T.);
#22125=ORIENTED_EDGE('',*,*,#16233,.T.);
#22126=ORIENTED_EDGE('',*,*,#16234,.T.);
#22127=ORIENTED_EDGE('',*,*,#16230,.F.);
#22128=ORIENTED_EDGE('',*,*,#16235,.T.);
#22129=ORIENTED_EDGE('',*,*,#16236,.T.);
#22130=ORIENTED_EDGE('',*,*,#15697,.T.);
#22131=ORIENTED_EDGE('',*,*,#16232,.F.);
#22132=ORIENTED_EDGE('',*,*,#16235,.F.);
#22133=ORIENTED_EDGE('',*,*,#16237,.F.);
#22134=ORIENTED_EDGE('',*,*,#16238,.F.);
#22135=ORIENTED_EDGE('',*,*,#16239,.F.);
#22136=ORIENTED_EDGE('',*,*,#16231,.F.);
#22137=ORIENTED_EDGE('',*,*,#16240,.F.);
#22138=ORIENTED_EDGE('',*,*,#16241,.F.);
#22139=ORIENTED_EDGE('',*,*,#16237,.T.);
#22140=ORIENTED_EDGE('',*,*,#16234,.F.);
#22141=ORIENTED_EDGE('',*,*,#16242,.F.);
#22142=ORIENTED_EDGE('',*,*,#16243,.F.);
#22143=ORIENTED_EDGE('',*,*,#16240,.T.);
#22144=ORIENTED_EDGE('',*,*,#16233,.F.);
#22145=ORIENTED_EDGE('',*,*,#15702,.T.);
#22146=ORIENTED_EDGE('',*,*,#16244,.F.);
#22147=ORIENTED_EDGE('',*,*,#16245,.T.);
#22148=ORIENTED_EDGE('',*,*,#16246,.F.);
#22149=ORIENTED_EDGE('',*,*,#16027,.F.);
#22150=ORIENTED_EDGE('',*,*,#16247,.F.);
#22151=ORIENTED_EDGE('',*,*,#16242,.T.);
#22152=ORIENTED_EDGE('',*,*,#16241,.T.);
#22153=ORIENTED_EDGE('',*,*,#16248,.T.);
#22154=ORIENTED_EDGE('',*,*,#16025,.T.);
#22155=ORIENTED_EDGE('',*,*,#16249,.T.);
#22156=ORIENTED_EDGE('',*,*,#16243,.T.);
#22157=ORIENTED_EDGE('',*,*,#16247,.T.);
#22158=ORIENTED_EDGE('',*,*,#16026,.T.);
#22159=ORIENTED_EDGE('',*,*,#16248,.F.);
#22160=ORIENTED_EDGE('',*,*,#16024,.T.);
#22161=ORIENTED_EDGE('',*,*,#16250,.T.);
#22162=ORIENTED_EDGE('',*,*,#16238,.T.);
#22163=ORIENTED_EDGE('',*,*,#16249,.F.);
#22164=ORIENTED_EDGE('',*,*,#16251,.T.);
#22165=ORIENTED_EDGE('',*,*,#16252,.T.);
#22166=ORIENTED_EDGE('',*,*,#16030,.T.);
#22167=ORIENTED_EDGE('',*,*,#16253,.T.);
#22168=ORIENTED_EDGE('',*,*,#16029,.T.);
#22169=ORIENTED_EDGE('',*,*,#16254,.T.);
#22170=ORIENTED_EDGE('',*,*,#16255,.T.);
#22171=ORIENTED_EDGE('',*,*,#16253,.F.);
#22172=ORIENTED_EDGE('',*,*,#16028,.T.);
#22173=ORIENTED_EDGE('',*,*,#16246,.T.);
#22174=ORIENTED_EDGE('',*,*,#16256,.T.);
#22175=ORIENTED_EDGE('',*,*,#16254,.F.);
#22176=ORIENTED_EDGE('',*,*,#16251,.F.);
#22177=ORIENTED_EDGE('',*,*,#16257,.T.);
#22178=ORIENTED_EDGE('',*,*,#16258,.F.);
#22179=ORIENTED_EDGE('',*,*,#16259,.F.);
#22180=ORIENTED_EDGE('',*,*,#16255,.F.);
#22181=ORIENTED_EDGE('',*,*,#16260,.T.);
#22182=ORIENTED_EDGE('',*,*,#16261,.F.);
#22183=ORIENTED_EDGE('',*,*,#16257,.F.);
#22184=ORIENTED_EDGE('',*,*,#16256,.F.);
#22185=ORIENTED_EDGE('',*,*,#16245,.F.);
#22186=ORIENTED_EDGE('',*,*,#16262,.F.);
#22187=ORIENTED_EDGE('',*,*,#16260,.F.);
#22188=ORIENTED_EDGE('',*,*,#15699,.T.);
#22189=ORIENTED_EDGE('',*,*,#16263,.T.);
#22190=ORIENTED_EDGE('',*,*,#16258,.T.);
#22191=ORIENTED_EDGE('',*,*,#16264,.T.);
#22192=ORIENTED_EDGE('',*,*,#16261,.T.);
#22193=ORIENTED_EDGE('',*,*,#16265,.T.);
#22194=ORIENTED_EDGE('',*,*,#15700,.T.);
#22195=ORIENTED_EDGE('',*,*,#16264,.F.);
#22196=ORIENTED_EDGE('',*,*,#16262,.T.);
#22197=ORIENTED_EDGE('',*,*,#16244,.T.);
#22198=ORIENTED_EDGE('',*,*,#15701,.T.);
#22199=ORIENTED_EDGE('',*,*,#16265,.F.);
#22200=ORIENTED_EDGE('',*,*,#15454,.F.);
#22201=ORIENTED_EDGE('',*,*,#15926,.F.);
#22202=ORIENTED_EDGE('',*,*,#15928,.F.);
#22203=ORIENTED_EDGE('',*,*,#15929,.F.);
#22204=ORIENTED_EDGE('',*,*,#16224,.F.);
#22205=ORIENTED_EDGE('',*,*,#15352,.F.);
#22206=ORIENTED_EDGE('',*,*,#16266,.T.);
#22207=ORIENTED_EDGE('',*,*,#16228,.F.);
#22208=ORIENTED_EDGE('',*,*,#15351,.F.);
#22209=ORIENTED_EDGE('',*,*,#16227,.F.);
#22210=ORIENTED_EDGE('',*,*,#16229,.F.);
#22211=ORIENTED_EDGE('',*,*,#16266,.F.);
#22212=ORIENTED_EDGE('',*,*,#15460,.F.);
#22213=ORIENTED_EDGE('',*,*,#15916,.F.);
#22214=ORIENTED_EDGE('',*,*,#15918,.F.);
#22215=ORIENTED_EDGE('',*,*,#15919,.F.);
#22216=ORIENTED_EDGE('',*,*,#16217,.F.);
#22217=ORIENTED_EDGE('',*,*,#16267,.T.);
#22218=ORIENTED_EDGE('',*,*,#16268,.T.);
#22219=ORIENTED_EDGE('',*,*,#16269,.F.);
#22220=ORIENTED_EDGE('',*,*,#16219,.F.);
#22221=ORIENTED_EDGE('',*,*,#15346,.F.);
#22222=ORIENTED_EDGE('',*,*,#16270,.T.);
#22223=ORIENTED_EDGE('',*,*,#16267,.F.);
#22224=ORIENTED_EDGE('',*,*,#16220,.F.);
#22225=ORIENTED_EDGE('',*,*,#16269,.T.);
#22226=ORIENTED_EDGE('',*,*,#16271,.T.);
#22227=ORIENTED_EDGE('',*,*,#15344,.F.);
#22228=ORIENTED_EDGE('',*,*,#15345,.F.);
#22229=ORIENTED_EDGE('',*,*,#16271,.F.);
#22230=ORIENTED_EDGE('',*,*,#16268,.F.);
#22231=ORIENTED_EDGE('',*,*,#16270,.F.);
#22232=ORIENTED_EDGE('',*,*,#15466,.F.);
#22233=ORIENTED_EDGE('',*,*,#15906,.F.);
#22234=ORIENTED_EDGE('',*,*,#15908,.F.);
#22235=ORIENTED_EDGE('',*,*,#15909,.F.);
#22236=ORIENTED_EDGE('',*,*,#16213,.F.);
#22237=ORIENTED_EDGE('',*,*,#16272,.T.);
#22238=ORIENTED_EDGE('',*,*,#16273,.T.);
#22239=ORIENTED_EDGE('',*,*,#16274,.F.);
#22240=ORIENTED_EDGE('',*,*,#16215,.F.);
#22241=ORIENTED_EDGE('',*,*,#15340,.F.);
#22242=ORIENTED_EDGE('',*,*,#16275,.T.);
#22243=ORIENTED_EDGE('',*,*,#16272,.F.);
#22244=ORIENTED_EDGE('',*,*,#16212,.F.);
#22245=ORIENTED_EDGE('',*,*,#16274,.T.);
#22246=ORIENTED_EDGE('',*,*,#16276,.T.);
#22247=ORIENTED_EDGE('',*,*,#15338,.F.);
#22248=ORIENTED_EDGE('',*,*,#15339,.F.);
#22249=ORIENTED_EDGE('',*,*,#16276,.F.);
#22250=ORIENTED_EDGE('',*,*,#16273,.F.);
#22251=ORIENTED_EDGE('',*,*,#16275,.F.);
#22252=ORIENTED_EDGE('',*,*,#15472,.F.);
#22253=ORIENTED_EDGE('',*,*,#15896,.F.);
#22254=ORIENTED_EDGE('',*,*,#15898,.F.);
#22255=ORIENTED_EDGE('',*,*,#15899,.F.);
#22256=ORIENTED_EDGE('',*,*,#16205,.F.);
#22257=ORIENTED_EDGE('',*,*,#15334,.F.);
#22258=ORIENTED_EDGE('',*,*,#16277,.T.);
#22259=ORIENTED_EDGE('',*,*,#16209,.F.);
#22260=ORIENTED_EDGE('',*,*,#15333,.F.);
#22261=ORIENTED_EDGE('',*,*,#16208,.F.);
#22262=ORIENTED_EDGE('',*,*,#16210,.F.);
#22263=ORIENTED_EDGE('',*,*,#16277,.F.);
#22264=ORIENTED_EDGE('',*,*,#15478,.F.);
#22265=ORIENTED_EDGE('',*,*,#15886,.F.);
#22266=ORIENTED_EDGE('',*,*,#15888,.F.);
#22267=ORIENTED_EDGE('',*,*,#15889,.F.);
#22268=ORIENTED_EDGE('',*,*,#16198,.F.);
#22269=ORIENTED_EDGE('',*,*,#16278,.T.);
#22270=ORIENTED_EDGE('',*,*,#16279,.T.);
#22271=ORIENTED_EDGE('',*,*,#16280,.F.);
#22272=ORIENTED_EDGE('',*,*,#16200,.F.);
#22273=ORIENTED_EDGE('',*,*,#15328,.F.);
#22274=ORIENTED_EDGE('',*,*,#16281,.T.);
#22275=ORIENTED_EDGE('',*,*,#16278,.F.);
#22276=ORIENTED_EDGE('',*,*,#16201,.F.);
#22277=ORIENTED_EDGE('',*,*,#16280,.T.);
#22278=ORIENTED_EDGE('',*,*,#16282,.T.);
#22279=ORIENTED_EDGE('',*,*,#15326,.F.);
#22280=ORIENTED_EDGE('',*,*,#15327,.F.);
#22281=ORIENTED_EDGE('',*,*,#16282,.F.);
#22282=ORIENTED_EDGE('',*,*,#16279,.F.);
#22283=ORIENTED_EDGE('',*,*,#16281,.F.);
#22284=ORIENTED_EDGE('',*,*,#15484,.F.);
#22285=ORIENTED_EDGE('',*,*,#15876,.F.);
#22286=ORIENTED_EDGE('',*,*,#15878,.F.);
#22287=ORIENTED_EDGE('',*,*,#15879,.F.);
#22288=ORIENTED_EDGE('',*,*,#16191,.F.);
#22289=ORIENTED_EDGE('',*,*,#15322,.F.);
#22290=ORIENTED_EDGE('',*,*,#16283,.T.);
#22291=ORIENTED_EDGE('',*,*,#16195,.F.);
#22292=ORIENTED_EDGE('',*,*,#15321,.F.);
#22293=ORIENTED_EDGE('',*,*,#16194,.F.);
#22294=ORIENTED_EDGE('',*,*,#16196,.F.);
#22295=ORIENTED_EDGE('',*,*,#16283,.F.);
#22296=ORIENTED_EDGE('',*,*,#15490,.F.);
#22297=ORIENTED_EDGE('',*,*,#15866,.F.);
#22298=ORIENTED_EDGE('',*,*,#15868,.F.);
#22299=ORIENTED_EDGE('',*,*,#15869,.F.);
#22300=ORIENTED_EDGE('',*,*,#16184,.F.);
#22301=ORIENTED_EDGE('',*,*,#16284,.T.);
#22302=ORIENTED_EDGE('',*,*,#16285,.T.);
#22303=ORIENTED_EDGE('',*,*,#16286,.F.);
#22304=ORIENTED_EDGE('',*,*,#16186,.F.);
#22305=ORIENTED_EDGE('',*,*,#15316,.F.);
#22306=ORIENTED_EDGE('',*,*,#16287,.T.);
#22307=ORIENTED_EDGE('',*,*,#16284,.F.);
#22308=ORIENTED_EDGE('',*,*,#16187,.F.);
#22309=ORIENTED_EDGE('',*,*,#16286,.T.);
#22310=ORIENTED_EDGE('',*,*,#16288,.T.);
#22311=ORIENTED_EDGE('',*,*,#15314,.F.);
#22312=ORIENTED_EDGE('',*,*,#15315,.F.);
#22313=ORIENTED_EDGE('',*,*,#16288,.F.);
#22314=ORIENTED_EDGE('',*,*,#16285,.F.);
#22315=ORIENTED_EDGE('',*,*,#16287,.F.);
#22316=ORIENTED_EDGE('',*,*,#15496,.F.);
#22317=ORIENTED_EDGE('',*,*,#15856,.F.);
#22318=ORIENTED_EDGE('',*,*,#15858,.F.);
#22319=ORIENTED_EDGE('',*,*,#15859,.F.);
#22320=ORIENTED_EDGE('',*,*,#16177,.F.);
#22321=ORIENTED_EDGE('',*,*,#15310,.F.);
#22322=ORIENTED_EDGE('',*,*,#16289,.T.);
#22323=ORIENTED_EDGE('',*,*,#16181,.F.);
#22324=ORIENTED_EDGE('',*,*,#15309,.F.);
#22325=ORIENTED_EDGE('',*,*,#16180,.F.);
#22326=ORIENTED_EDGE('',*,*,#16182,.F.);
#22327=ORIENTED_EDGE('',*,*,#16289,.F.);
#22328=ORIENTED_EDGE('',*,*,#15502,.F.);
#22329=ORIENTED_EDGE('',*,*,#15846,.F.);
#22330=ORIENTED_EDGE('',*,*,#15848,.F.);
#22331=ORIENTED_EDGE('',*,*,#15849,.F.);
#22332=ORIENTED_EDGE('',*,*,#16170,.F.);
#22333=ORIENTED_EDGE('',*,*,#16290,.T.);
#22334=ORIENTED_EDGE('',*,*,#16291,.T.);
#22335=ORIENTED_EDGE('',*,*,#16292,.F.);
#22336=ORIENTED_EDGE('',*,*,#16172,.F.);
#22337=ORIENTED_EDGE('',*,*,#15304,.F.);
#22338=ORIENTED_EDGE('',*,*,#16293,.T.);
#22339=ORIENTED_EDGE('',*,*,#16290,.F.);
#22340=ORIENTED_EDGE('',*,*,#16173,.F.);
#22341=ORIENTED_EDGE('',*,*,#16292,.T.);
#22342=ORIENTED_EDGE('',*,*,#16294,.T.);
#22343=ORIENTED_EDGE('',*,*,#15302,.F.);
#22344=ORIENTED_EDGE('',*,*,#15303,.F.);
#22345=ORIENTED_EDGE('',*,*,#16294,.F.);
#22346=ORIENTED_EDGE('',*,*,#16291,.F.);
#22347=ORIENTED_EDGE('',*,*,#16293,.F.);
#22348=ORIENTED_EDGE('',*,*,#15508,.F.);
#22349=ORIENTED_EDGE('',*,*,#15836,.F.);
#22350=ORIENTED_EDGE('',*,*,#15838,.F.);
#22351=ORIENTED_EDGE('',*,*,#15839,.F.);
#22352=ORIENTED_EDGE('',*,*,#16165,.F.);
#22353=ORIENTED_EDGE('',*,*,#16295,.T.);
#22354=ORIENTED_EDGE('',*,*,#16296,.T.);
#22355=ORIENTED_EDGE('',*,*,#16297,.F.);
#22356=ORIENTED_EDGE('',*,*,#16168,.F.);
#22357=ORIENTED_EDGE('',*,*,#15298,.F.);
#22358=ORIENTED_EDGE('',*,*,#16298,.T.);
#22359=ORIENTED_EDGE('',*,*,#16295,.F.);
#22360=ORIENTED_EDGE('',*,*,#16167,.F.);
#22361=ORIENTED_EDGE('',*,*,#16297,.T.);
#22362=ORIENTED_EDGE('',*,*,#16299,.T.);
#22363=ORIENTED_EDGE('',*,*,#15296,.F.);
#22364=ORIENTED_EDGE('',*,*,#15297,.F.);
#22365=ORIENTED_EDGE('',*,*,#16299,.F.);
#22366=ORIENTED_EDGE('',*,*,#16296,.F.);
#22367=ORIENTED_EDGE('',*,*,#16298,.F.);
#22368=ORIENTED_EDGE('',*,*,#15514,.F.);
#22369=ORIENTED_EDGE('',*,*,#15826,.F.);
#22370=ORIENTED_EDGE('',*,*,#15828,.F.);
#22371=ORIENTED_EDGE('',*,*,#15829,.F.);
#22372=ORIENTED_EDGE('',*,*,#16158,.F.);
#22373=ORIENTED_EDGE('',*,*,#15292,.F.);
#22374=ORIENTED_EDGE('',*,*,#16300,.T.);
#22375=ORIENTED_EDGE('',*,*,#16162,.F.);
#22376=ORIENTED_EDGE('',*,*,#15291,.F.);
#22377=ORIENTED_EDGE('',*,*,#16161,.F.);
#22378=ORIENTED_EDGE('',*,*,#16163,.F.);
#22379=ORIENTED_EDGE('',*,*,#16300,.F.);
#22380=ORIENTED_EDGE('',*,*,#15520,.F.);
#22381=ORIENTED_EDGE('',*,*,#15816,.F.);
#22382=ORIENTED_EDGE('',*,*,#15818,.F.);
#22383=ORIENTED_EDGE('',*,*,#15819,.F.);
#22384=ORIENTED_EDGE('',*,*,#16151,.F.);
#22385=ORIENTED_EDGE('',*,*,#16301,.T.);
#22386=ORIENTED_EDGE('',*,*,#16302,.T.);
#22387=ORIENTED_EDGE('',*,*,#16303,.F.);
#22388=ORIENTED_EDGE('',*,*,#16153,.F.);
#22389=ORIENTED_EDGE('',*,*,#15286,.F.);
#22390=ORIENTED_EDGE('',*,*,#16304,.T.);
#22391=ORIENTED_EDGE('',*,*,#16301,.F.);
#22392=ORIENTED_EDGE('',*,*,#16154,.F.);
#22393=ORIENTED_EDGE('',*,*,#16303,.T.);
#22394=ORIENTED_EDGE('',*,*,#16305,.T.);
#22395=ORIENTED_EDGE('',*,*,#15284,.F.);
#22396=ORIENTED_EDGE('',*,*,#15285,.F.);
#22397=ORIENTED_EDGE('',*,*,#16305,.F.);
#22398=ORIENTED_EDGE('',*,*,#16302,.F.);
#22399=ORIENTED_EDGE('',*,*,#16304,.F.);
#22400=ORIENTED_EDGE('',*,*,#15526,.F.);
#22401=ORIENTED_EDGE('',*,*,#15808,.F.);
#22402=ORIENTED_EDGE('',*,*,#15809,.F.);
#22403=ORIENTED_EDGE('',*,*,#15802,.F.);
#22404=ORIENTED_EDGE('',*,*,#16144,.F.);
#22405=ORIENTED_EDGE('',*,*,#15280,.F.);
#22406=ORIENTED_EDGE('',*,*,#16306,.T.);
#22407=ORIENTED_EDGE('',*,*,#16148,.F.);
#22408=ORIENTED_EDGE('',*,*,#15279,.F.);
#22409=ORIENTED_EDGE('',*,*,#16147,.F.);
#22410=ORIENTED_EDGE('',*,*,#16149,.F.);
#22411=ORIENTED_EDGE('',*,*,#16306,.F.);
#22412=ORIENTED_EDGE('',*,*,#15532,.F.);
#22413=ORIENTED_EDGE('',*,*,#15796,.F.);
#22414=ORIENTED_EDGE('',*,*,#15798,.F.);
#22415=ORIENTED_EDGE('',*,*,#15799,.F.);
#22416=ORIENTED_EDGE('',*,*,#16137,.F.);
#22417=ORIENTED_EDGE('',*,*,#16307,.T.);
#22418=ORIENTED_EDGE('',*,*,#16308,.T.);
#22419=ORIENTED_EDGE('',*,*,#16309,.F.);
#22420=ORIENTED_EDGE('',*,*,#16139,.F.);
#22421=ORIENTED_EDGE('',*,*,#15274,.F.);
#22422=ORIENTED_EDGE('',*,*,#16310,.T.);
#22423=ORIENTED_EDGE('',*,*,#16307,.F.);
#22424=ORIENTED_EDGE('',*,*,#16140,.F.);
#22425=ORIENTED_EDGE('',*,*,#16309,.T.);
#22426=ORIENTED_EDGE('',*,*,#16311,.T.);
#22427=ORIENTED_EDGE('',*,*,#15272,.F.);
#22428=ORIENTED_EDGE('',*,*,#15273,.F.);
#22429=ORIENTED_EDGE('',*,*,#16311,.F.);
#22430=ORIENTED_EDGE('',*,*,#16308,.F.);
#22431=ORIENTED_EDGE('',*,*,#16310,.F.);
#22432=ORIENTED_EDGE('',*,*,#15538,.F.);
#22433=ORIENTED_EDGE('',*,*,#15786,.F.);
#22434=ORIENTED_EDGE('',*,*,#15788,.F.);
#22435=ORIENTED_EDGE('',*,*,#15789,.F.);
#22436=ORIENTED_EDGE('',*,*,#16130,.F.);
#22437=ORIENTED_EDGE('',*,*,#15268,.F.);
#22438=ORIENTED_EDGE('',*,*,#16312,.T.);
#22439=ORIENTED_EDGE('',*,*,#16134,.F.);
#22440=ORIENTED_EDGE('',*,*,#15267,.F.);
#22441=ORIENTED_EDGE('',*,*,#16133,.F.);
#22442=ORIENTED_EDGE('',*,*,#16135,.F.);
#22443=ORIENTED_EDGE('',*,*,#16312,.F.);
#22444=ORIENTED_EDGE('',*,*,#15544,.F.);
#22445=ORIENTED_EDGE('',*,*,#15776,.F.);
#22446=ORIENTED_EDGE('',*,*,#15778,.F.);
#22447=ORIENTED_EDGE('',*,*,#15779,.F.);
#22448=ORIENTED_EDGE('',*,*,#16123,.F.);
#22449=ORIENTED_EDGE('',*,*,#16313,.T.);
#22450=ORIENTED_EDGE('',*,*,#16314,.T.);
#22451=ORIENTED_EDGE('',*,*,#16315,.F.);
#22452=ORIENTED_EDGE('',*,*,#16125,.F.);
#22453=ORIENTED_EDGE('',*,*,#15262,.F.);
#22454=ORIENTED_EDGE('',*,*,#16316,.T.);
#22455=ORIENTED_EDGE('',*,*,#16313,.F.);
#22456=ORIENTED_EDGE('',*,*,#16126,.F.);
#22457=ORIENTED_EDGE('',*,*,#16315,.T.);
#22458=ORIENTED_EDGE('',*,*,#16317,.T.);
#22459=ORIENTED_EDGE('',*,*,#15260,.F.);
#22460=ORIENTED_EDGE('',*,*,#15261,.F.);
#22461=ORIENTED_EDGE('',*,*,#16317,.F.);
#22462=ORIENTED_EDGE('',*,*,#16314,.F.);
#22463=ORIENTED_EDGE('',*,*,#16316,.F.);
#22464=ORIENTED_EDGE('',*,*,#15550,.F.);
#22465=ORIENTED_EDGE('',*,*,#15766,.F.);
#22466=ORIENTED_EDGE('',*,*,#15768,.F.);
#22467=ORIENTED_EDGE('',*,*,#15769,.F.);
#22468=ORIENTED_EDGE('',*,*,#16116,.F.);
#22469=ORIENTED_EDGE('',*,*,#15256,.F.);
#22470=ORIENTED_EDGE('',*,*,#16318,.T.);
#22471=ORIENTED_EDGE('',*,*,#16120,.F.);
#22472=ORIENTED_EDGE('',*,*,#15255,.F.);
#22473=ORIENTED_EDGE('',*,*,#16119,.F.);
#22474=ORIENTED_EDGE('',*,*,#16121,.F.);
#22475=ORIENTED_EDGE('',*,*,#16318,.F.);
#22476=ORIENTED_EDGE('',*,*,#15556,.F.);
#22477=ORIENTED_EDGE('',*,*,#15756,.F.);
#22478=ORIENTED_EDGE('',*,*,#15758,.F.);
#22479=ORIENTED_EDGE('',*,*,#15759,.F.);
#22480=ORIENTED_EDGE('',*,*,#16109,.F.);
#22481=ORIENTED_EDGE('',*,*,#16319,.T.);
#22482=ORIENTED_EDGE('',*,*,#16320,.T.);
#22483=ORIENTED_EDGE('',*,*,#16321,.F.);
#22484=ORIENTED_EDGE('',*,*,#16111,.F.);
#22485=ORIENTED_EDGE('',*,*,#15250,.F.);
#22486=ORIENTED_EDGE('',*,*,#16322,.T.);
#22487=ORIENTED_EDGE('',*,*,#16319,.F.);
#22488=ORIENTED_EDGE('',*,*,#16112,.F.);
#22489=ORIENTED_EDGE('',*,*,#16321,.T.);
#22490=ORIENTED_EDGE('',*,*,#16323,.T.);
#22491=ORIENTED_EDGE('',*,*,#15248,.F.);
#22492=ORIENTED_EDGE('',*,*,#15249,.F.);
#22493=ORIENTED_EDGE('',*,*,#16323,.F.);
#22494=ORIENTED_EDGE('',*,*,#16320,.F.);
#22495=ORIENTED_EDGE('',*,*,#16322,.F.);
#22496=ORIENTED_EDGE('',*,*,#15562,.F.);
#22497=ORIENTED_EDGE('',*,*,#15746,.F.);
#22498=ORIENTED_EDGE('',*,*,#15748,.F.);
#22499=ORIENTED_EDGE('',*,*,#15749,.F.);
#22500=ORIENTED_EDGE('',*,*,#16102,.F.);
#22501=ORIENTED_EDGE('',*,*,#15244,.F.);
#22502=ORIENTED_EDGE('',*,*,#16324,.T.);
#22503=ORIENTED_EDGE('',*,*,#16106,.F.);
#22504=ORIENTED_EDGE('',*,*,#15243,.F.);
#22505=ORIENTED_EDGE('',*,*,#16105,.F.);
#22506=ORIENTED_EDGE('',*,*,#16107,.F.);
#22507=ORIENTED_EDGE('',*,*,#16324,.F.);
#22508=ORIENTED_EDGE('',*,*,#15739,.F.);
#22509=ORIENTED_EDGE('',*,*,#15738,.T.);
#22510=ORIENTED_EDGE('',*,*,#16325,.T.);
#22511=ORIENTED_EDGE('',*,*,#15567,.F.);
#22512=ORIENTED_EDGE('',*,*,#15568,.F.);
#22513=ORIENTED_EDGE('',*,*,#16325,.F.);
#22514=ORIENTED_EDGE('',*,*,#15737,.F.);
#22515=ORIENTED_EDGE('',*,*,#15206,.F.);
#22516=ORIENTED_EDGE('',*,*,#16095,.F.);
#22517=ORIENTED_EDGE('',*,*,#16326,.T.);
#22518=ORIENTED_EDGE('',*,*,#16327,.T.);
#22519=ORIENTED_EDGE('',*,*,#16328,.F.);
#22520=ORIENTED_EDGE('',*,*,#16097,.F.);
#22521=ORIENTED_EDGE('',*,*,#15238,.F.);
#22522=ORIENTED_EDGE('',*,*,#16329,.T.);
#22523=ORIENTED_EDGE('',*,*,#16326,.F.);
#22524=ORIENTED_EDGE('',*,*,#16098,.F.);
#22525=ORIENTED_EDGE('',*,*,#16328,.T.);
#22526=ORIENTED_EDGE('',*,*,#16330,.T.);
#22527=ORIENTED_EDGE('',*,*,#15236,.F.);
#22528=ORIENTED_EDGE('',*,*,#15237,.F.);
#22529=ORIENTED_EDGE('',*,*,#16330,.F.);
#22530=ORIENTED_EDGE('',*,*,#16327,.F.);
#22531=ORIENTED_EDGE('',*,*,#16329,.F.);
#22532=ORIENTED_EDGE('',*,*,#15211,.F.);
#22533=ORIENTED_EDGE('',*,*,#15578,.F.);
#22534=ORIENTED_EDGE('',*,*,#15580,.F.);
#22535=ORIENTED_EDGE('',*,*,#15581,.F.);
#22536=ORIENTED_EDGE('',*,*,#16088,.F.);
#22537=ORIENTED_EDGE('',*,*,#15232,.F.);
#22538=ORIENTED_EDGE('',*,*,#16331,.T.);
#22539=ORIENTED_EDGE('',*,*,#16092,.F.);
#22540=ORIENTED_EDGE('',*,*,#15231,.F.);
#22541=ORIENTED_EDGE('',*,*,#16091,.F.);
#22542=ORIENTED_EDGE('',*,*,#16093,.F.);
#22543=ORIENTED_EDGE('',*,*,#16331,.F.);
#22544=ORIENTED_EDGE('',*,*,#15217,.F.);
#22545=ORIENTED_EDGE('',*,*,#15591,.F.);
#22546=ORIENTED_EDGE('',*,*,#15593,.F.);
#22547=ORIENTED_EDGE('',*,*,#15594,.F.);
#22548=ORIENTED_EDGE('',*,*,#16081,.F.);
#22549=ORIENTED_EDGE('',*,*,#16332,.T.);
#22550=ORIENTED_EDGE('',*,*,#16333,.T.);
#22551=ORIENTED_EDGE('',*,*,#16334,.F.);
#22552=ORIENTED_EDGE('',*,*,#16083,.F.);
#22553=ORIENTED_EDGE('',*,*,#15226,.F.);
#22554=ORIENTED_EDGE('',*,*,#16335,.T.);
#22555=ORIENTED_EDGE('',*,*,#16332,.F.);
#22556=ORIENTED_EDGE('',*,*,#16084,.F.);
#22557=ORIENTED_EDGE('',*,*,#16334,.T.);
#22558=ORIENTED_EDGE('',*,*,#16336,.T.);
#22559=ORIENTED_EDGE('',*,*,#15224,.F.);
#22560=ORIENTED_EDGE('',*,*,#15225,.F.);
#22561=ORIENTED_EDGE('',*,*,#16336,.F.);
#22562=ORIENTED_EDGE('',*,*,#16333,.F.);
#22563=ORIENTED_EDGE('',*,*,#16335,.F.);
#22564=ORIENTED_EDGE('',*,*,#15406,.F.);
#22565=ORIENTED_EDGE('',*,*,#15604,.F.);
#22566=ORIENTED_EDGE('',*,*,#15606,.F.);
#22567=ORIENTED_EDGE('',*,*,#15607,.F.);
#22568=ORIENTED_EDGE('',*,*,#16077,.F.);
#22569=ORIENTED_EDGE('',*,*,#16337,.T.);
#22570=ORIENTED_EDGE('',*,*,#16338,.T.);
#22571=ORIENTED_EDGE('',*,*,#16339,.F.);
#22572=ORIENTED_EDGE('',*,*,#16079,.F.);
#22573=ORIENTED_EDGE('',*,*,#15400,.F.);
#22574=ORIENTED_EDGE('',*,*,#16340,.T.);
#22575=ORIENTED_EDGE('',*,*,#16337,.F.);
#22576=ORIENTED_EDGE('',*,*,#16076,.F.);
#22577=ORIENTED_EDGE('',*,*,#16339,.T.);
#22578=ORIENTED_EDGE('',*,*,#16341,.T.);
#22579=ORIENTED_EDGE('',*,*,#15398,.F.);
#22580=ORIENTED_EDGE('',*,*,#15399,.F.);
#22581=ORIENTED_EDGE('',*,*,#16341,.F.);
#22582=ORIENTED_EDGE('',*,*,#16338,.F.);
#22583=ORIENTED_EDGE('',*,*,#16340,.F.);
#22584=ORIENTED_EDGE('',*,*,#15412,.F.);
#22585=ORIENTED_EDGE('',*,*,#15615,.F.);
#22586=ORIENTED_EDGE('',*,*,#15617,.F.);
#22587=ORIENTED_EDGE('',*,*,#16342,.F.);
#22588=ORIENTED_EDGE('',*,*,#15618,.F.);
#22589=ORIENTED_EDGE('',*,*,#15413,.F.);
#22590=ORIENTED_EDGE('',*,*,#16342,.T.);
#22591=ORIENTED_EDGE('',*,*,#15616,.F.);
#22592=ORIENTED_EDGE('',*,*,#16069,.F.);
#22593=ORIENTED_EDGE('',*,*,#15394,.F.);
#22594=ORIENTED_EDGE('',*,*,#16343,.T.);
#22595=ORIENTED_EDGE('',*,*,#16073,.F.);
#22596=ORIENTED_EDGE('',*,*,#15393,.F.);
#22597=ORIENTED_EDGE('',*,*,#16072,.F.);
#22598=ORIENTED_EDGE('',*,*,#16074,.F.);
#22599=ORIENTED_EDGE('',*,*,#16343,.F.);
#22600=ORIENTED_EDGE('',*,*,#15705,.F.);
#22601=ORIENTED_EDGE('',*,*,#16344,.T.);
#22602=ORIENTED_EDGE('',*,*,#16345,.T.);
#22603=ORIENTED_EDGE('',*,*,#15417,.F.);
#22604=ORIENTED_EDGE('',*,*,#15418,.F.);
#22605=ORIENTED_EDGE('',*,*,#16345,.F.);
#22606=ORIENTED_EDGE('',*,*,#16346,.F.);
#22607=ORIENTED_EDGE('',*,*,#16347,.F.);
#22608=ORIENTED_EDGE('',*,*,#15708,.F.);
#22609=ORIENTED_EDGE('',*,*,#16348,.T.);
#22610=ORIENTED_EDGE('',*,*,#16346,.T.);
#22611=ORIENTED_EDGE('',*,*,#16344,.F.);
#22612=ORIENTED_EDGE('',*,*,#15709,.F.);
#22613=ORIENTED_EDGE('',*,*,#15419,.F.);
#22614=ORIENTED_EDGE('',*,*,#16347,.T.);
#22615=ORIENTED_EDGE('',*,*,#16348,.F.);
#22616=ORIENTED_EDGE('',*,*,#16062,.F.);
#22617=ORIENTED_EDGE('',*,*,#16349,.T.);
#22618=ORIENTED_EDGE('',*,*,#16350,.T.);
#22619=ORIENTED_EDGE('',*,*,#16351,.F.);
#22620=ORIENTED_EDGE('',*,*,#16064,.F.);
#22621=ORIENTED_EDGE('',*,*,#15388,.F.);
#22622=ORIENTED_EDGE('',*,*,#16352,.T.);
#22623=ORIENTED_EDGE('',*,*,#16349,.F.);
#22624=ORIENTED_EDGE('',*,*,#16065,.F.);
#22625=ORIENTED_EDGE('',*,*,#16351,.T.);
#22626=ORIENTED_EDGE('',*,*,#16353,.T.);
#22627=ORIENTED_EDGE('',*,*,#15386,.F.);
#22628=ORIENTED_EDGE('',*,*,#15387,.F.);
#22629=ORIENTED_EDGE('',*,*,#16353,.F.);
#22630=ORIENTED_EDGE('',*,*,#16350,.F.);
#22631=ORIENTED_EDGE('',*,*,#16352,.F.);
#22632=ORIENTED_EDGE('',*,*,#15710,.F.);
#22633=ORIENTED_EDGE('',*,*,#16354,.T.);
#22634=ORIENTED_EDGE('',*,*,#16355,.T.);
#22635=ORIENTED_EDGE('',*,*,#15423,.F.);
#22636=ORIENTED_EDGE('',*,*,#15424,.F.);
#22637=ORIENTED_EDGE('',*,*,#16355,.F.);
#22638=ORIENTED_EDGE('',*,*,#16356,.F.);
#22639=ORIENTED_EDGE('',*,*,#16357,.F.);
#22640=ORIENTED_EDGE('',*,*,#15713,.F.);
#22641=ORIENTED_EDGE('',*,*,#16358,.T.);
#22642=ORIENTED_EDGE('',*,*,#16356,.T.);
#22643=ORIENTED_EDGE('',*,*,#16354,.F.);
#22644=ORIENTED_EDGE('',*,*,#15714,.F.);
#22645=ORIENTED_EDGE('',*,*,#15425,.F.);
#22646=ORIENTED_EDGE('',*,*,#16357,.T.);
#22647=ORIENTED_EDGE('',*,*,#16358,.F.);
#22648=ORIENTED_EDGE('',*,*,#16055,.F.);
#22649=ORIENTED_EDGE('',*,*,#15382,.F.);
#22650=ORIENTED_EDGE('',*,*,#16359,.T.);
#22651=ORIENTED_EDGE('',*,*,#16059,.F.);
#22652=ORIENTED_EDGE('',*,*,#15381,.F.);
#22653=ORIENTED_EDGE('',*,*,#16058,.F.);
#22654=ORIENTED_EDGE('',*,*,#16060,.F.);
#22655=ORIENTED_EDGE('',*,*,#16359,.F.);
#22656=ORIENTED_EDGE('',*,*,#15715,.F.);
#22657=ORIENTED_EDGE('',*,*,#16360,.T.);
#22658=ORIENTED_EDGE('',*,*,#16361,.T.);
#22659=ORIENTED_EDGE('',*,*,#15429,.F.);
#22660=ORIENTED_EDGE('',*,*,#15430,.F.);
#22661=ORIENTED_EDGE('',*,*,#16361,.F.);
#22662=ORIENTED_EDGE('',*,*,#16362,.F.);
#22663=ORIENTED_EDGE('',*,*,#16363,.F.);
#22664=ORIENTED_EDGE('',*,*,#15718,.F.);
#22665=ORIENTED_EDGE('',*,*,#16364,.T.);
#22666=ORIENTED_EDGE('',*,*,#16362,.T.);
#22667=ORIENTED_EDGE('',*,*,#16360,.F.);
#22668=ORIENTED_EDGE('',*,*,#15719,.F.);
#22669=ORIENTED_EDGE('',*,*,#15431,.F.);
#22670=ORIENTED_EDGE('',*,*,#16363,.T.);
#22671=ORIENTED_EDGE('',*,*,#16364,.F.);
#22672=ORIENTED_EDGE('',*,*,#16048,.F.);
#22673=ORIENTED_EDGE('',*,*,#16365,.T.);
#22674=ORIENTED_EDGE('',*,*,#16366,.T.);
#22675=ORIENTED_EDGE('',*,*,#16367,.F.);
#22676=ORIENTED_EDGE('',*,*,#16050,.F.);
#22677=ORIENTED_EDGE('',*,*,#15376,.F.);
#22678=ORIENTED_EDGE('',*,*,#16368,.T.);
#22679=ORIENTED_EDGE('',*,*,#16365,.F.);
#22680=ORIENTED_EDGE('',*,*,#16051,.F.);
#22681=ORIENTED_EDGE('',*,*,#16367,.T.);
#22682=ORIENTED_EDGE('',*,*,#16369,.T.);
#22683=ORIENTED_EDGE('',*,*,#15374,.F.);
#22684=ORIENTED_EDGE('',*,*,#15375,.F.);
#22685=ORIENTED_EDGE('',*,*,#16369,.F.);
#22686=ORIENTED_EDGE('',*,*,#16366,.F.);
#22687=ORIENTED_EDGE('',*,*,#16368,.F.);
#22688=ORIENTED_EDGE('',*,*,#15720,.F.);
#22689=ORIENTED_EDGE('',*,*,#16370,.T.);
#22690=ORIENTED_EDGE('',*,*,#16371,.T.);
#22691=ORIENTED_EDGE('',*,*,#15435,.F.);
#22692=ORIENTED_EDGE('',*,*,#15436,.F.);
#22693=ORIENTED_EDGE('',*,*,#16371,.F.);
#22694=ORIENTED_EDGE('',*,*,#16372,.F.);
#22695=ORIENTED_EDGE('',*,*,#16373,.F.);
#22696=ORIENTED_EDGE('',*,*,#15723,.F.);
#22697=ORIENTED_EDGE('',*,*,#16374,.T.);
#22698=ORIENTED_EDGE('',*,*,#16372,.T.);
#22699=ORIENTED_EDGE('',*,*,#16370,.F.);
#22700=ORIENTED_EDGE('',*,*,#15724,.F.);
#22701=ORIENTED_EDGE('',*,*,#15437,.F.);
#22702=ORIENTED_EDGE('',*,*,#16373,.T.);
#22703=ORIENTED_EDGE('',*,*,#16374,.F.);
#22704=ORIENTED_EDGE('',*,*,#16041,.F.);
#22705=ORIENTED_EDGE('',*,*,#15370,.F.);
#22706=ORIENTED_EDGE('',*,*,#16375,.T.);
#22707=ORIENTED_EDGE('',*,*,#16045,.F.);
#22708=ORIENTED_EDGE('',*,*,#15369,.F.);
#22709=ORIENTED_EDGE('',*,*,#16044,.F.);
#22710=ORIENTED_EDGE('',*,*,#16046,.F.);
#22711=ORIENTED_EDGE('',*,*,#16375,.F.);
#22712=ORIENTED_EDGE('',*,*,#15725,.F.);
#22713=ORIENTED_EDGE('',*,*,#16376,.T.);
#22714=ORIENTED_EDGE('',*,*,#16377,.T.);
#22715=ORIENTED_EDGE('',*,*,#15441,.F.);
#22716=ORIENTED_EDGE('',*,*,#15442,.F.);
#22717=ORIENTED_EDGE('',*,*,#16377,.F.);
#22718=ORIENTED_EDGE('',*,*,#16378,.F.);
#22719=ORIENTED_EDGE('',*,*,#16379,.F.);
#22720=ORIENTED_EDGE('',*,*,#15728,.F.);
#22721=ORIENTED_EDGE('',*,*,#16380,.T.);
#22722=ORIENTED_EDGE('',*,*,#16378,.T.);
#22723=ORIENTED_EDGE('',*,*,#16376,.F.);
#22724=ORIENTED_EDGE('',*,*,#15729,.F.);
#22725=ORIENTED_EDGE('',*,*,#15443,.F.);
#22726=ORIENTED_EDGE('',*,*,#16379,.T.);
#22727=ORIENTED_EDGE('',*,*,#16380,.F.);
#22728=ORIENTED_EDGE('',*,*,#16034,.F.);
#22729=ORIENTED_EDGE('',*,*,#16381,.T.);
#22730=ORIENTED_EDGE('',*,*,#16382,.T.);
#22731=ORIENTED_EDGE('',*,*,#16383,.F.);
#22732=ORIENTED_EDGE('',*,*,#16036,.F.);
#22733=ORIENTED_EDGE('',*,*,#15364,.F.);
#22734=ORIENTED_EDGE('',*,*,#16384,.T.);
#22735=ORIENTED_EDGE('',*,*,#16381,.F.);
#22736=ORIENTED_EDGE('',*,*,#16037,.F.);
#22737=ORIENTED_EDGE('',*,*,#16383,.T.);
#22738=ORIENTED_EDGE('',*,*,#16385,.T.);
#22739=ORIENTED_EDGE('',*,*,#15362,.F.);
#22740=ORIENTED_EDGE('',*,*,#15363,.F.);
#22741=ORIENTED_EDGE('',*,*,#16385,.F.);
#22742=ORIENTED_EDGE('',*,*,#16382,.F.);
#22743=ORIENTED_EDGE('',*,*,#16384,.F.);
#22744=ORIENTED_EDGE('',*,*,#15730,.F.);
#22745=ORIENTED_EDGE('',*,*,#16386,.T.);
#22746=ORIENTED_EDGE('',*,*,#16387,.T.);
#22747=ORIENTED_EDGE('',*,*,#15447,.F.);
#22748=ORIENTED_EDGE('',*,*,#15448,.F.);
#22749=ORIENTED_EDGE('',*,*,#16387,.F.);
#22750=ORIENTED_EDGE('',*,*,#16388,.F.);
#22751=ORIENTED_EDGE('',*,*,#16389,.F.);
#22752=ORIENTED_EDGE('',*,*,#15733,.F.);
#22753=ORIENTED_EDGE('',*,*,#16390,.T.);
#22754=ORIENTED_EDGE('',*,*,#16388,.T.);
#22755=ORIENTED_EDGE('',*,*,#16386,.F.);
#22756=ORIENTED_EDGE('',*,*,#15734,.F.);
#22757=ORIENTED_EDGE('',*,*,#15449,.F.);
#22758=ORIENTED_EDGE('',*,*,#16389,.T.);
#22759=ORIENTED_EDGE('',*,*,#16390,.F.);
#22760=ORIENTED_EDGE('',*,*,#15357,.F.);
#22761=ORIENTED_EDGE('',*,*,#16391,.F.);
#22762=ORIENTED_EDGE('',*,*,#16392,.F.);
#22763=ORIENTED_EDGE('',*,*,#16393,.F.);
#22764=ORIENTED_EDGE('',*,*,#16032,.F.);
#22765=ORIENTED_EDGE('',*,*,#15358,.F.);
#22766=ORIENTED_EDGE('',*,*,#16393,.T.);
#22767=ORIENTED_EDGE('',*,*,#16394,.F.);
#22768=ORIENTED_EDGE('',*,*,#15932,.F.);
#22769=ORIENTED_EDGE('',*,*,#16394,.T.);
#22770=ORIENTED_EDGE('',*,*,#16392,.T.);
#22771=ORIENTED_EDGE('',*,*,#16395,.F.);
#22772=ORIENTED_EDGE('',*,*,#15934,.F.);
#22773=ORIENTED_EDGE('',*,*,#16395,.T.);
#22774=ORIENTED_EDGE('',*,*,#16391,.T.);
#22775=ORIENTED_EDGE('',*,*,#15356,.F.);
#22776=ORIENTED_EDGE('',*,*,#16236,.F.);
#22777=ORIENTED_EDGE('',*,*,#16239,.T.);
#22778=ORIENTED_EDGE('',*,*,#16250,.F.);
#22779=ORIENTED_EDGE('',*,*,#16031,.F.);
#22780=ORIENTED_EDGE('',*,*,#16252,.F.);
#22781=ORIENTED_EDGE('',*,*,#16259,.T.);
#22782=ORIENTED_EDGE('',*,*,#16263,.F.);
#22783=ORIENTED_EDGE('',*,*,#15698,.T.);
#26173=ADVANCED_FACE('',(#7349),#929,.T.);
#26174=ADVANCED_FACE('',(#7350),#930,.F.);
#26175=ADVANCED_FACE('',(#7351),#6672,.T.);
#26176=ADVANCED_FACE('',(#7352),#931,.T.);
#26177=ADVANCED_FACE('',(#7353),#932,.T.);
#26178=ADVANCED_FACE('',(#7354),#933,.T.);
#26179=ADVANCED_FACE('',(#7355),#934,.F.);
#26180=ADVANCED_FACE('',(#7356),#935,.F.);
#26181=ADVANCED_FACE('',(#7357),#936,.F.);
#26182=ADVANCED_FACE('',(#7358),#937,.T.);
#26183=ADVANCED_FACE('',(#7359),#938,.T.);
#26184=ADVANCED_FACE('',(#7360),#939,.T.);
#26185=ADVANCED_FACE('',(#7361),#940,.F.);
#26186=ADVANCED_FACE('',(#7362),#941,.F.);
#26187=ADVANCED_FACE('',(#7363),#942,.F.);
#26188=ADVANCED_FACE('',(#7364),#943,.T.);
#26189=ADVANCED_FACE('',(#7365),#944,.T.);
#26190=ADVANCED_FACE('',(#7366),#945,.T.);
#26191=ADVANCED_FACE('',(#7367),#946,.F.);
#26192=ADVANCED_FACE('',(#7368),#947,.F.);
#26193=ADVANCED_FACE('',(#7369),#948,.F.);
#26194=ADVANCED_FACE('',(#7370),#949,.T.);
#26195=ADVANCED_FACE('',(#7371),#950,.T.);
#26196=ADVANCED_FACE('',(#7372),#951,.F.);
#26197=ADVANCED_FACE('',(#7373),#952,.F.);
#26198=ADVANCED_FACE('',(#7374),#953,.T.);
#26199=ADVANCED_FACE('',(#7375,#681),#954,.T.);
#26200=ADVANCED_FACE('',(#7376),#955,.T.);
#26201=ADVANCED_FACE('',(#7377),#956,.T.);
#26202=ADVANCED_FACE('',(#7378),#957,.T.);
#26203=ADVANCED_FACE('',(#7379),#958,.T.);
#26204=ADVANCED_FACE('',(#7380),#959,.T.);
#26205=ADVANCED_FACE('',(#7381),#960,.T.);
#26206=ADVANCED_FACE('',(#7382),#961,.T.);
#26207=ADVANCED_FACE('',(#7383),#962,.T.);
#26208=ADVANCED_FACE('',(#7384),#963,.T.);
#26209=ADVANCED_FACE('',(#7385),#964,.T.);
#26210=ADVANCED_FACE('',(#7386),#965,.T.);
#26211=ADVANCED_FACE('',(#7387),#966,.T.);
#26212=ADVANCED_FACE('',(#7388),#967,.T.);
#26213=ADVANCED_FACE('',(#7389),#968,.T.);
#26214=ADVANCED_FACE('',(#7390),#969,.T.);
#26215=ADVANCED_FACE('',(#7391),#970,.T.);
#26216=ADVANCED_FACE('',(#7392),#971,.T.);
#26217=ADVANCED_FACE('',(#7393),#972,.T.);
#26218=ADVANCED_FACE('',(#7394),#973,.T.);
#26219=ADVANCED_FACE('',(#7395),#974,.F.);
#26220=ADVANCED_FACE('',(#7396),#975,.T.);
#26221=ADVANCED_FACE('',(#7397),#976,.T.);
#26222=ADVANCED_FACE('',(#7398),#977,.T.);
#26223=ADVANCED_FACE('',(#7399),#978,.T.);
#26224=ADVANCED_FACE('',(#7400),#979,.F.);
#26225=ADVANCED_FACE('',(#7401),#980,.F.);
#26226=ADVANCED_FACE('',(#7402),#981,.F.);
#26227=ADVANCED_FACE('',(#7403),#982,.T.);
#26228=ADVANCED_FACE('',(#7404),#983,.T.);
#26229=ADVANCED_FACE('',(#7405),#984,.T.);
#26230=ADVANCED_FACE('',(#7406),#985,.F.);
#26231=ADVANCED_FACE('',(#7407),#986,.F.);
#26232=ADVANCED_FACE('',(#7408),#987,.F.);
#26233=ADVANCED_FACE('',(#7409),#988,.T.);
#26234=ADVANCED_FACE('',(#7410),#989,.T.);
#26235=ADVANCED_FACE('',(#7411),#990,.T.);
#26236=ADVANCED_FACE('',(#7412),#991,.F.);
#26237=ADVANCED_FACE('',(#7413),#992,.F.);
#26238=ADVANCED_FACE('',(#7414),#993,.F.);
#26239=ADVANCED_FACE('',(#7415),#994,.T.);
#26240=ADVANCED_FACE('',(#7416),#995,.T.);
#26241=ADVANCED_FACE('',(#7417),#996,.T.);
#26242=ADVANCED_FACE('',(#7418),#997,.F.);
#26243=ADVANCED_FACE('',(#7419),#998,.F.);
#26244=ADVANCED_FACE('',(#7420),#999,.F.);
#26245=ADVANCED_FACE('',(#7421),#1000,.T.);
#26246=ADVANCED_FACE('',(#7422),#1001,.T.);
#26247=ADVANCED_FACE('',(#7423),#1002,.T.);
#26248=ADVANCED_FACE('',(#7424),#1003,.F.);
#26249=ADVANCED_FACE('',(#7425),#1004,.F.);
#26250=ADVANCED_FACE('',(#7426),#1005,.F.);
#26251=ADVANCED_FACE('',(#7427),#1006,.T.);
#26252=ADVANCED_FACE('',(#7428),#1007,.T.);
#26253=ADVANCED_FACE('',(#7429),#1008,.T.);
#26254=ADVANCED_FACE('',(#7430),#1009,.F.);
#26255=ADVANCED_FACE('',(#7431),#1010,.F.);
#26256=ADVANCED_FACE('',(#7432),#1011,.F.);
#26257=ADVANCED_FACE('',(#7433),#1012,.T.);
#26258=ADVANCED_FACE('',(#7434),#1013,.F.);
#26259=ADVANCED_FACE('',(#7435),#1014,.T.);
#26260=ADVANCED_FACE('',(#7436),#1015,.T.);
#26261=ADVANCED_FACE('',(#7437),#1016,.F.);
#26262=ADVANCED_FACE('',(#7438),#1017,.F.);
#26263=ADVANCED_FACE('',(#7439),#1018,.T.);
#26264=ADVANCED_FACE('',(#7440),#1019,.T.);
#26265=ADVANCED_FACE('',(#7441),#1020,.T.);
#26266=ADVANCED_FACE('',(#7442),#1021,.F.);
#26267=ADVANCED_FACE('',(#7443),#1022,.F.);
#26268=ADVANCED_FACE('',(#7444),#1023,.F.);
#26269=ADVANCED_FACE('',(#7445),#1024,.T.);
#26270=ADVANCED_FACE('',(#7446),#1025,.T.);
#26271=ADVANCED_FACE('',(#7447),#1026,.T.);
#26272=ADVANCED_FACE('',(#7448),#1027,.F.);
#26273=ADVANCED_FACE('',(#7449),#1028,.F.);
#26274=ADVANCED_FACE('',(#7450),#1029,.F.);
#26275=ADVANCED_FACE('',(#7451),#1030,.T.);
#26276=ADVANCED_FACE('',(#7452),#1031,.T.);
#26277=ADVANCED_FACE('',(#7453),#1032,.T.);
#26278=ADVANCED_FACE('',(#7454),#1033,.F.);
#26279=ADVANCED_FACE('',(#7455),#1034,.F.);
#26280=ADVANCED_FACE('',(#7456),#1035,.F.);
#26281=ADVANCED_FACE('',(#7457),#1036,.T.);
#26282=ADVANCED_FACE('',(#7458),#1037,.T.);
#26283=ADVANCED_FACE('',(#7459),#1038,.T.);
#26284=ADVANCED_FACE('',(#7460),#1039,.F.);
#26285=ADVANCED_FACE('',(#7461),#1040,.F.);
#26286=ADVANCED_FACE('',(#7462),#1041,.F.);
#26287=ADVANCED_FACE('',(#7463),#1042,.T.);
#26288=ADVANCED_FACE('',(#7464),#1043,.T.);
#26289=ADVANCED_FACE('',(#7465),#1044,.T.);
#26290=ADVANCED_FACE('',(#7466),#1045,.F.);
#26291=ADVANCED_FACE('',(#7467),#1046,.F.);
#26292=ADVANCED_FACE('',(#7468),#1047,.F.);
#26293=ADVANCED_FACE('',(#7469),#1048,.T.);
#26294=ADVANCED_FACE('',(#7470),#1049,.T.);
#26295=ADVANCED_FACE('',(#7471),#1050,.T.);
#26296=ADVANCED_FACE('',(#7472),#1051,.F.);
#26297=ADVANCED_FACE('',(#7473),#1052,.F.);
#26298=ADVANCED_FACE('',(#7474),#1053,.F.);
#26299=ADVANCED_FACE('',(#7475),#1054,.T.);
#26300=ADVANCED_FACE('',(#7476),#1055,.T.);
#26301=ADVANCED_FACE('',(#7477),#1056,.T.);
#26302=ADVANCED_FACE('',(#7478),#1057,.F.);
#26303=ADVANCED_FACE('',(#7479),#1058,.F.);
#26304=ADVANCED_FACE('',(#7480),#1059,.F.);
#26305=ADVANCED_FACE('',(#7481),#1060,.T.);
#26306=ADVANCED_FACE('',(#7482),#1061,.T.);
#26307=ADVANCED_FACE('',(#7483),#1062,.T.);
#26308=ADVANCED_FACE('',(#7484),#1063,.F.);
#26309=ADVANCED_FACE('',(#7485),#1064,.F.);
#26310=ADVANCED_FACE('',(#7486),#1065,.F.);
#26311=ADVANCED_FACE('',(#7487),#1066,.T.);
#26312=ADVANCED_FACE('',(#7488),#1067,.T.);
#26313=ADVANCED_FACE('',(#7489),#1068,.T.);
#26314=ADVANCED_FACE('',(#7490),#1069,.F.);
#26315=ADVANCED_FACE('',(#7491),#1070,.F.);
#26316=ADVANCED_FACE('',(#7492),#1071,.F.);
#26317=ADVANCED_FACE('',(#7493),#1072,.T.);
#26318=ADVANCED_FACE('',(#7494),#1073,.T.);
#26319=ADVANCED_FACE('',(#7495),#1074,.T.);
#26320=ADVANCED_FACE('',(#7496),#1075,.F.);
#26321=ADVANCED_FACE('',(#7497),#1076,.F.);
#26322=ADVANCED_FACE('',(#7498),#1077,.F.);
#26323=ADVANCED_FACE('',(#7499),#1078,.T.);
#26324=ADVANCED_FACE('',(#7500),#1079,.T.);
#26325=ADVANCED_FACE('',(#7501),#1080,.T.);
#26326=ADVANCED_FACE('',(#7502),#1081,.F.);
#26327=ADVANCED_FACE('',(#7503),#1082,.F.);
#26328=ADVANCED_FACE('',(#7504),#1083,.F.);
#26329=ADVANCED_FACE('',(#7505),#1084,.T.);
#26330=ADVANCED_FACE('',(#7506),#1085,.T.);
#26331=ADVANCED_FACE('',(#7507),#1086,.T.);
#26332=ADVANCED_FACE('',(#7508),#1087,.F.);
#26333=ADVANCED_FACE('',(#7509),#1088,.F.);
#26334=ADVANCED_FACE('',(#7510),#1089,.F.);
#26335=ADVANCED_FACE('',(#7511),#1090,.T.);
#26336=ADVANCED_FACE('',(#7512),#1091,.T.);
#26337=ADVANCED_FACE('',(#7513,#682),#1092,.T.);
#26338=ADVANCED_FACE('',(#7514),#1093,.T.);
#26339=ADVANCED_FACE('',(#7515),#1094,.T.);
#26340=ADVANCED_FACE('',(#7516),#1095,.T.);
#26341=ADVANCED_FACE('',(#7517),#1096,.T.);
#26342=ADVANCED_FACE('',(#7518),#1097,.T.);
#26343=ADVANCED_FACE('',(#7519),#1098,.T.);
#26344=ADVANCED_FACE('',(#7520),#1099,.T.);
#26345=ADVANCED_FACE('',(#7521),#1100,.F.);
#26346=ADVANCED_FACE('',(#7522),#1101,.F.);
#26347=ADVANCED_FACE('',(#7523),#1102,.T.);
#26348=ADVANCED_FACE('',(#7524),#1103,.T.);
#26349=ADVANCED_FACE('',(#7525),#1104,.T.);
#26350=ADVANCED_FACE('',(#7526),#1105,.T.);
#26351=ADVANCED_FACE('',(#7527),#1106,.T.);
#26352=ADVANCED_FACE('',(#7528),#1107,.T.);
#26353=ADVANCED_FACE('',(#7529),#1108,.F.);
#26354=ADVANCED_FACE('',(#7530),#1109,.F.);
#26355=ADVANCED_FACE('',(#7531),#1110,.T.);
#26356=ADVANCED_FACE('',(#7532),#1111,.T.);
#26357=ADVANCED_FACE('',(#7533),#1112,.T.);
#26358=ADVANCED_FACE('',(#7534),#1113,.T.);
#26359=ADVANCED_FACE('',(#7535),#1114,.T.);
#26360=ADVANCED_FACE('',(#7536),#1115,.T.);
#26361=ADVANCED_FACE('',(#7537),#1116,.F.);
#26362=ADVANCED_FACE('',(#7538),#1117,.F.);
#26363=ADVANCED_FACE('',(#7539),#1118,.T.);
#26364=ADVANCED_FACE('',(#7540),#1119,.T.);
#26365=ADVANCED_FACE('',(#7541),#1120,.T.);
#26366=ADVANCED_FACE('',(#7542),#1121,.T.);
#26367=ADVANCED_FACE('',(#7543),#1122,.T.);
#26368=ADVANCED_FACE('',(#7544),#1123,.T.);
#26369=ADVANCED_FACE('',(#7545),#1124,.T.);
#26370=ADVANCED_FACE('',(#7546),#1125,.T.);
#26371=ADVANCED_FACE('',(#7547),#1126,.T.);
#26372=ADVANCED_FACE('',(#7548),#1127,.F.);
#26373=ADVANCED_FACE('',(#7549),#1128,.F.);
#26374=ADVANCED_FACE('',(#7550),#1129,.T.);
#26375=ADVANCED_FACE('',(#7551),#1130,.T.);
#26376=ADVANCED_FACE('',(#7552),#1131,.T.);
#26377=ADVANCED_FACE('',(#7553),#1132,.T.);
#26378=ADVANCED_FACE('',(#7554),#1133,.T.);
#26379=ADVANCED_FACE('',(#7555),#1134,.T.);
#26380=ADVANCED_FACE('',(#7556),#1135,.F.);
#26381=ADVANCED_FACE('',(#7557),#1136,.F.);
#26382=ADVANCED_FACE('',(#7558),#1137,.T.);
#26383=ADVANCED_FACE('',(#7559),#1138,.T.);
#26384=ADVANCED_FACE('',(#7560),#1139,.T.);
#26385=ADVANCED_FACE('',(#7561),#1140,.T.);
#26386=ADVANCED_FACE('',(#7562),#1141,.T.);
#26387=ADVANCED_FACE('',(#7563),#1142,.T.);
#26388=ADVANCED_FACE('',(#7564),#1143,.F.);
#26389=ADVANCED_FACE('',(#7565),#1144,.F.);
#26390=ADVANCED_FACE('',(#7566),#1145,.T.);
#26391=ADVANCED_FACE('',(#7567),#1146,.T.);
#26392=ADVANCED_FACE('',(#7568),#1147,.T.);
#26393=ADVANCED_FACE('',(#7569),#1148,.T.);
#26394=ADVANCED_FACE('',(#7570),#1149,.T.);
#26395=ADVANCED_FACE('',(#7571),#1150,.T.);
#26396=ADVANCED_FACE('',(#7572),#1151,.F.);
#26397=ADVANCED_FACE('',(#7573),#1152,.F.);
#26398=ADVANCED_FACE('',(#7574),#1153,.T.);
#26399=ADVANCED_FACE('',(#7575),#1154,.T.);
#26400=ADVANCED_FACE('',(#7576),#1155,.T.);
#26401=ADVANCED_FACE('',(#7577),#1156,.T.);
#26402=ADVANCED_FACE('',(#7578),#1157,.T.);
#26403=ADVANCED_FACE('',(#7579),#1158,.T.);
#26404=ADVANCED_FACE('',(#7580),#1159,.F.);
#26405=ADVANCED_FACE('',(#7581),#1160,.F.);
#26406=ADVANCED_FACE('',(#7582),#1161,.T.);
#26407=ADVANCED_FACE('',(#7583),#1162,.T.);
#26408=ADVANCED_FACE('',(#7584),#1163,.T.);
#26409=ADVANCED_FACE('',(#7585),#1164,.T.);
#26410=ADVANCED_FACE('',(#7586),#1165,.T.);
#26411=ADVANCED_FACE('',(#7587),#1166,.T.);
#26412=ADVANCED_FACE('',(#7588),#1167,.F.);
#26413=ADVANCED_FACE('',(#7589),#1168,.F.);
#26414=ADVANCED_FACE('',(#7590),#1169,.T.);
#26415=ADVANCED_FACE('',(#7591),#1170,.T.);
#26416=ADVANCED_FACE('',(#7592),#1171,.T.);
#26417=ADVANCED_FACE('',(#7593),#1172,.T.);
#26418=ADVANCED_FACE('',(#7594),#1173,.T.);
#26419=ADVANCED_FACE('',(#7595),#1174,.T.);
#26420=ADVANCED_FACE('',(#7596),#1175,.T.);
#26421=ADVANCED_FACE('',(#7597),#1176,.T.);
#26422=ADVANCED_FACE('',(#7598),#1177,.T.);
#26423=ADVANCED_FACE('',(#7599),#1178,.F.);
#26424=ADVANCED_FACE('',(#7600),#1179,.F.);
#26425=ADVANCED_FACE('',(#7601),#1180,.T.);
#26426=ADVANCED_FACE('',(#7602),#1181,.T.);
#26427=ADVANCED_FACE('',(#7603),#1182,.T.);
#26428=ADVANCED_FACE('',(#7604),#1183,.T.);
#26429=ADVANCED_FACE('',(#7605),#1184,.T.);
#26430=ADVANCED_FACE('',(#7606),#1185,.T.);
#26431=ADVANCED_FACE('',(#7607),#1186,.F.);
#26432=ADVANCED_FACE('',(#7608),#1187,.F.);
#26433=ADVANCED_FACE('',(#7609),#1188,.T.);
#26434=ADVANCED_FACE('',(#7610),#1189,.T.);
#26435=ADVANCED_FACE('',(#7611),#1190,.T.);
#26436=ADVANCED_FACE('',(#7612),#1191,.T.);
#26437=ADVANCED_FACE('',(#7613),#1192,.T.);
#26438=ADVANCED_FACE('',(#7614),#1193,.T.);
#26439=ADVANCED_FACE('',(#7615),#1194,.F.);
#26440=ADVANCED_FACE('',(#7616),#1195,.F.);
#26441=ADVANCED_FACE('',(#7617),#1196,.T.);
#26442=ADVANCED_FACE('',(#7618),#1197,.T.);
#26443=ADVANCED_FACE('',(#7619),#1198,.T.);
#26444=ADVANCED_FACE('',(#7620),#1199,.T.);
#26445=ADVANCED_FACE('',(#7621),#1200,.T.);
#26446=ADVANCED_FACE('',(#7622),#1201,.T.);
#26447=ADVANCED_FACE('',(#7623),#1202,.T.);
#26448=ADVANCED_FACE('',(#7624),#1203,.T.);
#26449=ADVANCED_FACE('',(#7625),#1204,.T.);
#26450=ADVANCED_FACE('',(#7626),#1205,.F.);
#26451=ADVANCED_FACE('',(#7627),#1206,.F.);
#26452=ADVANCED_FACE('',(#7628),#1207,.T.);
#26453=ADVANCED_FACE('',(#7629),#1208,.T.);
#26454=ADVANCED_FACE('',(#7630),#1209,.T.);
#26455=ADVANCED_FACE('',(#7631),#1210,.F.);
#26456=ADVANCED_FACE('',(#7632),#1211,.F.);
#26457=ADVANCED_FACE('',(#7633),#1212,.F.);
#26458=ADVANCED_FACE('',(#7634),#6673,.F.);
#26459=ADVANCED_FACE('',(#7635),#1213,.T.);
#26460=ADVANCED_FACE('',(#7636),#1214,.T.);
#26461=ADVANCED_FACE('',(#7637),#1215,.T.);
#26462=ADVANCED_FACE('',(#7638),#1216,.T.);
#26463=ADVANCED_FACE('',(#7639),#1217,.T.);
#26464=ADVANCED_FACE('',(#7640),#1218,.T.);
#26465=ADVANCED_FACE('',(#7641),#1219,.F.);
#26466=ADVANCED_FACE('',(#7642),#1220,.F.);
#26467=ADVANCED_FACE('',(#7643),#1221,.F.);
#26468=ADVANCED_FACE('',(#7644),#1222,.T.);
#26469=ADVANCED_FACE('',(#7645),#1223,.T.);
#26470=ADVANCED_FACE('',(#7646),#1224,.T.);
#26471=ADVANCED_FACE('',(#7647),#1225,.F.);
#26472=ADVANCED_FACE('',(#7648),#1226,.F.);
#26473=ADVANCED_FACE('',(#7649),#1227,.F.);
#26474=ADVANCED_FACE('',(#7650),#1228,.F.);
#26475=ADVANCED_FACE('',(#7651),#1229,.F.);
#26476=ADVANCED_FACE('',(#7652),#1230,.F.);
#26477=ADVANCED_FACE('',(#7653),#1231,.F.);
#26478=ADVANCED_FACE('',(#7654),#1232,.F.);
#26479=ADVANCED_FACE('',(#7655),#1233,.F.);
#26480=ADVANCED_FACE('',(#7656),#1234,.F.);
#26481=ADVANCED_FACE('',(#7657),#1235,.F.);
#26482=ADVANCED_FACE('',(#7658),#1236,.F.);
#26483=ADVANCED_FACE('',(#7659),#1237,.F.);
#26484=ADVANCED_FACE('',(#7660),#1238,.F.);
#26485=ADVANCED_FACE('',(#7661),#1239,.F.);
#26486=ADVANCED_FACE('',(#7662),#1240,.F.);
#26487=ADVANCED_FACE('',(#7663),#1241,.F.);
#26488=ADVANCED_FACE('',(#7664),#1242,.F.);
#26489=ADVANCED_FACE('',(#7665),#1243,.F.);
#26490=ADVANCED_FACE('',(#7666),#1244,.F.);
#26491=ADVANCED_FACE('',(#7667),#1245,.F.);
#26492=ADVANCED_FACE('',(#7668),#1246,.F.);
#26493=ADVANCED_FACE('',(#7669),#1247,.F.);
#26494=ADVANCED_FACE('',(#7670),#1248,.F.);
#26495=ADVANCED_FACE('',(#7671),#1249,.F.);
#26496=ADVANCED_FACE('',(#7672),#1250,.F.);
#26497=ADVANCED_FACE('',(#7673),#1251,.F.);
#26498=ADVANCED_FACE('',(#7674),#1252,.F.);
#26499=ADVANCED_FACE('',(#7675),#1253,.F.);
#26500=ADVANCED_FACE('',(#7676),#1254,.F.);
#26501=ADVANCED_FACE('',(#7677),#1255,.F.);
#26502=ADVANCED_FACE('',(#7678),#1256,.F.);
#26503=ADVANCED_FACE('',(#7679),#1257,.F.);
#26504=ADVANCED_FACE('',(#7680),#1258,.F.);
#26505=ADVANCED_FACE('',(#7681),#1259,.F.);
#26506=ADVANCED_FACE('',(#7682),#1260,.F.);
#26507=ADVANCED_FACE('',(#7683),#1261,.F.);
#26508=ADVANCED_FACE('',(#7684),#1262,.F.);
#26509=ADVANCED_FACE('',(#7685),#1263,.F.);
#26510=ADVANCED_FACE('',(#7686),#1264,.F.);
#26511=ADVANCED_FACE('',(#7687),#1265,.F.);
#26512=ADVANCED_FACE('',(#7688),#1266,.F.);
#26513=ADVANCED_FACE('',(#7689),#1267,.F.);
#26514=ADVANCED_FACE('',(#7690),#1268,.F.);
#26515=ADVANCED_FACE('',(#7691),#1269,.F.);
#26516=ADVANCED_FACE('',(#7692),#1270,.F.);
#26517=ADVANCED_FACE('',(#7693),#1271,.F.);
#26518=ADVANCED_FACE('',(#7694),#1272,.F.);
#26519=ADVANCED_FACE('',(#7695),#1273,.F.);
#26520=ADVANCED_FACE('',(#7696),#1274,.F.);
#26521=ADVANCED_FACE('',(#7697),#1275,.F.);
#26522=ADVANCED_FACE('',(#7698),#1276,.F.);
#26523=ADVANCED_FACE('',(#7699),#1277,.F.);
#26524=ADVANCED_FACE('',(#7700),#1278,.F.);
#26525=ADVANCED_FACE('',(#7701),#1279,.F.);
#26526=ADVANCED_FACE('',(#7702),#1280,.F.);
#26527=ADVANCED_FACE('',(#7703),#1281,.F.);
#26528=ADVANCED_FACE('',(#7704),#1282,.F.);
#26529=ADVANCED_FACE('',(#7705),#1283,.F.);
#26530=ADVANCED_FACE('',(#7706),#1284,.F.);
#26531=ADVANCED_FACE('',(#7707),#1285,.F.);
#26532=ADVANCED_FACE('',(#7708),#1286,.F.);
#26533=ADVANCED_FACE('',(#7709),#1287,.F.);
#26534=ADVANCED_FACE('',(#7710),#1288,.F.);
#26535=ADVANCED_FACE('',(#7711),#1289,.F.);
#26536=ADVANCED_FACE('',(#7712),#1290,.F.);
#26537=ADVANCED_FACE('',(#7713),#1291,.F.);
#26538=ADVANCED_FACE('',(#7714),#1292,.F.);
#26539=ADVANCED_FACE('',(#7715),#1293,.F.);
#26540=ADVANCED_FACE('',(#7716),#1294,.F.);
#26541=ADVANCED_FACE('',(#7717),#1295,.F.);
#26542=ADVANCED_FACE('',(#7718),#1296,.F.);
#26543=ADVANCED_FACE('',(#7719),#1297,.F.);
#26544=ADVANCED_FACE('',(#7720),#1298,.F.);
#26545=ADVANCED_FACE('',(#7721),#1299,.F.);
#26546=ADVANCED_FACE('',(#7722),#1300,.F.);
#26547=ADVANCED_FACE('',(#7723),#1301,.F.);
#26548=ADVANCED_FACE('',(#7724),#1302,.F.);
#26549=ADVANCED_FACE('',(#7725),#1303,.F.);
#26550=ADVANCED_FACE('',(#7726),#1304,.F.);
#26551=ADVANCED_FACE('',(#7727),#1305,.F.);
#26552=ADVANCED_FACE('',(#7728),#1306,.F.);
#26553=ADVANCED_FACE('',(#7729),#1307,.F.);
#26554=ADVANCED_FACE('',(#7730),#1308,.F.);
#26555=ADVANCED_FACE('',(#7731),#1309,.F.);
#26556=ADVANCED_FACE('',(#7732),#1310,.F.);
#26557=ADVANCED_FACE('',(#7733),#1311,.F.);
#26558=ADVANCED_FACE('',(#7734),#1312,.F.);
#26559=ADVANCED_FACE('',(#7735),#1313,.F.);
#26560=ADVANCED_FACE('',(#7736),#1314,.F.);
#26561=ADVANCED_FACE('',(#7737),#1315,.F.);
#26562=ADVANCED_FACE('',(#7738),#1316,.F.);
#26563=ADVANCED_FACE('',(#7739),#1317,.F.);
#26564=ADVANCED_FACE('',(#7740),#1318,.F.);
#26565=ADVANCED_FACE('',(#7741),#1319,.F.);
#26566=ADVANCED_FACE('',(#7742),#1320,.F.);
#26567=ADVANCED_FACE('',(#7743),#1321,.F.);
#26568=ADVANCED_FACE('',(#7744),#1322,.F.);
#26569=ADVANCED_FACE('',(#7745),#1323,.F.);
#26570=ADVANCED_FACE('',(#7746),#1324,.F.);
#26571=ADVANCED_FACE('',(#7747),#1325,.F.);
#26572=ADVANCED_FACE('',(#7748),#1326,.F.);
#26573=ADVANCED_FACE('',(#7749),#1327,.F.);
#26574=ADVANCED_FACE('',(#7750),#1328,.F.);
#26575=ADVANCED_FACE('',(#7751),#1329,.F.);
#26576=ADVANCED_FACE('',(#7752),#1330,.F.);
#26577=ADVANCED_FACE('',(#7753),#1331,.F.);
#26578=ADVANCED_FACE('',(#7754),#1332,.F.);
#26579=ADVANCED_FACE('',(#7755),#1333,.F.);
#26580=ADVANCED_FACE('',(#7756),#1334,.F.);
#26581=ADVANCED_FACE('',(#7757),#1335,.F.);
#26582=ADVANCED_FACE('',(#7758),#1336,.F.);
#26583=ADVANCED_FACE('',(#7759),#1337,.F.);
#26584=ADVANCED_FACE('',(#7760),#1338,.F.);
#26585=ADVANCED_FACE('',(#7761),#1339,.F.);
#26586=ADVANCED_FACE('',(#7762),#1340,.F.);
#26587=ADVANCED_FACE('',(#7763),#1341,.F.);
#26588=ADVANCED_FACE('',(#7764),#1342,.F.);
#26589=ADVANCED_FACE('',(#7765),#1343,.F.);
#26590=ADVANCED_FACE('',(#7766),#1344,.F.);
#26591=ADVANCED_FACE('',(#7767),#1345,.F.);
#26592=ADVANCED_FACE('',(#7768),#1346,.F.);
#26593=ADVANCED_FACE('',(#7769),#1347,.F.);
#26594=ADVANCED_FACE('',(#7770),#1348,.F.);
#26595=ADVANCED_FACE('',(#7771),#1349,.F.);
#26596=ADVANCED_FACE('',(#7772),#1350,.F.);
#26597=ADVANCED_FACE('',(#7773),#1351,.F.);
#26598=ADVANCED_FACE('',(#7774),#1352,.F.);
#26599=ADVANCED_FACE('',(#7775),#1353,.F.);
#26600=ADVANCED_FACE('',(#7776),#1354,.F.);
#26601=ADVANCED_FACE('',(#7777),#1355,.F.);
#26602=ADVANCED_FACE('',(#7778),#1356,.F.);
#26603=ADVANCED_FACE('',(#7779),#1357,.F.);
#26604=ADVANCED_FACE('',(#7780),#1358,.F.);
#26605=ADVANCED_FACE('',(#7781),#1359,.F.);
#26606=ADVANCED_FACE('',(#7782),#1360,.F.);
#26607=ADVANCED_FACE('',(#7783),#1361,.F.);
#26608=ADVANCED_FACE('',(#7784),#1362,.F.);
#26609=ADVANCED_FACE('',(#7785),#1363,.F.);
#26610=ADVANCED_FACE('',(#7786),#1364,.F.);
#26611=ADVANCED_FACE('',(#7787),#1365,.F.);
#26612=ADVANCED_FACE('',(#7788),#1366,.F.);
#26613=ADVANCED_FACE('',(#7789),#1367,.F.);
#26614=ADVANCED_FACE('',(#7790),#1368,.F.);
#26615=ADVANCED_FACE('',(#7791),#6674,.F.);
#27224=CLOSED_SHELL('',(#26173,#26174,#26175,#26176,#26177,#26178,#26179,
#26180,#26181,#26182,#26183,#26184,#26185,#26186,#26187,#26188,#26189,#26190,
#26191,#26192,#26193,#26194,#26195,#26196,#26197,#26198,#26199,#26200,#26201,
#26202,#26203,#26204,#26205,#26206,#26207,#26208,#26209,#26210,#26211,#26212,
#26213,#26214,#26215,#26216,#26217,#26218,#26219,#26220,#26221,#26222,#26223,
#26224,#26225,#26226,#26227,#26228,#26229,#26230,#26231,#26232,#26233,#26234,
#26235,#26236,#26237,#26238,#26239,#26240,#26241,#26242,#26243,#26244,#26245,
#26246,#26247,#26248,#26249,#26250,#26251,#26252,#26253,#26254,#26255,#26256,
#26257,#26258,#26259,#26260,#26261,#26262,#26263,#26264,#26265,#26266,#26267,
#26268,#26269,#26270,#26271,#26272,#26273,#26274,#26275,#26276,#26277,#26278,
#26279,#26280,#26281,#26282,#26283,#26284,#26285,#26286,#26287,#26288,#26289,
#26290,#26291,#26292,#26293,#26294,#26295,#26296,#26297,#26298,#26299,#26300,
#26301,#26302,#26303,#26304,#26305,#26306,#26307,#26308,#26309,#26310,#26311,
#26312,#26313,#26314,#26315,#26316,#26317,#26318,#26319,#26320,#26321,#26322,
#26323,#26324,#26325,#26326,#26327,#26328,#26329,#26330,#26331,#26332,#26333,
#26334,#26335,#26336,#26337,#26338,#26339,#26340,#26341,#26342,#26343,#26344,
#26345,#26346,#26347,#26348,#26349,#26350,#26351,#26352,#26353,#26354,#26355,
#26356,#26357,#26358,#26359,#26360,#26361,#26362,#26363,#26364,#26365,#26366,
#26367,#26368,#26369,#26370,#26371,#26372,#26373,#26374,#26375,#26376,#26377,
#26378,#26379,#26380,#26381,#26382,#26383,#26384,#26385,#26386,#26387,#26388,
#26389,#26390,#26391,#26392,#26393,#26394,#26395,#26396,#26397,#26398,#26399,
#26400,#26401,#26402,#26403,#26404,#26405,#26406,#26407,#26408,#26409,#26410,
#26411,#26412,#26413,#26414,#26415,#26416,#26417,#26418,#26419,#26420,#26421,
#26422,#26423,#26424,#26425,#26426,#26427,#26428,#26429,#26430,#26431,#26432,
#26433,#26434,#26435,#26436,#26437,#26438,#26439,#26440,#26441,#26442,#26443,
#26444,#26445,#26446,#26447,#26448,#26449,#26450,#26451,#26452,#26453,#26454,
#26455,#26456,#26457,#26458,#26459,#26460,#26461,#26462,#26463,#26464,#26465,
#26466,#26467,#26468,#26469,#26470,#26471,#26472,#26473,#26474,#26475,#26476,
#26477,#26478,#26479,#26480,#26481,#26482,#26483,#26484,#26485,#26486,#26487,
#26488,#26489,#26490,#26491,#26492,#26493,#26494,#26495,#26496,#26497,#26498,
#26499,#26500,#26501,#26502,#26503,#26504,#26505,#26506,#26507,#26508,#26509,
#26510,#26511,#26512,#26513,#26514,#26515,#26516,#26517,#26518,#26519,#26520,
#26521,#26522,#26523,#26524,#26525,#26526,#26527,#26528,#26529,#26530,#26531,
#26532,#26533,#26534,#26535,#26536,#26537,#26538,#26539,#26540,#26541,#26542,
#26543,#26544,#26545,#26546,#26547,#26548,#26549,#26550,#26551,#26552,#26553,
#26554,#26555,#26556,#26557,#26558,#26559,#26560,#26561,#26562,#26563,#26564,
#26565,#26566,#26567,#26568,#26569,#26570,#26571,#26572,#26573,#26574,#26575,
#26576,#26577,#26578,#26579,#26580,#26581,#26582,#26583,#26584,#26585,#26586,
#26587,#26588,#26589,#26590,#26591,#26592,#26593,#26594,#26595,#26596,#26597,
#26598,#26599,#26600,#26601,#26602,#26603,#26604,#26605,#26606,#26607,#26608,
#26609,#26610,#26611,#26612,#26613,#26614,#26615));
#28371=AXIS2_PLACEMENT_3D('',#42565,#32389,#32390);
#28372=AXIS2_PLACEMENT_3D('',#42566,#32391,#32392);
#28373=AXIS2_PLACEMENT_3D('',#42569,#32393,#32394);
#28374=AXIS2_PLACEMENT_3D('',#42575,#32398,#32399);
#28375=AXIS2_PLACEMENT_3D('',#42581,#32403,#32404);
#28376=AXIS2_PLACEMENT_3D('',#42583,#32405,#32406);
#28377=AXIS2_PLACEMENT_3D('',#42585,#32407,#32408);
#28378=AXIS2_PLACEMENT_3D('',#42589,#32410,#32411);
#28379=AXIS2_PLACEMENT_3D('',#42593,#32413,#32414);
#28380=AXIS2_PLACEMENT_3D('',#42595,#32415,#32416);
#28381=AXIS2_PLACEMENT_3D('',#42597,#32417,#32418);
#28382=AXIS2_PLACEMENT_3D('',#42601,#32420,#32421);
#28383=AXIS2_PLACEMENT_3D('',#42605,#32423,#32424);
#28384=AXIS2_PLACEMENT_3D('',#42607,#32425,#32426);
#28385=AXIS2_PLACEMENT_3D('',#42611,#32428,#32429);
#28386=AXIS2_PLACEMENT_3D('',#42613,#32430,#32431);
#28387=AXIS2_PLACEMENT_3D('',#42617,#32433,#32434);
#28388=AXIS2_PLACEMENT_3D('',#42621,#32436,#32437);
#28389=AXIS2_PLACEMENT_3D('',#42623,#32438,#32439);
#28390=AXIS2_PLACEMENT_3D('',#42625,#32440,#32441);
#28391=AXIS2_PLACEMENT_3D('',#42629,#32443,#32444);
#28392=AXIS2_PLACEMENT_3D('',#42633,#32446,#32447);
#28393=AXIS2_PLACEMENT_3D('',#42635,#32448,#32449);
#28394=AXIS2_PLACEMENT_3D('',#42637,#32450,#32451);
#28395=AXIS2_PLACEMENT_3D('',#42641,#32453,#32454);
#28396=AXIS2_PLACEMENT_3D('',#42645,#32456,#32457);
#28397=AXIS2_PLACEMENT_3D('',#42647,#32458,#32459);
#28398=AXIS2_PLACEMENT_3D('',#42649,#32460,#32461);
#28399=AXIS2_PLACEMENT_3D('',#42653,#32463,#32464);
#28400=AXIS2_PLACEMENT_3D('',#42657,#32466,#32467);
#28401=AXIS2_PLACEMENT_3D('',#42659,#32468,#32469);
#28402=AXIS2_PLACEMENT_3D('',#42661,#32470,#32471);
#28403=AXIS2_PLACEMENT_3D('',#42665,#32473,#32474);
#28404=AXIS2_PLACEMENT_3D('',#42669,#32476,#32477);
#28405=AXIS2_PLACEMENT_3D('',#42671,#32478,#32479);
#28406=AXIS2_PLACEMENT_3D('',#42673,#32480,#32481);
#28407=AXIS2_PLACEMENT_3D('',#42677,#32483,#32484);
#28408=AXIS2_PLACEMENT_3D('',#42681,#32486,#32487);
#28409=AXIS2_PLACEMENT_3D('',#42683,#32488,#32489);
#28410=AXIS2_PLACEMENT_3D('',#42685,#32490,#32491);
#28411=AXIS2_PLACEMENT_3D('',#42689,#32493,#32494);
#28412=AXIS2_PLACEMENT_3D('',#42693,#32496,#32497);
#28413=AXIS2_PLACEMENT_3D('',#42695,#32498,#32499);
#28414=AXIS2_PLACEMENT_3D('',#42697,#32500,#32501);
#28415=AXIS2_PLACEMENT_3D('',#42701,#32503,#32504);
#28416=AXIS2_PLACEMENT_3D('',#42705,#32506,#32507);
#28417=AXIS2_PLACEMENT_3D('',#42707,#32508,#32509);
#28418=AXIS2_PLACEMENT_3D('',#42709,#32510,#32511);
#28419=AXIS2_PLACEMENT_3D('',#42713,#32513,#32514);
#28420=AXIS2_PLACEMENT_3D('',#42717,#32516,#32517);
#28421=AXIS2_PLACEMENT_3D('',#42719,#32518,#32519);
#28422=AXIS2_PLACEMENT_3D('',#42721,#32520,#32521);
#28423=AXIS2_PLACEMENT_3D('',#42725,#32523,#32524);
#28424=AXIS2_PLACEMENT_3D('',#42729,#32526,#32527);
#28425=AXIS2_PLACEMENT_3D('',#42731,#32528,#32529);
#28426=AXIS2_PLACEMENT_3D('',#42733,#32530,#32531);
#28427=AXIS2_PLACEMENT_3D('',#42737,#32533,#32534);
#28428=AXIS2_PLACEMENT_3D('',#42741,#32536,#32537);
#28429=AXIS2_PLACEMENT_3D('',#42743,#32538,#32539);
#28430=AXIS2_PLACEMENT_3D('',#42745,#32540,#32541);
#28431=AXIS2_PLACEMENT_3D('',#42749,#32543,#32544);
#28432=AXIS2_PLACEMENT_3D('',#42753,#32546,#32547);
#28433=AXIS2_PLACEMENT_3D('',#42755,#32548,#32549);
#28434=AXIS2_PLACEMENT_3D('',#42757,#32550,#32551);
#28435=AXIS2_PLACEMENT_3D('',#42761,#32553,#32554);
#28436=AXIS2_PLACEMENT_3D('',#42765,#32556,#32557);
#28437=AXIS2_PLACEMENT_3D('',#42767,#32558,#32559);
#28438=AXIS2_PLACEMENT_3D('',#42769,#32560,#32561);
#28439=AXIS2_PLACEMENT_3D('',#42773,#32563,#32564);
#28440=AXIS2_PLACEMENT_3D('',#42777,#32566,#32567);
#28441=AXIS2_PLACEMENT_3D('',#42779,#32568,#32569);
#28442=AXIS2_PLACEMENT_3D('',#42781,#32570,#32571);
#28443=AXIS2_PLACEMENT_3D('',#42785,#32573,#32574);
#28444=AXIS2_PLACEMENT_3D('',#42789,#32576,#32577);
#28445=AXIS2_PLACEMENT_3D('',#42791,#32578,#32579);
#28446=AXIS2_PLACEMENT_3D('',#42793,#32580,#32581);
#28447=AXIS2_PLACEMENT_3D('',#42797,#32583,#32584);
#28448=AXIS2_PLACEMENT_3D('',#42801,#32586,#32587);
#28449=AXIS2_PLACEMENT_3D('',#42803,#32588,#32589);
#28450=AXIS2_PLACEMENT_3D('',#42805,#32590,#32591);
#28451=AXIS2_PLACEMENT_3D('',#42809,#32593,#32594);
#28452=AXIS2_PLACEMENT_3D('',#42813,#32596,#32597);
#28453=AXIS2_PLACEMENT_3D('',#42815,#32598,#32599);
#28454=AXIS2_PLACEMENT_3D('',#42817,#32600,#32601);
#28455=AXIS2_PLACEMENT_3D('',#42821,#32603,#32604);
#28456=AXIS2_PLACEMENT_3D('',#42825,#32606,#32607);
#28457=AXIS2_PLACEMENT_3D('',#42827,#32608,#32609);
#28458=AXIS2_PLACEMENT_3D('',#42829,#32610,#32611);
#28459=AXIS2_PLACEMENT_3D('',#42833,#32613,#32614);
#28460=AXIS2_PLACEMENT_3D('',#42837,#32616,#32617);
#28461=AXIS2_PLACEMENT_3D('',#42839,#32618,#32619);
#28462=AXIS2_PLACEMENT_3D('',#42841,#32620,#32621);
#28463=AXIS2_PLACEMENT_3D('',#42845,#32623,#32624);
#28464=AXIS2_PLACEMENT_3D('',#42849,#32626,#32627);
#28465=AXIS2_PLACEMENT_3D('',#42851,#32628,#32629);
#28466=AXIS2_PLACEMENT_3D('',#42853,#32630,#32631);
#28467=AXIS2_PLACEMENT_3D('',#42857,#32633,#32634);
#28468=AXIS2_PLACEMENT_3D('',#42861,#32636,#32637);
#28469=AXIS2_PLACEMENT_3D('',#42863,#32638,#32639);
#28470=AXIS2_PLACEMENT_3D('',#42865,#32640,#32641);
#28471=AXIS2_PLACEMENT_3D('',#42869,#32643,#32644);
#28472=AXIS2_PLACEMENT_3D('',#42873,#32646,#32647);
#28473=AXIS2_PLACEMENT_3D('',#42875,#32648,#32649);
#28474=AXIS2_PLACEMENT_3D('',#42877,#32650,#32651);
#28475=AXIS2_PLACEMENT_3D('',#42881,#32653,#32654);
#28476=AXIS2_PLACEMENT_3D('',#42885,#32656,#32657);
#28477=AXIS2_PLACEMENT_3D('',#42887,#32658,#32659);
#28478=AXIS2_PLACEMENT_3D('',#42889,#32660,#32661);
#28479=AXIS2_PLACEMENT_3D('',#42893,#32663,#32664);
#28480=AXIS2_PLACEMENT_3D('',#42897,#32666,#32667);
#28481=AXIS2_PLACEMENT_3D('',#42899,#32668,#32669);
#28482=AXIS2_PLACEMENT_3D('',#42901,#32670,#32671);
#28483=AXIS2_PLACEMENT_3D('',#42905,#32673,#32674);
#28484=AXIS2_PLACEMENT_3D('',#42909,#32676,#32677);
#28485=AXIS2_PLACEMENT_3D('',#42911,#32678,#32679);
#28486=AXIS2_PLACEMENT_3D('',#42913,#32680,#32681);
#28487=AXIS2_PLACEMENT_3D('',#42917,#32683,#32684);
#28488=AXIS2_PLACEMENT_3D('',#42921,#32686,#32687);
#28489=AXIS2_PLACEMENT_3D('',#42923,#32688,#32689);
#28490=AXIS2_PLACEMENT_3D('',#42925,#32690,#32691);
#28491=AXIS2_PLACEMENT_3D('',#42929,#32693,#32694);
#28492=AXIS2_PLACEMENT_3D('',#42933,#32696,#32697);
#28493=AXIS2_PLACEMENT_3D('',#42935,#32698,#32699);
#28494=AXIS2_PLACEMENT_3D('',#42937,#32700,#32701);
#28495=AXIS2_PLACEMENT_3D('',#42941,#32703,#32704);
#28496=AXIS2_PLACEMENT_3D('',#42945,#32706,#32707);
#28497=AXIS2_PLACEMENT_3D('',#42947,#32708,#32709);
#28498=AXIS2_PLACEMENT_3D('',#42949,#32710,#32711);
#28499=AXIS2_PLACEMENT_3D('',#42953,#32713,#32714);
#28500=AXIS2_PLACEMENT_3D('',#42957,#32716,#32717);
#28501=AXIS2_PLACEMENT_3D('',#42959,#32718,#32719);
#28502=AXIS2_PLACEMENT_3D('',#42961,#32720,#32721);
#28503=AXIS2_PLACEMENT_3D('',#42965,#32723,#32724);
#28504=AXIS2_PLACEMENT_3D('',#42969,#32726,#32727);
#28505=AXIS2_PLACEMENT_3D('',#42970,#32728,#32729);
#28506=AXIS2_PLACEMENT_3D('',#42972,#32730,#32731);
#28507=AXIS2_PLACEMENT_3D('',#42974,#32732,#32733);
#28508=AXIS2_PLACEMENT_3D('',#42978,#32735,#32736);
#28509=AXIS2_PLACEMENT_3D('',#42982,#32738,#32739);
#28510=AXIS2_PLACEMENT_3D('',#42984,#32740,#32741);
#28511=AXIS2_PLACEMENT_3D('',#42986,#32742,#32743);
#28512=AXIS2_PLACEMENT_3D('',#42990,#32745,#32746);
#28513=AXIS2_PLACEMENT_3D('',#42994,#32748,#32749);
#28514=AXIS2_PLACEMENT_3D('',#42996,#32750,#32751);
#28515=AXIS2_PLACEMENT_3D('',#42998,#32752,#32753);
#28516=AXIS2_PLACEMENT_3D('',#43002,#32755,#32756);
#28517=AXIS2_PLACEMENT_3D('',#43006,#32758,#32759);
#28518=AXIS2_PLACEMENT_3D('',#43008,#32760,#32761);
#28519=AXIS2_PLACEMENT_3D('',#43010,#32762,#32763);
#28520=AXIS2_PLACEMENT_3D('',#43014,#32765,#32766);
#28521=AXIS2_PLACEMENT_3D('',#43018,#32768,#32769);
#28522=AXIS2_PLACEMENT_3D('',#43020,#32770,#32771);
#28523=AXIS2_PLACEMENT_3D('',#43022,#32772,#32773);
#28524=AXIS2_PLACEMENT_3D('',#43026,#32775,#32776);
#28525=AXIS2_PLACEMENT_3D('',#43030,#32778,#32779);
#28526=AXIS2_PLACEMENT_3D('',#43032,#32780,#32781);
#28527=AXIS2_PLACEMENT_3D('',#43034,#32782,#32783);
#28528=AXIS2_PLACEMENT_3D('',#43038,#32785,#32786);
#28529=AXIS2_PLACEMENT_3D('',#43042,#32788,#32789);
#28530=AXIS2_PLACEMENT_3D('',#43044,#32790,#32791);
#28531=AXIS2_PLACEMENT_3D('',#43046,#32792,#32793);
#28532=AXIS2_PLACEMENT_3D('',#43050,#32795,#32796);
#28533=AXIS2_PLACEMENT_3D('',#43054,#32798,#32799);
#28534=AXIS2_PLACEMENT_3D('',#43056,#32800,#32801);
#28535=AXIS2_PLACEMENT_3D('',#43058,#32802,#32803);
#28536=AXIS2_PLACEMENT_3D('',#43062,#32805,#32806);
#28537=AXIS2_PLACEMENT_3D('',#43066,#32808,#32809);
#28538=AXIS2_PLACEMENT_3D('',#43068,#32810,#32811);
#28539=AXIS2_PLACEMENT_3D('',#43070,#32812,#32813);
#28540=AXIS2_PLACEMENT_3D('',#43074,#32815,#32816);
#28541=AXIS2_PLACEMENT_3D('',#43078,#32818,#32819);
#28542=AXIS2_PLACEMENT_3D('',#43080,#32820,#32821);
#28543=AXIS2_PLACEMENT_3D('',#43082,#32822,#32823);
#28544=AXIS2_PLACEMENT_3D('',#43086,#32825,#32826);
#28545=AXIS2_PLACEMENT_3D('',#43090,#32828,#32829);
#28546=AXIS2_PLACEMENT_3D('',#43092,#32830,#32831);
#28547=AXIS2_PLACEMENT_3D('',#43094,#32832,#32833);
#28548=AXIS2_PLACEMENT_3D('',#43098,#32835,#32836);
#28549=AXIS2_PLACEMENT_3D('',#43102,#32838,#32839);
#28550=AXIS2_PLACEMENT_3D('',#43104,#32840,#32841);
#28551=AXIS2_PLACEMENT_3D('',#43106,#32842,#32843);
#28552=AXIS2_PLACEMENT_3D('',#43110,#32845,#32846);
#28553=AXIS2_PLACEMENT_3D('',#43114,#32848,#32849);
#28554=AXIS2_PLACEMENT_3D('',#43116,#32850,#32851);
#28555=AXIS2_PLACEMENT_3D('',#43118,#32852,#32853);
#28556=AXIS2_PLACEMENT_3D('',#43122,#32855,#32856);
#28557=AXIS2_PLACEMENT_3D('',#43126,#32858,#32859);
#28558=AXIS2_PLACEMENT_3D('',#43128,#32860,#32861);
#28559=AXIS2_PLACEMENT_3D('',#43130,#32862,#32863);
#28560=AXIS2_PLACEMENT_3D('',#43134,#32865,#32866);
#28561=AXIS2_PLACEMENT_3D('',#43138,#32868,#32869);
#28562=AXIS2_PLACEMENT_3D('',#43140,#32870,#32871);
#28563=AXIS2_PLACEMENT_3D('',#43142,#32872,#32873);
#28564=AXIS2_PLACEMENT_3D('',#43146,#32875,#32876);
#28565=AXIS2_PLACEMENT_3D('',#43150,#32878,#32879);
#28566=AXIS2_PLACEMENT_3D('',#43152,#32880,#32881);
#28567=AXIS2_PLACEMENT_3D('',#43154,#32882,#32883);
#28568=AXIS2_PLACEMENT_3D('',#43158,#32885,#32886);
#28569=AXIS2_PLACEMENT_3D('',#43162,#32888,#32889);
#28570=AXIS2_PLACEMENT_3D('',#43164,#32890,#32891);
#28571=AXIS2_PLACEMENT_3D('',#43166,#32892,#32893);
#28572=AXIS2_PLACEMENT_3D('',#43170,#32895,#32896);
#28573=AXIS2_PLACEMENT_3D('',#43174,#32898,#32899);
#28574=AXIS2_PLACEMENT_3D('',#43176,#32900,#32901);
#28575=AXIS2_PLACEMENT_3D('',#43178,#32902,#32903);
#28576=AXIS2_PLACEMENT_3D('',#43182,#32905,#32906);
#28577=AXIS2_PLACEMENT_3D('',#43186,#32908,#32909);
#28578=AXIS2_PLACEMENT_3D('',#43188,#32910,#32911);
#28579=AXIS2_PLACEMENT_3D('',#43190,#32912,#32913);
#28580=AXIS2_PLACEMENT_3D('',#43194,#32915,#32916);
#28581=AXIS2_PLACEMENT_3D('',#43198,#32918,#32919);
#28582=AXIS2_PLACEMENT_3D('',#43200,#32920,#32921);
#28583=AXIS2_PLACEMENT_3D('',#43202,#32922,#32923);
#28584=AXIS2_PLACEMENT_3D('',#43206,#32925,#32926);
#28585=AXIS2_PLACEMENT_3D('',#43210,#32928,#32929);
#28586=AXIS2_PLACEMENT_3D('',#43212,#32930,#32931);
#28587=AXIS2_PLACEMENT_3D('',#43214,#32932,#32933);
#28588=AXIS2_PLACEMENT_3D('',#43218,#32935,#32936);
#28589=AXIS2_PLACEMENT_3D('',#43222,#32938,#32939);
#28590=AXIS2_PLACEMENT_3D('',#43224,#32940,#32941);
#28591=AXIS2_PLACEMENT_3D('',#43226,#32942,#32943);
#28592=AXIS2_PLACEMENT_3D('',#43230,#32945,#32946);
#28593=AXIS2_PLACEMENT_3D('',#43234,#32948,#32949);
#28594=AXIS2_PLACEMENT_3D('',#43236,#32950,#32951);
#28595=AXIS2_PLACEMENT_3D('',#43238,#32952,#32953);
#28596=AXIS2_PLACEMENT_3D('',#43242,#32955,#32956);
#28597=AXIS2_PLACEMENT_3D('',#43246,#32958,#32959);
#28598=AXIS2_PLACEMENT_3D('',#43248,#32960,#32961);
#28599=AXIS2_PLACEMENT_3D('',#43250,#32962,#32963);
#28600=AXIS2_PLACEMENT_3D('',#43254,#32965,#32966);
#28601=AXIS2_PLACEMENT_3D('',#43258,#32968,#32969);
#28602=AXIS2_PLACEMENT_3D('',#43260,#32970,#32971);
#28603=AXIS2_PLACEMENT_3D('',#43262,#32972,#32973);
#28604=AXIS2_PLACEMENT_3D('',#43266,#32975,#32976);
#28605=AXIS2_PLACEMENT_3D('',#43270,#32978,#32979);
#28606=AXIS2_PLACEMENT_3D('',#43272,#32980,#32981);
#28607=AXIS2_PLACEMENT_3D('',#43274,#32982,#32983);
#28608=AXIS2_PLACEMENT_3D('',#43278,#32985,#32986);
#28609=AXIS2_PLACEMENT_3D('',#43282,#32988,#32989);
#28610=AXIS2_PLACEMENT_3D('',#43284,#32990,#32991);
#28611=AXIS2_PLACEMENT_3D('',#43286,#32992,#32993);
#28612=AXIS2_PLACEMENT_3D('',#43290,#32995,#32996);
#28613=AXIS2_PLACEMENT_3D('',#43294,#32998,#32999);
#28614=AXIS2_PLACEMENT_3D('',#43296,#33000,#33001);
#28615=AXIS2_PLACEMENT_3D('',#43298,#33002,#33003);
#28616=AXIS2_PLACEMENT_3D('',#43301,#33005,#33006);
#28617=AXIS2_PLACEMENT_3D('',#43302,#33007,#33008);
#28618=AXIS2_PLACEMENT_3D('',#43308,#33012,#33013);
#28619=AXIS2_PLACEMENT_3D('',#43314,#33017,#33018);
#28620=AXIS2_PLACEMENT_3D('',#43317,#33021,#33022);
#28621=AXIS2_PLACEMENT_3D('',#43321,#33025,#33026);
#28622=AXIS2_PLACEMENT_3D('',#43325,#33029,#33030);
#28623=AXIS2_PLACEMENT_3D('',#43327,#33032,#33033);
#28624=AXIS2_PLACEMENT_3D('',#43333,#33037,#33038);
#28625=AXIS2_PLACEMENT_3D('',#43339,#33042,#33043);
#28626=AXIS2_PLACEMENT_3D('',#43342,#33046,#33047);
#28627=AXIS2_PLACEMENT_3D('',#43346,#33050,#33051);
#28628=AXIS2_PLACEMENT_3D('',#43350,#33054,#33055);
#28629=AXIS2_PLACEMENT_3D('',#43352,#33057,#33058);
#28630=AXIS2_PLACEMENT_3D('',#43358,#33062,#33063);
#28631=AXIS2_PLACEMENT_3D('',#43364,#33067,#33068);
#28632=AXIS2_PLACEMENT_3D('',#43367,#33071,#33072);
#28633=AXIS2_PLACEMENT_3D('',#43371,#33075,#33076);
#28634=AXIS2_PLACEMENT_3D('',#43375,#33079,#33080);
#28635=AXIS2_PLACEMENT_3D('',#43377,#33082,#33083);
#28636=AXIS2_PLACEMENT_3D('',#43383,#33087,#33088);
#28637=AXIS2_PLACEMENT_3D('',#43389,#33092,#33093);
#28638=AXIS2_PLACEMENT_3D('',#43393,#33096,#33097);
#28639=AXIS2_PLACEMENT_3D('',#43397,#33100,#33101);
#28640=AXIS2_PLACEMENT_3D('',#43400,#33104,#33105);
#28641=AXIS2_PLACEMENT_3D('',#43533,#33184,#33185);
#28642=AXIS2_PLACEMENT_3D('',#43541,#33189,#33190);
#28643=AXIS2_PLACEMENT_3D('',#43545,#33193,#33194);
#28644=AXIS2_PLACEMENT_3D('',#43549,#33197,#33198);
#28645=AXIS2_PLACEMENT_3D('',#43553,#33201,#33202);
#28646=AXIS2_PLACEMENT_3D('',#43555,#33204,#33205);
#28647=AXIS2_PLACEMENT_3D('',#43559,#33208,#33209);
#28648=AXIS2_PLACEMENT_3D('',#43563,#33212,#33213);
#28649=AXIS2_PLACEMENT_3D('',#43565,#33215,#33216);
#28650=AXIS2_PLACEMENT_3D('',#43569,#33219,#33220);
#28651=AXIS2_PLACEMENT_3D('',#43573,#33223,#33224);
#28652=AXIS2_PLACEMENT_3D('',#43575,#33226,#33227);
#28653=AXIS2_PLACEMENT_3D('',#43579,#33230,#33231);
#28654=AXIS2_PLACEMENT_3D('',#43583,#33234,#33235);
#28655=AXIS2_PLACEMENT_3D('',#43585,#33237,#33238);
#28656=AXIS2_PLACEMENT_3D('',#43589,#33241,#33242);
#28657=AXIS2_PLACEMENT_3D('',#43593,#33245,#33246);
#28658=AXIS2_PLACEMENT_3D('',#43595,#33248,#33249);
#28659=AXIS2_PLACEMENT_3D('',#43599,#33252,#33253);
#28660=AXIS2_PLACEMENT_3D('',#43603,#33256,#33257);
#28661=AXIS2_PLACEMENT_3D('',#43605,#33259,#33260);
#28662=AXIS2_PLACEMENT_3D('',#43609,#33263,#33264);
#28663=AXIS2_PLACEMENT_3D('',#43613,#33267,#33268);
#28664=AXIS2_PLACEMENT_3D('',#43615,#33270,#33271);
#28665=AXIS2_PLACEMENT_3D('',#43619,#33274,#33275);
#28666=AXIS2_PLACEMENT_3D('',#43623,#33278,#33279);
#28667=AXIS2_PLACEMENT_3D('',#43625,#33281,#33282);
#28668=AXIS2_PLACEMENT_3D('',#43629,#33285,#33286);
#28669=AXIS2_PLACEMENT_3D('',#43633,#33289,#33290);
#28670=AXIS2_PLACEMENT_3D('',#43635,#33292,#33293);
#28671=AXIS2_PLACEMENT_3D('',#43639,#33296,#33297);
#28672=AXIS2_PLACEMENT_3D('',#43643,#33300,#33301);
#28673=AXIS2_PLACEMENT_3D('',#43645,#33303,#33304);
#28674=AXIS2_PLACEMENT_3D('',#43649,#33307,#33308);
#28675=AXIS2_PLACEMENT_3D('',#43653,#33311,#33312);
#28676=AXIS2_PLACEMENT_3D('',#43655,#33314,#33315);
#28677=AXIS2_PLACEMENT_3D('',#43659,#33318,#33319);
#28678=AXIS2_PLACEMENT_3D('',#43663,#33322,#33323);
#28679=AXIS2_PLACEMENT_3D('',#43665,#33325,#33326);
#28680=AXIS2_PLACEMENT_3D('',#43669,#33329,#33330);
#28681=AXIS2_PLACEMENT_3D('',#43673,#33333,#33334);
#28682=AXIS2_PLACEMENT_3D('',#43675,#33336,#33337);
#28683=AXIS2_PLACEMENT_3D('',#43679,#33340,#33341);
#28684=AXIS2_PLACEMENT_3D('',#43683,#33344,#33345);
#28685=AXIS2_PLACEMENT_3D('',#43685,#33347,#33348);
#28686=AXIS2_PLACEMENT_3D('',#43689,#33351,#33352);
#28687=AXIS2_PLACEMENT_3D('',#43693,#33355,#33356);
#28688=AXIS2_PLACEMENT_3D('',#43695,#33358,#33359);
#28689=AXIS2_PLACEMENT_3D('',#43699,#33362,#33363);
#28690=AXIS2_PLACEMENT_3D('',#43703,#33366,#33367);
#28691=AXIS2_PLACEMENT_3D('',#43705,#33369,#33370);
#28692=AXIS2_PLACEMENT_3D('',#43709,#33373,#33374);
#28693=AXIS2_PLACEMENT_3D('',#43713,#33377,#33378);
#28694=AXIS2_PLACEMENT_3D('',#43715,#33380,#33381);
#28695=AXIS2_PLACEMENT_3D('',#43719,#33384,#33385);
#28696=AXIS2_PLACEMENT_3D('',#43723,#33388,#33389);
#28697=AXIS2_PLACEMENT_3D('',#43725,#33391,#33392);
#28698=AXIS2_PLACEMENT_3D('',#43729,#33395,#33396);
#28699=AXIS2_PLACEMENT_3D('',#43733,#33399,#33400);
#28700=AXIS2_PLACEMENT_3D('',#43735,#33402,#33403);
#28701=AXIS2_PLACEMENT_3D('',#43739,#33406,#33407);
#28702=AXIS2_PLACEMENT_3D('',#43743,#33410,#33411);
#28703=AXIS2_PLACEMENT_3D('',#43747,#33414,#33415);
#28704=AXIS2_PLACEMENT_3D('',#43749,#33417,#33418);
#28705=AXIS2_PLACEMENT_3D('',#43753,#33421,#33422);
#28706=AXIS2_PLACEMENT_3D('',#43755,#33424,#33425);
#28707=AXIS2_PLACEMENT_3D('',#43759,#33428,#33429);
#28708=AXIS2_PLACEMENT_3D('',#43763,#33432,#33433);
#28709=AXIS2_PLACEMENT_3D('',#43765,#33435,#33436);
#28710=AXIS2_PLACEMENT_3D('',#43769,#33439,#33440);
#28711=AXIS2_PLACEMENT_3D('',#43773,#33443,#33444);
#28712=AXIS2_PLACEMENT_3D('',#43775,#33446,#33447);
#28713=AXIS2_PLACEMENT_3D('',#43779,#33450,#33451);
#28714=AXIS2_PLACEMENT_3D('',#43783,#33454,#33455);
#28715=AXIS2_PLACEMENT_3D('',#43785,#33457,#33458);
#28716=AXIS2_PLACEMENT_3D('',#43789,#33461,#33462);
#28717=AXIS2_PLACEMENT_3D('',#43793,#33465,#33466);
#28718=AXIS2_PLACEMENT_3D('',#43795,#33468,#33469);
#28719=AXIS2_PLACEMENT_3D('',#43799,#33472,#33473);
#28720=AXIS2_PLACEMENT_3D('',#43803,#33476,#33477);
#28721=AXIS2_PLACEMENT_3D('',#43805,#33479,#33480);
#28722=AXIS2_PLACEMENT_3D('',#43809,#33483,#33484);
#28723=AXIS2_PLACEMENT_3D('',#43813,#33487,#33488);
#28724=AXIS2_PLACEMENT_3D('',#43815,#33490,#33491);
#28725=AXIS2_PLACEMENT_3D('',#43819,#33494,#33495);
#28726=AXIS2_PLACEMENT_3D('',#43823,#33498,#33499);
#28727=AXIS2_PLACEMENT_3D('',#43825,#33501,#33502);
#28728=AXIS2_PLACEMENT_3D('',#43829,#33505,#33506);
#28729=AXIS2_PLACEMENT_3D('',#43833,#33509,#33510);
#28730=AXIS2_PLACEMENT_3D('',#43835,#33512,#33513);
#28731=AXIS2_PLACEMENT_3D('',#43839,#33516,#33517);
#28732=AXIS2_PLACEMENT_3D('',#43843,#33520,#33521);
#28733=AXIS2_PLACEMENT_3D('',#43845,#33523,#33524);
#28734=AXIS2_PLACEMENT_3D('',#43849,#33527,#33528);
#28735=AXIS2_PLACEMENT_3D('',#43853,#33531,#33532);
#28736=AXIS2_PLACEMENT_3D('',#43855,#33534,#33535);
#28737=AXIS2_PLACEMENT_3D('',#43859,#33538,#33539);
#28738=AXIS2_PLACEMENT_3D('',#43863,#33542,#33543);
#28739=AXIS2_PLACEMENT_3D('',#43865,#33545,#33546);
#28740=AXIS2_PLACEMENT_3D('',#43869,#33549,#33550);
#28741=AXIS2_PLACEMENT_3D('',#43873,#33553,#33554);
#28742=AXIS2_PLACEMENT_3D('',#43875,#33556,#33557);
#28743=AXIS2_PLACEMENT_3D('',#43879,#33560,#33561);
#28744=AXIS2_PLACEMENT_3D('',#43883,#33564,#33565);
#28745=AXIS2_PLACEMENT_3D('',#43885,#33567,#33568);
#28746=AXIS2_PLACEMENT_3D('',#43889,#33571,#33572);
#28747=AXIS2_PLACEMENT_3D('',#43893,#33575,#33576);
#28748=AXIS2_PLACEMENT_3D('',#43895,#33578,#33579);
#28749=AXIS2_PLACEMENT_3D('',#43899,#33582,#33583);
#28750=AXIS2_PLACEMENT_3D('',#43903,#33586,#33587);
#28751=AXIS2_PLACEMENT_3D('',#43905,#33589,#33590);
#28752=AXIS2_PLACEMENT_3D('',#43909,#33593,#33594);
#28753=AXIS2_PLACEMENT_3D('',#43913,#33597,#33598);
#28754=AXIS2_PLACEMENT_3D('',#43915,#33600,#33601);
#28755=AXIS2_PLACEMENT_3D('',#43919,#33604,#33605);
#28756=AXIS2_PLACEMENT_3D('',#43923,#33608,#33609);
#28757=AXIS2_PLACEMENT_3D('',#43925,#33611,#33612);
#28758=AXIS2_PLACEMENT_3D('',#43929,#33615,#33616);
#28759=AXIS2_PLACEMENT_3D('',#43933,#33619,#33620);
#28760=AXIS2_PLACEMENT_3D('',#43935,#33622,#33623);
#28761=AXIS2_PLACEMENT_3D('',#43939,#33626,#33627);
#28762=AXIS2_PLACEMENT_3D('',#43943,#33630,#33631);
#28763=AXIS2_PLACEMENT_3D('',#43945,#33633,#33634);
#28764=AXIS2_PLACEMENT_3D('',#43949,#33637,#33638);
#28765=AXIS2_PLACEMENT_3D('',#43953,#33641,#33642);
#28766=AXIS2_PLACEMENT_3D('',#43955,#33644,#33645);
#28767=AXIS2_PLACEMENT_3D('',#43959,#33648,#33649);
#28768=AXIS2_PLACEMENT_3D('',#43963,#33652,#33653);
#28769=AXIS2_PLACEMENT_3D('',#43965,#33655,#33656);
#28770=AXIS2_PLACEMENT_3D('',#43969,#33659,#33660);
#28771=AXIS2_PLACEMENT_3D('',#43973,#33663,#33664);
#28772=AXIS2_PLACEMENT_3D('',#43975,#33666,#33667);
#28773=AXIS2_PLACEMENT_3D('',#43979,#33670,#33671);
#28774=AXIS2_PLACEMENT_3D('',#43983,#33674,#33675);
#28775=AXIS2_PLACEMENT_3D('',#43985,#33677,#33678);
#28776=AXIS2_PLACEMENT_3D('',#43989,#33681,#33682);
#28777=AXIS2_PLACEMENT_3D('',#43993,#33685,#33686);
#28778=AXIS2_PLACEMENT_3D('',#43995,#33688,#33689);
#28779=AXIS2_PLACEMENT_3D('',#44004,#33694,#33695);
#28780=AXIS2_PLACEMENT_3D('',#44007,#33698,#33699);
#28781=AXIS2_PLACEMENT_3D('',#44162,#33791,#33792);
#28782=AXIS2_PLACEMENT_3D('',#44169,#33796,#33797);
#28783=AXIS2_PLACEMENT_3D('',#44170,#33798,#33799);
#28784=AXIS2_PLACEMENT_3D('',#44172,#33801,#33802);
#28785=AXIS2_PLACEMENT_3D('',#44178,#33806,#33807);
#28786=AXIS2_PLACEMENT_3D('',#44180,#33809,#33810);
#28787=AXIS2_PLACEMENT_3D('',#44182,#33812,#33813);
#28788=AXIS2_PLACEMENT_3D('',#44188,#33817,#33818);
#28789=AXIS2_PLACEMENT_3D('',#44190,#33820,#33821);
#28790=AXIS2_PLACEMENT_3D('',#44192,#33823,#33824);
#28791=AXIS2_PLACEMENT_3D('',#44196,#33827,#33828);
#28792=AXIS2_PLACEMENT_3D('',#44200,#33831,#33832);
#28793=AXIS2_PLACEMENT_3D('',#44206,#33836,#33837);
#28794=AXIS2_PLACEMENT_3D('',#44208,#33839,#33840);
#28795=AXIS2_PLACEMENT_3D('',#44210,#33842,#33843);
#28796=AXIS2_PLACEMENT_3D('',#44216,#33847,#33848);
#28797=AXIS2_PLACEMENT_3D('',#44218,#33850,#33851);
#28798=AXIS2_PLACEMENT_3D('',#44220,#33853,#33854);
#28799=AXIS2_PLACEMENT_3D('',#44224,#33857,#33858);
#28800=AXIS2_PLACEMENT_3D('',#44228,#33861,#33862);
#28801=AXIS2_PLACEMENT_3D('',#44234,#33866,#33867);
#28802=AXIS2_PLACEMENT_3D('',#44236,#33869,#33870);
#28803=AXIS2_PLACEMENT_3D('',#44238,#33872,#33873);
#28804=AXIS2_PLACEMENT_3D('',#44244,#33877,#33878);
#28805=AXIS2_PLACEMENT_3D('',#44246,#33880,#33881);
#28806=AXIS2_PLACEMENT_3D('',#44248,#33883,#33884);
#28807=AXIS2_PLACEMENT_3D('',#44252,#33887,#33888);
#28808=AXIS2_PLACEMENT_3D('',#44256,#33891,#33892);
#28809=AXIS2_PLACEMENT_3D('',#44260,#33895,#33896);
#28810=AXIS2_PLACEMENT_3D('',#44264,#33899,#33900);
#28811=AXIS2_PLACEMENT_3D('',#44266,#33902,#33903);
#28812=AXIS2_PLACEMENT_3D('',#44272,#33907,#33908);
#28813=AXIS2_PLACEMENT_3D('',#44274,#33910,#33911);
#28814=AXIS2_PLACEMENT_3D('',#44276,#33913,#33914);
#28815=AXIS2_PLACEMENT_3D('',#44282,#33918,#33919);
#28816=AXIS2_PLACEMENT_3D('',#44284,#33921,#33922);
#28817=AXIS2_PLACEMENT_3D('',#44286,#33924,#33925);
#28818=AXIS2_PLACEMENT_3D('',#44290,#33928,#33929);
#28819=AXIS2_PLACEMENT_3D('',#44294,#33932,#33933);
#28820=AXIS2_PLACEMENT_3D('',#44300,#33937,#33938);
#28821=AXIS2_PLACEMENT_3D('',#44302,#33940,#33941);
#28822=AXIS2_PLACEMENT_3D('',#44304,#33943,#33944);
#28823=AXIS2_PLACEMENT_3D('',#44310,#33948,#33949);
#28824=AXIS2_PLACEMENT_3D('',#44312,#33951,#33952);
#28825=AXIS2_PLACEMENT_3D('',#44314,#33954,#33955);
#28826=AXIS2_PLACEMENT_3D('',#44318,#33958,#33959);
#28827=AXIS2_PLACEMENT_3D('',#44322,#33962,#33963);
#28828=AXIS2_PLACEMENT_3D('',#44328,#33967,#33968);
#28829=AXIS2_PLACEMENT_3D('',#44330,#33970,#33971);
#28830=AXIS2_PLACEMENT_3D('',#44332,#33973,#33974);
#28831=AXIS2_PLACEMENT_3D('',#44338,#33978,#33979);
#28832=AXIS2_PLACEMENT_3D('',#44340,#33981,#33982);
#28833=AXIS2_PLACEMENT_3D('',#44342,#33984,#33985);
#28834=AXIS2_PLACEMENT_3D('',#44346,#33988,#33989);
#28835=AXIS2_PLACEMENT_3D('',#44350,#33992,#33993);
#28836=AXIS2_PLACEMENT_3D('',#44356,#33997,#33998);
#28837=AXIS2_PLACEMENT_3D('',#44358,#34000,#34001);
#28838=AXIS2_PLACEMENT_3D('',#44360,#34003,#34004);
#28839=AXIS2_PLACEMENT_3D('',#44366,#34008,#34009);
#28840=AXIS2_PLACEMENT_3D('',#44368,#34011,#34012);
#28841=AXIS2_PLACEMENT_3D('',#44370,#34014,#34015);
#28842=AXIS2_PLACEMENT_3D('',#44374,#34018,#34019);
#28843=AXIS2_PLACEMENT_3D('',#44378,#34022,#34023);
#28844=AXIS2_PLACEMENT_3D('',#44384,#34027,#34028);
#28845=AXIS2_PLACEMENT_3D('',#44386,#34030,#34031);
#28846=AXIS2_PLACEMENT_3D('',#44388,#34033,#34034);
#28847=AXIS2_PLACEMENT_3D('',#44394,#34038,#34039);
#28848=AXIS2_PLACEMENT_3D('',#44396,#34041,#34042);
#28849=AXIS2_PLACEMENT_3D('',#44398,#34044,#34045);
#28850=AXIS2_PLACEMENT_3D('',#44402,#34048,#34049);
#28851=AXIS2_PLACEMENT_3D('',#44406,#34052,#34053);
#28852=AXIS2_PLACEMENT_3D('',#44412,#34057,#34058);
#28853=AXIS2_PLACEMENT_3D('',#44414,#34060,#34061);
#28854=AXIS2_PLACEMENT_3D('',#44416,#34063,#34064);
#28855=AXIS2_PLACEMENT_3D('',#44422,#34068,#34069);
#28856=AXIS2_PLACEMENT_3D('',#44424,#34071,#34072);
#28857=AXIS2_PLACEMENT_3D('',#44426,#34074,#34075);
#28858=AXIS2_PLACEMENT_3D('',#44430,#34078,#34079);
#28859=AXIS2_PLACEMENT_3D('',#44434,#34082,#34083);
#28860=AXIS2_PLACEMENT_3D('',#44440,#34087,#34088);
#28861=AXIS2_PLACEMENT_3D('',#44442,#34090,#34091);
#28862=AXIS2_PLACEMENT_3D('',#44444,#34093,#34094);
#28863=AXIS2_PLACEMENT_3D('',#44450,#34098,#34099);
#28864=AXIS2_PLACEMENT_3D('',#44452,#34101,#34102);
#28865=AXIS2_PLACEMENT_3D('',#44454,#34104,#34105);
#28866=AXIS2_PLACEMENT_3D('',#44460,#34109,#34110);
#28867=AXIS2_PLACEMENT_3D('',#44462,#34112,#34113);
#28868=AXIS2_PLACEMENT_3D('',#44464,#34115,#34116);
#28869=AXIS2_PLACEMENT_3D('',#44468,#34119,#34120);
#28870=AXIS2_PLACEMENT_3D('',#44472,#34123,#34124);
#28871=AXIS2_PLACEMENT_3D('',#44478,#34128,#34129);
#28872=AXIS2_PLACEMENT_3D('',#44480,#34131,#34132);
#28873=AXIS2_PLACEMENT_3D('',#44482,#34134,#34135);
#28874=AXIS2_PLACEMENT_3D('',#44488,#34139,#34140);
#28875=AXIS2_PLACEMENT_3D('',#44490,#34142,#34143);
#28876=AXIS2_PLACEMENT_3D('',#44492,#34145,#34146);
#28877=AXIS2_PLACEMENT_3D('',#44496,#34149,#34150);
#28878=AXIS2_PLACEMENT_3D('',#44500,#34153,#34154);
#28879=AXIS2_PLACEMENT_3D('',#44506,#34158,#34159);
#28880=AXIS2_PLACEMENT_3D('',#44508,#34161,#34162);
#28881=AXIS2_PLACEMENT_3D('',#44510,#34164,#34165);
#28882=AXIS2_PLACEMENT_3D('',#44516,#34169,#34170);
#28883=AXIS2_PLACEMENT_3D('',#44518,#34172,#34173);
#28884=AXIS2_PLACEMENT_3D('',#44520,#34175,#34176);
#28885=AXIS2_PLACEMENT_3D('',#44524,#34179,#34180);
#28886=AXIS2_PLACEMENT_3D('',#44528,#34183,#34184);
#28887=AXIS2_PLACEMENT_3D('',#44532,#34187,#34188);
#28888=AXIS2_PLACEMENT_3D('',#44536,#34191,#34192);
#28889=AXIS2_PLACEMENT_3D('',#44538,#34194,#34195);
#28890=AXIS2_PLACEMENT_3D('',#44544,#34199,#34200);
#28891=AXIS2_PLACEMENT_3D('',#44546,#34202,#34203);
#28892=AXIS2_PLACEMENT_3D('',#44548,#34205,#34206);
#28893=AXIS2_PLACEMENT_3D('',#44554,#34210,#34211);
#28894=AXIS2_PLACEMENT_3D('',#44556,#34213,#34214);
#28895=AXIS2_PLACEMENT_3D('',#44558,#34216,#34217);
#28896=AXIS2_PLACEMENT_3D('',#44562,#34220,#34221);
#28897=AXIS2_PLACEMENT_3D('',#44566,#34224,#34225);
#28898=AXIS2_PLACEMENT_3D('',#44572,#34229,#34230);
#28899=AXIS2_PLACEMENT_3D('',#44574,#34231,#34232);
#28900=AXIS2_PLACEMENT_3D('',#44576,#34234,#34235);
#28901=AXIS2_PLACEMENT_3D('',#44579,#34237,#34238);
#28902=AXIS2_PLACEMENT_3D('',#44580,#34239,#34240);
#28903=AXIS2_PLACEMENT_3D('',#44586,#34244,#34245);
#28904=AXIS2_PLACEMENT_3D('',#44590,#34248,#34249);
#28905=AXIS2_PLACEMENT_3D('',#44594,#34252,#34253);
#28906=AXIS2_PLACEMENT_3D('',#44596,#34254,#34255);
#28907=AXIS2_PLACEMENT_3D('',#44599,#34257,#34258);
#28908=AXIS2_PLACEMENT_3D('',#44600,#34259,#34260);
#28909=AXIS2_PLACEMENT_3D('',#44601,#34261,#34262);
#28910=AXIS2_PLACEMENT_3D('',#44604,#34265,#34266);
#28911=AXIS2_PLACEMENT_3D('',#44605,#34267,#34268);
#28912=AXIS2_PLACEMENT_3D('',#44606,#34269,#34270);
#28913=AXIS2_PLACEMENT_3D('',#44607,#34271,#34272);
#28914=AXIS2_PLACEMENT_3D('',#44611,#34274,#34275);
#28915=AXIS2_PLACEMENT_3D('',#44613,#34277,#34278);
#28916=AXIS2_PLACEMENT_3D('',#44617,#34281,#34282);
#28917=AXIS2_PLACEMENT_3D('',#44619,#34284,#34285);
#28918=AXIS2_PLACEMENT_3D('',#44625,#34289,#34290);
#28919=AXIS2_PLACEMENT_3D('',#44629,#34293,#34294);
#28920=AXIS2_PLACEMENT_3D('',#44631,#34296,#34297);
#28921=AXIS2_PLACEMENT_3D('',#44632,#34298,#34299);
#28922=AXIS2_PLACEMENT_3D('',#44634,#34301,#34302);
#28923=AXIS2_PLACEMENT_3D('',#44636,#34304,#34305);
#28924=AXIS2_PLACEMENT_3D('',#44637,#34306,#34307);
#28925=AXIS2_PLACEMENT_3D('',#44638,#34308,#34309);
#28926=AXIS2_PLACEMENT_3D('',#44640,#34311,#34312);
#28927=AXIS2_PLACEMENT_3D('',#44641,#34313,#34314);
#28928=AXIS2_PLACEMENT_3D('',#44642,#34315,#34316);
#28929=AXIS2_PLACEMENT_3D('',#44648,#34320,#34321);
#28930=AXIS2_PLACEMENT_3D('',#44650,#34323,#34324);
#28931=AXIS2_PLACEMENT_3D('',#44652,#34326,#34327);
#28932=AXIS2_PLACEMENT_3D('',#44653,#34328,#34329);
#28933=AXIS2_PLACEMENT_3D('',#44654,#34330,#34331);
#28934=AXIS2_PLACEMENT_3D('',#44660,#34335,#34336);
#28935=AXIS2_PLACEMENT_3D('',#44662,#34338,#34339);
#28936=AXIS2_PLACEMENT_3D('',#44664,#34341,#34342);
#28937=AXIS2_PLACEMENT_3D('',#44665,#34343,#34344);
#28938=AXIS2_PLACEMENT_3D('',#44666,#34345,#34346);
#28939=AXIS2_PLACEMENT_3D('',#44668,#34348,#34349);
#28940=AXIS2_PLACEMENT_3D('',#44669,#34350,#34351);
#28941=AXIS2_PLACEMENT_3D('',#44670,#34352,#34353);
#28942=AXIS2_PLACEMENT_3D('',#44676,#34357,#34358);
#28943=AXIS2_PLACEMENT_3D('',#44678,#34360,#34361);
#28944=AXIS2_PLACEMENT_3D('',#44680,#34363,#34364);
#28945=AXIS2_PLACEMENT_3D('',#44681,#34365,#34366);
#28946=AXIS2_PLACEMENT_3D('',#44682,#34367,#34368);
#28947=AXIS2_PLACEMENT_3D('',#44684,#34370,#34371);
#28948=AXIS2_PLACEMENT_3D('',#44685,#34372,#34373);
#28949=AXIS2_PLACEMENT_3D('',#44686,#34374,#34375);
#28950=AXIS2_PLACEMENT_3D('',#44692,#34379,#34380);
#28951=AXIS2_PLACEMENT_3D('',#44694,#34382,#34383);
#28952=AXIS2_PLACEMENT_3D('',#44696,#34385,#34386);
#28953=AXIS2_PLACEMENT_3D('',#44697,#34387,#34388);
#28954=AXIS2_PLACEMENT_3D('',#44698,#34389,#34390);
#28955=AXIS2_PLACEMENT_3D('',#44700,#34392,#34393);
#28956=AXIS2_PLACEMENT_3D('',#44701,#34394,#34395);
#28957=AXIS2_PLACEMENT_3D('',#44702,#34396,#34397);
#28958=AXIS2_PLACEMENT_3D('',#44708,#34401,#34402);
#28959=AXIS2_PLACEMENT_3D('',#44710,#34404,#34405);
#28960=AXIS2_PLACEMENT_3D('',#44712,#34407,#34408);
#28961=AXIS2_PLACEMENT_3D('',#44713,#34409,#34410);
#28962=AXIS2_PLACEMENT_3D('',#44714,#34411,#34412);
#28963=AXIS2_PLACEMENT_3D('',#44720,#34416,#34417);
#28964=AXIS2_PLACEMENT_3D('',#44722,#34419,#34420);
#28965=AXIS2_PLACEMENT_3D('',#44724,#34422,#34423);
#28966=AXIS2_PLACEMENT_3D('',#44725,#34424,#34425);
#28967=AXIS2_PLACEMENT_3D('',#44726,#34426,#34427);
#28968=AXIS2_PLACEMENT_3D('',#44728,#34429,#34430);
#28969=AXIS2_PLACEMENT_3D('',#44729,#34431,#34432);
#28970=AXIS2_PLACEMENT_3D('',#44730,#34433,#34434);
#28971=AXIS2_PLACEMENT_3D('',#44736,#34438,#34439);
#28972=AXIS2_PLACEMENT_3D('',#44738,#34441,#34442);
#28973=AXIS2_PLACEMENT_3D('',#44740,#34444,#34445);
#28974=AXIS2_PLACEMENT_3D('',#44741,#34446,#34447);
#28975=AXIS2_PLACEMENT_3D('',#44742,#34448,#34449);
#28976=AXIS2_PLACEMENT_3D('',#44744,#34451,#34452);
#28977=AXIS2_PLACEMENT_3D('',#44745,#34453,#34454);
#28978=AXIS2_PLACEMENT_3D('',#44746,#34455,#34456);
#28979=AXIS2_PLACEMENT_3D('',#44752,#34460,#34461);
#28980=AXIS2_PLACEMENT_3D('',#44754,#34463,#34464);
#28981=AXIS2_PLACEMENT_3D('',#44756,#34466,#34467);
#28982=AXIS2_PLACEMENT_3D('',#44757,#34468,#34469);
#28983=AXIS2_PLACEMENT_3D('',#44758,#34470,#34471);
#28984=AXIS2_PLACEMENT_3D('',#44760,#34473,#34474);
#28985=AXIS2_PLACEMENT_3D('',#44761,#34475,#34476);
#28986=AXIS2_PLACEMENT_3D('',#44762,#34477,#34478);
#28987=AXIS2_PLACEMENT_3D('',#44768,#34482,#34483);
#28988=AXIS2_PLACEMENT_3D('',#44770,#34485,#34486);
#28989=AXIS2_PLACEMENT_3D('',#44772,#34488,#34489);
#28990=AXIS2_PLACEMENT_3D('',#44773,#34490,#34491);
#28991=AXIS2_PLACEMENT_3D('',#44774,#34492,#34493);
#28992=AXIS2_PLACEMENT_3D('',#44776,#34495,#34496);
#28993=AXIS2_PLACEMENT_3D('',#44777,#34497,#34498);
#28994=AXIS2_PLACEMENT_3D('',#44778,#34499,#34500);
#28995=AXIS2_PLACEMENT_3D('',#44784,#34504,#34505);
#28996=AXIS2_PLACEMENT_3D('',#44786,#34507,#34508);
#28997=AXIS2_PLACEMENT_3D('',#44788,#34510,#34511);
#28998=AXIS2_PLACEMENT_3D('',#44789,#34512,#34513);
#28999=AXIS2_PLACEMENT_3D('',#44790,#34514,#34515);
#29000=AXIS2_PLACEMENT_3D('',#44792,#34517,#34518);
#29001=AXIS2_PLACEMENT_3D('',#44793,#34519,#34520);
#29002=AXIS2_PLACEMENT_3D('',#44795,#34522,#34523);
#29003=AXIS2_PLACEMENT_3D('',#44796,#34524,#34525);
#29004=AXIS2_PLACEMENT_3D('',#44802,#34529,#34530);
#29005=AXIS2_PLACEMENT_3D('',#44804,#34532,#34533);
#29006=AXIS2_PLACEMENT_3D('',#44806,#34535,#34536);
#29007=AXIS2_PLACEMENT_3D('',#44807,#34537,#34538);
#29008=AXIS2_PLACEMENT_3D('',#44808,#34539,#34540);
#29009=AXIS2_PLACEMENT_3D('',#44810,#34542,#34543);
#29010=AXIS2_PLACEMENT_3D('',#44811,#34544,#34545);
#29011=AXIS2_PLACEMENT_3D('',#44812,#34546,#34547);
#29012=AXIS2_PLACEMENT_3D('',#44818,#34551,#34552);
#29013=AXIS2_PLACEMENT_3D('',#44820,#34554,#34555);
#29014=AXIS2_PLACEMENT_3D('',#44822,#34557,#34558);
#29015=AXIS2_PLACEMENT_3D('',#44823,#34559,#34560);
#29016=AXIS2_PLACEMENT_3D('',#44824,#34561,#34562);
#29017=AXIS2_PLACEMENT_3D('',#44830,#34566,#34567);
#29018=AXIS2_PLACEMENT_3D('',#44832,#34569,#34570);
#29019=AXIS2_PLACEMENT_3D('',#44834,#34572,#34573);
#29020=AXIS2_PLACEMENT_3D('',#44835,#34574,#34575);
#29021=AXIS2_PLACEMENT_3D('',#44837,#34577,#34578);
#29022=AXIS2_PLACEMENT_3D('',#44838,#34579,#34580);
#29023=AXIS2_PLACEMENT_3D('',#44840,#34582,#34583);
#29024=AXIS2_PLACEMENT_3D('',#44841,#34584,#34585);
#29025=AXIS2_PLACEMENT_3D('',#44845,#34588,#34589);
#29026=AXIS2_PLACEMENT_3D('',#44849,#34592,#34593);
#29027=AXIS2_PLACEMENT_3D('',#44851,#34595,#34596);
#29028=AXIS2_PLACEMENT_3D('',#44852,#34597,#34598);
#29029=AXIS2_PLACEMENT_3D('',#44858,#34602,#34603);
#29030=AXIS2_PLACEMENT_3D('',#44860,#34605,#34606);
#29031=AXIS2_PLACEMENT_3D('',#44862,#34608,#34609);
#29032=AXIS2_PLACEMENT_3D('',#44863,#34610,#34611);
#29033=AXIS2_PLACEMENT_3D('',#44867,#34614,#34615);
#29034=AXIS2_PLACEMENT_3D('',#44871,#34618,#34619);
#29035=AXIS2_PLACEMENT_3D('',#44873,#34621,#34622);
#29036=AXIS2_PLACEMENT_3D('',#44874,#34623,#34624);
#29037=AXIS2_PLACEMENT_3D('',#44876,#34626,#34627);
#29038=AXIS2_PLACEMENT_3D('',#44877,#34628,#34629);
#29039=AXIS2_PLACEMENT_3D('',#44881,#34632,#34633);
#29040=AXIS2_PLACEMENT_3D('',#44885,#34636,#34637);
#29041=AXIS2_PLACEMENT_3D('',#44887,#34639,#34640);
#29042=AXIS2_PLACEMENT_3D('',#44888,#34641,#34642);
#29043=AXIS2_PLACEMENT_3D('',#44894,#34646,#34647);
#29044=AXIS2_PLACEMENT_3D('',#44896,#34649,#34650);
#29045=AXIS2_PLACEMENT_3D('',#44898,#34652,#34653);
#29046=AXIS2_PLACEMENT_3D('',#44899,#34654,#34655);
#29047=AXIS2_PLACEMENT_3D('',#44903,#34658,#34659);
#29048=AXIS2_PLACEMENT_3D('',#44907,#34662,#34663);
#29049=AXIS2_PLACEMENT_3D('',#44909,#34665,#34666);
#29050=AXIS2_PLACEMENT_3D('',#44910,#34667,#34668);
#29051=AXIS2_PLACEMENT_3D('',#44912,#34670,#34671);
#29052=AXIS2_PLACEMENT_3D('',#44913,#34672,#34673);
#29053=AXIS2_PLACEMENT_3D('',#44917,#34676,#34677);
#29054=AXIS2_PLACEMENT_3D('',#44921,#34680,#34681);
#29055=AXIS2_PLACEMENT_3D('',#44923,#34683,#34684);
#29056=AXIS2_PLACEMENT_3D('',#44924,#34685,#34686);
#29057=AXIS2_PLACEMENT_3D('',#44930,#34690,#34691);
#29058=AXIS2_PLACEMENT_3D('',#44932,#34693,#34694);
#29059=AXIS2_PLACEMENT_3D('',#44934,#34696,#34697);
#29060=AXIS2_PLACEMENT_3D('',#44935,#34698,#34699);
#29061=AXIS2_PLACEMENT_3D('',#44939,#34702,#34703);
#29062=AXIS2_PLACEMENT_3D('',#44943,#34706,#34707);
#29063=AXIS2_PLACEMENT_3D('',#44945,#34709,#34710);
#29064=AXIS2_PLACEMENT_3D('',#44946,#34711,#34712);
#29065=AXIS2_PLACEMENT_3D('',#44952,#34716,#34717);
#29066=AXIS2_PLACEMENT_3D('',#44954,#34719,#34720);
#29067=AXIS2_PLACEMENT_3D('',#44956,#34722,#34723);
#29068=AXIS2_PLACEMENT_3D('',#44957,#34724,#34725);
#32389=DIRECTION('axis',(0.,0.,1.));
#32390=DIRECTION('refdir',(1.,0.,0.));
#32391=DIRECTION('center_axis',(-0.612372435695795,0.707106781186547,0.353553390593274));
#32392=DIRECTION('ref_axis',(0.5,0.,0.866025403784439));
#32393=DIRECTION('center_axis',(-0.612372435695795,0.707106781186547,0.353553390593274));
#32394=DIRECTION('ref_axis',(-0.612372435695794,-0.707106781186548,0.353553390593273));
#32395=DIRECTION('',(0.5,0.,0.866025403784439));
#32396=DIRECTION('',(-0.788675134594812,-0.577350269189626,-0.211324865405189));
#32397=DIRECTION('',(-0.5,0.,-0.866025403784439));
#32398=DIRECTION('center_axis',(0.866025403784439,0.,-0.5));
#32399=DIRECTION('ref_axis',(0.5,0.,0.866025403784439));
#32400=DIRECTION('',(0.,1.,0.));
#32401=DIRECTION('',(0.5,0.,0.866025403784439));
#32402=DIRECTION('',(0.,-1.,0.));
#32403=DIRECTION('center_axis',(0.,1.,0.));
#32404=DIRECTION('ref_axis',(0.,0.,1.));
#32405=DIRECTION('center_axis',(0.,1.,0.));
#32406=DIRECTION('ref_axis',(1.,0.,0.));
#32407=DIRECTION('center_axis',(0.672498511963959,0.707106781186546,-0.218508012224411));
#32408=DIRECTION('ref_axis',(-0.672498511963956,0.707106781186549,0.21850801222441));
#32409=DIRECTION('',(0.,-1.,0.));
#32410=DIRECTION('center_axis',(0.,-1.,0.));
#32411=DIRECTION('ref_axis',(0.,0.,1.));
#32412=DIRECTION('',(0.,1.,0.));
#32413=DIRECTION('center_axis',(-0.672498511963953,0.707106781186552,0.218508012224409));
#32414=DIRECTION('ref_axis',(-0.672498511963962,-0.707106781186543,0.218508012224412));
#32415=DIRECTION('center_axis',(0.,1.,0.));
#32416=DIRECTION('ref_axis',(1.,0.,0.));
#32417=DIRECTION('center_axis',(0.703233176253404,0.707106781186548,-0.0739127852035666));
#32418=DIRECTION('ref_axis',(-0.703233176253404,0.707106781186547,0.0739127852035666));
#32419=DIRECTION('',(0.,-1.,0.));
#32420=DIRECTION('center_axis',(0.,-1.,0.));
#32421=DIRECTION('ref_axis',(0.,0.,1.));
#32422=DIRECTION('',(0.,1.,0.));
#32423=DIRECTION('center_axis',(-0.703233176253404,0.707106781186547,0.0739127852035666));
#32424=DIRECTION('ref_axis',(-0.703233176253404,-0.707106781186548,0.0739127852035665));
#32425=DIRECTION('center_axis',(0.,1.,0.));
#32426=DIRECTION('ref_axis',(1.,0.,0.));
#32427=DIRECTION('',(0.,-1.,0.));
#32428=DIRECTION('center_axis',(0.,1.,0.));
#32429=DIRECTION('ref_axis',(1.,0.,0.));
#32430=DIRECTION('center_axis',(-0.703233176253403,-0.707106781186549,0.0739127852035665));
#32431=DIRECTION('ref_axis',(-0.703233176253406,0.707106781186546,0.0739127852035667));
#32432=DIRECTION('',(0.,1.,0.));
#32433=DIRECTION('center_axis',(0.,1.,0.));
#32434=DIRECTION('ref_axis',(0.,0.,1.));
#32435=DIRECTION('',(0.,-1.,0.));
#32436=DIRECTION('center_axis',(0.703233176253405,-0.707106781186546,-0.0739127852035667));
#32437=DIRECTION('ref_axis',(-0.703233176253403,-0.707106781186549,0.0739127852035666));
#32438=DIRECTION('center_axis',(0.,1.,0.));
#32439=DIRECTION('ref_axis',(1.,0.,0.));
#32440=DIRECTION('center_axis',(-0.672498511963956,-0.70710678118655,0.21850801222441));
#32441=DIRECTION('ref_axis',(-0.672498511963959,0.707106781186545,0.218508012224411));
#32442=DIRECTION('',(0.,1.,0.));
#32443=DIRECTION('center_axis',(0.,1.,0.));
#32444=DIRECTION('ref_axis',(0.,0.,1.));
#32445=DIRECTION('',(0.,-1.,0.));
#32446=DIRECTION('center_axis',(0.672498511963956,-0.707106781186549,-0.21850801222441));
#32447=DIRECTION('ref_axis',(-0.672498511963959,-0.707106781186546,0.218508012224411));
#32448=DIRECTION('center_axis',(0.,1.,0.));
#32449=DIRECTION('ref_axis',(1.,0.,0.));
#32450=DIRECTION('center_axis',(-0.612372435695791,-0.707106781186552,0.353553390593272));
#32451=DIRECTION('ref_axis',(-0.612372435695798,0.707106781186543,0.353553390593276));
#32452=DIRECTION('',(0.,1.,0.));
#32453=DIRECTION('center_axis',(0.,1.,0.));
#32454=DIRECTION('ref_axis',(0.,0.,1.));
#32455=DIRECTION('',(0.,-1.,0.));
#32456=DIRECTION('center_axis',(0.612372435695794,-0.707106781186548,-0.353553390593274));
#32457=DIRECTION('ref_axis',(-0.612372435695795,-0.707106781186547,0.353553390593274));
#32458=DIRECTION('center_axis',(0.,1.,0.));
#32459=DIRECTION('ref_axis',(1.,0.,0.));
#32460=DIRECTION('center_axis',(-0.525482745498768,-0.707106781186536,0.473146789255823));
#32461=DIRECTION('ref_axis',(-0.52548274549875,0.707106781186559,0.473146789255807));
#32462=DIRECTION('',(0.,1.,0.));
#32463=DIRECTION('center_axis',(0.,1.,0.));
#32464=DIRECTION('ref_axis',(0.,0.,1.));
#32465=DIRECTION('',(0.,-1.,0.));
#32466=DIRECTION('center_axis',(0.525482745498765,-0.70710678118654,-0.47314678925582));
#32467=DIRECTION('ref_axis',(-0.525482745498753,-0.707106781186555,0.47314678925581));
#32468=DIRECTION('center_axis',(0.,1.,0.));
#32469=DIRECTION('ref_axis',(1.,0.,0.));
#32470=DIRECTION('center_axis',(-0.415626937777454,-0.707106781186547,0.572061402817684));
#32471=DIRECTION('ref_axis',(-0.415626937777453,0.707106781186548,0.572061402817684));
#32472=DIRECTION('',(0.,1.,0.));
#32473=DIRECTION('center_axis',(0.,1.,0.));
#32474=DIRECTION('ref_axis',(0.,0.,1.));
#32475=DIRECTION('',(0.,-1.,0.));
#32476=DIRECTION('center_axis',(0.415626937777452,-0.707106781186551,-0.572061402817682));
#32477=DIRECTION('ref_axis',(-0.415626937777455,-0.707106781186544,0.572061402817687));
#32478=DIRECTION('center_axis',(0.,1.,0.));
#32479=DIRECTION('ref_axis',(1.,0.,0.));
#32480=DIRECTION('center_axis',(-0.287606238475956,-0.707106781186536,0.645974188021262));
#32481=DIRECTION('ref_axis',(-0.287606238475946,0.707106781186559,0.64597418802124));
#32482=DIRECTION('',(0.,1.,0.));
#32483=DIRECTION('center_axis',(0.,1.,0.));
#32484=DIRECTION('ref_axis',(0.,0.,1.));
#32485=DIRECTION('',(0.,-1.,0.));
#32486=DIRECTION('center_axis',(0.287606238475952,-0.707106781186546,-0.645974188021253));
#32487=DIRECTION('ref_axis',(-0.28760623847595,-0.707106781186549,0.645974188021249));
#32488=DIRECTION('center_axis',(0.,1.,0.));
#32489=DIRECTION('ref_axis',(1.,0.,0.));
#32490=DIRECTION('center_axis',(-0.147015766465198,-0.707106781186553,0.69165480148022));
#32491=DIRECTION('ref_axis',(-0.1470157664652,0.707106781186542,0.691654801480231));
#32492=DIRECTION('',(0.,1.,0.));
#32493=DIRECTION('center_axis',(0.,1.,0.));
#32494=DIRECTION('ref_axis',(0.,0.,1.));
#32495=DIRECTION('',(0.,-1.,0.));
#32496=DIRECTION('center_axis',(0.1470157664652,-0.707106781186543,-0.69165480148023));
#32497=DIRECTION('ref_axis',(-0.147015766465198,-0.707106781186552,0.691654801480221));
#32498=DIRECTION('center_axis',(0.,1.,0.));
#32499=DIRECTION('ref_axis',(1.,0.,0.));
#32500=DIRECTION('center_axis',(-8.65956056235491E-17,-0.707106781186549,
0.707106781186546));
#32501=DIRECTION('ref_axis',(0.,0.707106781186546,0.70710678118655));
#32502=DIRECTION('',(0.,1.,0.));
#32503=DIRECTION('center_axis',(0.,1.,0.));
#32504=DIRECTION('ref_axis',(0.,0.,1.));
#32505=DIRECTION('',(0.,-1.,0.));
#32506=DIRECTION('center_axis',(8.65956056235492E-17,-0.707106781186549,
-0.707106781186546));
#32507=DIRECTION('ref_axis',(0.,-0.707106781186546,0.707106781186549));
#32508=DIRECTION('center_axis',(0.,1.,0.));
#32509=DIRECTION('ref_axis',(1.,0.,0.));
#32510=DIRECTION('center_axis',(0.147015766465198,-0.707106781186549,0.691654801480225));
#32511=DIRECTION('ref_axis',(0.147015766465198,0.707106781186547,0.691654801480227));
#32512=DIRECTION('',(0.,1.,0.));
#32513=DIRECTION('center_axis',(0.,1.,0.));
#32514=DIRECTION('ref_axis',(0.,0.,1.));
#32515=DIRECTION('',(0.,-1.,0.));
#32516=DIRECTION('center_axis',(-0.147015766465198,-0.707106781186548,-0.691654801480226));
#32517=DIRECTION('ref_axis',(0.147015766465198,-0.707106781186547,0.691654801480226));
#32518=DIRECTION('center_axis',(0.,1.,0.));
#32519=DIRECTION('ref_axis',(1.,0.,0.));
#32520=DIRECTION('center_axis',(0.287606238475948,-0.707106781186554,0.645974188021245));
#32521=DIRECTION('ref_axis',(0.287606238475953,0.707106781186541,0.645974188021257));
#32522=DIRECTION('',(0.,1.,0.));
#32523=DIRECTION('center_axis',(0.,1.,0.));
#32524=DIRECTION('ref_axis',(0.,0.,1.));
#32525=DIRECTION('',(0.,-1.,0.));
#32526=DIRECTION('center_axis',(-0.28760623847595,-0.707106781186549,-0.64597418802125));
#32527=DIRECTION('ref_axis',(0.287606238475951,-0.707106781186546,0.645974188021252));
#32528=DIRECTION('center_axis',(0.,1.,0.));
#32529=DIRECTION('ref_axis',(1.,0.,0.));
#32530=DIRECTION('center_axis',(0.415626937777451,-0.707106781186552,0.572061402817681));
#32531=DIRECTION('ref_axis',(0.415626937777456,0.707106781186543,0.572061402817688));
#32532=DIRECTION('',(0.,1.,0.));
#32533=DIRECTION('center_axis',(0.,1.,0.));
#32534=DIRECTION('ref_axis',(0.,0.,1.));
#32535=DIRECTION('',(0.,-1.,0.));
#32536=DIRECTION('center_axis',(-0.415626937777457,-0.707106781186541,-0.57206140281769));
#32537=DIRECTION('ref_axis',(0.415626937777449,-0.707106781186554,0.572061402817679));
#32538=DIRECTION('center_axis',(0.,1.,0.));
#32539=DIRECTION('ref_axis',(1.,0.,0.));
#32540=DIRECTION('center_axis',(0.525482745498763,-0.707106781186542,0.473146789255819));
#32541=DIRECTION('ref_axis',(0.525482745498754,0.707106781186554,0.473146789255811));
#32542=DIRECTION('',(0.,1.,0.));
#32543=DIRECTION('center_axis',(0.,1.,0.));
#32544=DIRECTION('ref_axis',(0.,0.,1.));
#32545=DIRECTION('',(0.,-1.,0.));
#32546=DIRECTION('center_axis',(-0.525482745498763,-0.707106781186542,-0.473146789255819));
#32547=DIRECTION('ref_axis',(0.525482745498754,-0.707106781186554,0.473146789255811));
#32548=DIRECTION('center_axis',(0.,1.,0.));
#32549=DIRECTION('ref_axis',(1.,0.,0.));
#32550=DIRECTION('center_axis',(0.612372435695789,-0.707106781186554,0.353553390593271));
#32551=DIRECTION('ref_axis',(0.6123724356958,0.707106781186541,0.353553390593277));
#32552=DIRECTION('',(0.,1.,0.));
#32553=DIRECTION('center_axis',(0.,1.,0.));
#32554=DIRECTION('ref_axis',(0.,0.,1.));
#32555=DIRECTION('',(0.,-1.,0.));
#32556=DIRECTION('center_axis',(-0.612372435695789,-0.707106781186554,-0.353553390593271));
#32557=DIRECTION('ref_axis',(0.6123724356958,-0.707106781186541,0.353553390593277));
#32558=DIRECTION('center_axis',(0.,1.,0.));
#32559=DIRECTION('ref_axis',(1.,0.,0.));
#32560=DIRECTION('center_axis',(0.672498511963956,-0.707106781186549,0.21850801222441));
#32561=DIRECTION('ref_axis',(0.672498511963959,0.707106781186546,0.218508012224411));
#32562=DIRECTION('',(0.,1.,0.));
#32563=DIRECTION('center_axis',(0.,1.,0.));
#32564=DIRECTION('ref_axis',(0.,0.,1.));
#32565=DIRECTION('',(0.,-1.,0.));
#32566=DIRECTION('center_axis',(-0.672498511963956,-0.707106781186549,-0.21850801222441));
#32567=DIRECTION('ref_axis',(0.672498511963959,-0.707106781186546,0.218508012224411));
#32568=DIRECTION('center_axis',(0.,1.,0.));
#32569=DIRECTION('ref_axis',(1.,0.,0.));
#32570=DIRECTION('center_axis',(0.703233176253405,-0.707106781186547,0.0739127852035674));
#32571=DIRECTION('ref_axis',(0.703233176253403,0.707106781186548,0.0739127852035672));
#32572=DIRECTION('',(0.,1.,0.));
#32573=DIRECTION('center_axis',(0.,1.,0.));
#32574=DIRECTION('ref_axis',(0.,0.,1.));
#32575=DIRECTION('',(0.,-1.,0.));
#32576=DIRECTION('center_axis',(-0.703233176253405,-0.707106781186547,-0.0739127852035674));
#32577=DIRECTION('ref_axis',(0.703233176253403,-0.707106781186548,0.0739127852035672));
#32578=DIRECTION('center_axis',(0.,1.,0.));
#32579=DIRECTION('ref_axis',(1.,0.,0.));
#32580=DIRECTION('center_axis',(0.703233176253406,-0.707106781186546,-0.0739127852035666));
#32581=DIRECTION('ref_axis',(-0.703233176253402,-0.707106781186549,0.0739127852035662));
#32582=DIRECTION('',(0.,1.,0.));
#32583=DIRECTION('center_axis',(0.,1.,0.));
#32584=DIRECTION('ref_axis',(0.,0.,1.));
#32585=DIRECTION('',(0.,-1.,0.));
#32586=DIRECTION('center_axis',(-0.703233176253405,-0.707106781186547,0.0739127852035665));
#32587=DIRECTION('ref_axis',(-0.703233176253403,0.707106781186548,0.0739127852035663));
#32588=DIRECTION('center_axis',(0.,1.,0.));
#32589=DIRECTION('ref_axis',(1.,0.,0.));
#32590=DIRECTION('center_axis',(0.672498511963956,-0.707106781186549,-0.21850801222441));
#32591=DIRECTION('ref_axis',(-0.672498511963959,-0.707106781186546,0.218508012224411));
#32592=DIRECTION('',(0.,1.,0.));
#32593=DIRECTION('center_axis',(0.,1.,0.));
#32594=DIRECTION('ref_axis',(0.,0.,1.));
#32595=DIRECTION('',(0.,-1.,0.));
#32596=DIRECTION('center_axis',(-0.672498511963959,-0.707106781186545,0.218508012224411));
#32597=DIRECTION('ref_axis',(-0.672498511963955,0.70710678118655,0.21850801222441));
#32598=DIRECTION('center_axis',(0.,1.,0.));
#32599=DIRECTION('ref_axis',(1.,0.,0.));
#32600=DIRECTION('center_axis',(0.612372435695792,-0.707106781186551,-0.353553390593272));
#32601=DIRECTION('ref_axis',(-0.612372435695797,-0.707106781186545,0.353553390593275));
#32602=DIRECTION('',(0.,1.,0.));
#32603=DIRECTION('center_axis',(0.,1.,0.));
#32604=DIRECTION('ref_axis',(0.,0.,1.));
#32605=DIRECTION('',(0.,-1.,0.));
#32606=DIRECTION('center_axis',(-0.612372435695802,-0.70710678118654,0.353553390593277));
#32607=DIRECTION('ref_axis',(-0.612372435695788,0.707106781186555,0.353553390593269));
#32608=DIRECTION('center_axis',(0.,1.,0.));
#32609=DIRECTION('ref_axis',(1.,0.,0.));
#32610=DIRECTION('center_axis',(0.525482745498764,-0.707106781186541,-0.473146789255819));
#32611=DIRECTION('ref_axis',(-0.525482745498755,-0.707106781186554,0.473146789255811));
#32612=DIRECTION('',(0.,1.,0.));
#32613=DIRECTION('center_axis',(0.,1.,0.));
#32614=DIRECTION('ref_axis',(0.,0.,1.));
#32615=DIRECTION('',(0.,-1.,0.));
#32616=DIRECTION('center_axis',(-0.525482745498762,-0.707106781186544,0.473146789255817));
#32617=DIRECTION('ref_axis',(-0.525482745498757,0.707106781186551,0.473146789255813));
#32618=DIRECTION('center_axis',(0.,1.,0.));
#32619=DIRECTION('ref_axis',(1.,0.,0.));
#32620=DIRECTION('center_axis',(0.415626937777451,-0.707106781186552,-0.572061402817681));
#32621=DIRECTION('ref_axis',(-0.415626937777456,-0.707106781186543,0.572061402817688));
#32622=DIRECTION('',(0.,1.,0.));
#32623=DIRECTION('center_axis',(0.,1.,0.));
#32624=DIRECTION('ref_axis',(0.,0.,1.));
#32625=DIRECTION('',(0.,-1.,0.));
#32626=DIRECTION('center_axis',(-0.415626937777453,-0.707106781186549,0.572061402817683));
#32627=DIRECTION('ref_axis',(-0.415626937777454,0.707106781186547,0.572061402817685));
#32628=DIRECTION('center_axis',(0.,1.,0.));
#32629=DIRECTION('ref_axis',(1.,0.,0.));
#32630=DIRECTION('center_axis',(0.287606238475947,-0.707106781186558,-0.645974188021242));
#32631=DIRECTION('ref_axis',(-0.287606238475955,-0.707106781186537,0.64597418802126));
#32632=DIRECTION('',(0.,1.,0.));
#32633=DIRECTION('center_axis',(0.,1.,0.));
#32634=DIRECTION('ref_axis',(0.,0.,1.));
#32635=DIRECTION('',(0.,-1.,0.));
#32636=DIRECTION('center_axis',(-0.287606238475954,-0.70710678118654,0.645974188021258));
#32637=DIRECTION('ref_axis',(-0.287606238475948,0.707106781186555,0.645974188021244));
#32638=DIRECTION('center_axis',(0.,1.,0.));
#32639=DIRECTION('ref_axis',(1.,0.,0.));
#32640=DIRECTION('center_axis',(0.147015766465199,-0.707106781186549,-0.691654801480225));
#32641=DIRECTION('ref_axis',(-0.147015766465199,-0.707106781186547,0.691654801480227));
#32642=DIRECTION('',(0.,1.,0.));
#32643=DIRECTION('center_axis',(0.,1.,0.));
#32644=DIRECTION('ref_axis',(0.,0.,1.));
#32645=DIRECTION('',(0.,-1.,0.));
#32646=DIRECTION('center_axis',(-0.1470157664652,-0.707106781186542,0.69165480148023));
#32647=DIRECTION('ref_axis',(-0.147015766465198,0.707106781186553,0.691654801480221));
#32648=DIRECTION('center_axis',(0.,1.,0.));
#32649=DIRECTION('ref_axis',(1.,0.,0.));
#32650=DIRECTION('center_axis',(0.,-0.707106781186549,-0.707106781186546));
#32651=DIRECTION('ref_axis',(0.,-0.707106781186546,0.707106781186549));
#32652=DIRECTION('',(0.,1.,0.));
#32653=DIRECTION('center_axis',(0.,1.,0.));
#32654=DIRECTION('ref_axis',(0.,0.,1.));
#32655=DIRECTION('',(0.,-1.,0.));
#32656=DIRECTION('center_axis',(0.,-0.707106781186549,0.707106781186546));
#32657=DIRECTION('ref_axis',(0.,0.707106781186546,0.707106781186549));
#32658=DIRECTION('center_axis',(0.,1.,0.));
#32659=DIRECTION('ref_axis',(1.,0.,0.));
#32660=DIRECTION('center_axis',(-0.147015766465198,-0.70710678118655,-0.691654801480224));
#32661=DIRECTION('ref_axis',(0.147015766465199,-0.707106781186545,0.691654801480228));
#32662=DIRECTION('',(0.,1.,0.));
#32663=DIRECTION('center_axis',(0.,1.,0.));
#32664=DIRECTION('ref_axis',(0.,0.,1.));
#32665=DIRECTION('',(0.,-1.,0.));
#32666=DIRECTION('center_axis',(0.147015766465198,-0.707106781186549,0.691654801480225));
#32667=DIRECTION('ref_axis',(0.147015766465199,0.707106781186547,0.691654801480227));
#32668=DIRECTION('center_axis',(0.,1.,0.));
#32669=DIRECTION('ref_axis',(1.,0.,0.));
#32670=DIRECTION('center_axis',(-0.287606238475955,-0.707106781186538,-0.64597418802126));
#32671=DIRECTION('ref_axis',(0.287606238475947,-0.707106781186557,0.645974188021242));
#32672=DIRECTION('',(0.,1.,0.));
#32673=DIRECTION('center_axis',(0.,1.,0.));
#32674=DIRECTION('ref_axis',(0.,0.,1.));
#32675=DIRECTION('',(0.,-1.,0.));
#32676=DIRECTION('center_axis',(0.287606238475944,-0.707106781186565,0.645974188021235));
#32677=DIRECTION('ref_axis',(0.287606238475958,0.70710678118653,0.645974188021267));
#32678=DIRECTION('center_axis',(0.,1.,0.));
#32679=DIRECTION('ref_axis',(1.,0.,0.));
#32680=DIRECTION('center_axis',(-0.415626937777456,-0.707106781186543,-0.572061402817688));
#32681=DIRECTION('ref_axis',(0.415626937777451,-0.707106781186551,0.572061402817681));
#32682=DIRECTION('',(0.,1.,0.));
#32683=DIRECTION('center_axis',(0.,1.,0.));
#32684=DIRECTION('ref_axis',(0.,0.,1.));
#32685=DIRECTION('',(0.,-1.,0.));
#32686=DIRECTION('center_axis',(0.415626937777451,-0.707106781186551,0.572061402817681));
#32687=DIRECTION('ref_axis',(0.415626937777455,0.707106781186544,0.572061402817687));
#32688=DIRECTION('center_axis',(0.,1.,0.));
#32689=DIRECTION('ref_axis',(1.,0.,0.));
#32690=DIRECTION('center_axis',(-0.525482745498762,-0.707106781186544,-0.473146789255818));
#32691=DIRECTION('ref_axis',(0.525482745498756,-0.707106781186551,0.473146789255813));
#32692=DIRECTION('',(0.,1.,0.));
#32693=DIRECTION('center_axis',(0.,1.,0.));
#32694=DIRECTION('ref_axis',(0.,0.,1.));
#32695=DIRECTION('',(0.,-1.,0.));
#32696=DIRECTION('center_axis',(0.525482745498748,-0.707106781186563,0.473146789255805));
#32697=DIRECTION('ref_axis',(0.52548274549877,0.707106781186532,0.473146789255825));
#32698=DIRECTION('center_axis',(0.,1.,0.));
#32699=DIRECTION('ref_axis',(1.,0.,0.));
#32700=DIRECTION('center_axis',(-0.612372435695801,-0.70710678118654,-0.353553390593278));
#32701=DIRECTION('ref_axis',(0.612372435695788,-0.707106781186555,0.35355339059327));
#32702=DIRECTION('',(0.,1.,0.));
#32703=DIRECTION('center_axis',(0.,1.,0.));
#32704=DIRECTION('ref_axis',(0.,0.,1.));
#32705=DIRECTION('',(0.,-1.,0.));
#32706=DIRECTION('center_axis',(0.612372435695798,-0.707106781186544,0.353553390593276));
#32707=DIRECTION('ref_axis',(0.612372435695791,0.707106781186551,0.353553390593272));
#32708=DIRECTION('center_axis',(0.,1.,0.));
#32709=DIRECTION('ref_axis',(1.,0.,0.));
#32710=DIRECTION('center_axis',(-0.672498511963955,-0.707106781186549,-0.21850801222441));
#32711=DIRECTION('ref_axis',(0.672498511963959,-0.707106781186546,0.218508012224411));
#32712=DIRECTION('',(0.,1.,0.));
#32713=DIRECTION('center_axis',(0.,1.,0.));
#32714=DIRECTION('ref_axis',(0.,0.,1.));
#32715=DIRECTION('',(0.,-1.,0.));
#32716=DIRECTION('center_axis',(0.672498511963958,-0.707106781186547,0.218508012224411));
#32717=DIRECTION('ref_axis',(0.672498511963957,0.707106781186548,0.218508012224411));
#32718=DIRECTION('center_axis',(0.,1.,0.));
#32719=DIRECTION('ref_axis',(1.,0.,0.));
#32720=DIRECTION('center_axis',(-0.703233176253405,-0.707106781186547,-0.0739127852035669));
#32721=DIRECTION('ref_axis',(0.703233176253403,-0.707106781186548,0.0739127852035668));
#32722=DIRECTION('',(0.,1.,0.));
#32723=DIRECTION('center_axis',(0.,1.,0.));
#32724=DIRECTION('ref_axis',(0.,0.,1.));
#32725=DIRECTION('',(0.,-1.,0.));
#32726=DIRECTION('center_axis',(0.703233176253404,-0.707106781186547,0.0739127852035669));
#32727=DIRECTION('ref_axis',(0.703233176253404,0.707106781186548,0.0739127852035668));
#32728=DIRECTION('center_axis',(0.,1.,0.));
#32729=DIRECTION('ref_axis',(1.,0.,0.));
#32730=DIRECTION('center_axis',(0.,1.,0.));
#32731=DIRECTION('ref_axis',(1.,0.,0.));
#32732=DIRECTION('center_axis',(0.703233176253406,0.707106781186546,0.073912785203567));
#32733=DIRECTION('ref_axis',(0.703233176253403,-0.707106781186549,0.0739127852035667));
#32734=DIRECTION('',(0.,-1.,0.));
#32735=DIRECTION('center_axis',(0.,-1.,0.));
#32736=DIRECTION('ref_axis',(0.,0.,1.));
#32737=DIRECTION('',(0.,1.,0.));
#32738=DIRECTION('center_axis',(-0.703233176253405,0.707106781186547,-0.0739127852035669));
#32739=DIRECTION('ref_axis',(0.703233176253403,0.707106781186548,0.0739127852035668));
#32740=DIRECTION('center_axis',(0.,1.,0.));
#32741=DIRECTION('ref_axis',(1.,0.,0.));
#32742=DIRECTION('center_axis',(0.672498511963959,0.707106781186546,0.218508012224411));
#32743=DIRECTION('ref_axis',(0.672498511963955,-0.707106781186549,0.21850801222441));
#32744=DIRECTION('',(0.,-1.,0.));
#32745=DIRECTION('center_axis',(0.,-1.,0.));
#32746=DIRECTION('ref_axis',(0.,0.,1.));
#32747=DIRECTION('',(0.,1.,0.));
#32748=DIRECTION('center_axis',(-0.672498511963952,0.707106781186553,-0.218508012224409));
#32749=DIRECTION('ref_axis',(0.672498511963962,0.707106781186542,0.218508012224412));
#32750=DIRECTION('center_axis',(0.,1.,0.));
#32751=DIRECTION('ref_axis',(1.,0.,0.));
#32752=DIRECTION('center_axis',(0.612372435695797,0.707106781186544,0.353553390593275));
#32753=DIRECTION('ref_axis',(0.612372435695792,-0.707106781186551,0.353553390593272));
#32754=DIRECTION('',(0.,-1.,0.));
#32755=DIRECTION('center_axis',(0.,-1.,0.));
#32756=DIRECTION('ref_axis',(0.,0.,1.));
#32757=DIRECTION('',(0.,1.,0.));
#32758=DIRECTION('center_axis',(-0.612372435695796,0.707106781186545,-0.353553390593275));
#32759=DIRECTION('ref_axis',(0.612372435695792,0.70710678118655,0.353553390593273));
#32760=DIRECTION('center_axis',(0.,1.,0.));
#32761=DIRECTION('ref_axis',(1.,0.,0.));
#32762=DIRECTION('center_axis',(0.525482745498763,0.707106781186542,0.473146789255819));
#32763=DIRECTION('ref_axis',(0.525482745498754,-0.707106781186553,0.473146789255811));
#32764=DIRECTION('',(0.,-1.,0.));
#32765=DIRECTION('center_axis',(0.,-1.,0.));
#32766=DIRECTION('ref_axis',(0.,0.,1.));
#32767=DIRECTION('',(0.,1.,0.));
#32768=DIRECTION('center_axis',(-0.525482745498759,0.707106781186547,-0.473146789255815));
#32769=DIRECTION('ref_axis',(0.525482745498758,0.707106781186548,0.473146789255815));
#32770=DIRECTION('center_axis',(0.,1.,0.));
#32771=DIRECTION('ref_axis',(1.,0.,0.));
#32772=DIRECTION('center_axis',(0.415626937777452,0.707106781186551,0.572061402817682));
#32773=DIRECTION('ref_axis',(0.415626937777455,-0.707106781186544,0.572061402817687));
#32774=DIRECTION('',(0.,-1.,0.));
#32775=DIRECTION('center_axis',(0.,-1.,0.));
#32776=DIRECTION('ref_axis',(0.,0.,1.));
#32777=DIRECTION('',(0.,1.,0.));
#32778=DIRECTION('center_axis',(-0.41562693777745,0.707106781186553,-0.57206140281768));
#32779=DIRECTION('ref_axis',(0.415626937777457,0.707106781186542,0.572061402817689));
#32780=DIRECTION('center_axis',(0.,1.,0.));
#32781=DIRECTION('ref_axis',(1.,0.,0.));
#32782=DIRECTION('center_axis',(0.28760623847595,0.707106781186549,0.64597418802125));
#32783=DIRECTION('ref_axis',(0.287606238475951,-0.707106781186546,0.645974188021252));
#32784=DIRECTION('',(0.,-1.,0.));
#32785=DIRECTION('center_axis',(0.,-1.,0.));
#32786=DIRECTION('ref_axis',(0.,0.,1.));
#32787=DIRECTION('',(0.,1.,0.));
#32788=DIRECTION('center_axis',(-0.28760623847595,0.707106781186549,-0.64597418802125));
#32789=DIRECTION('ref_axis',(0.287606238475951,0.707106781186546,0.645974188021252));
#32790=DIRECTION('center_axis',(0.,1.,0.));
#32791=DIRECTION('ref_axis',(1.,0.,0.));
#32792=DIRECTION('center_axis',(0.147015766465199,0.707106781186544,0.691654801480229));
#32793=DIRECTION('ref_axis',(0.147015766465198,-0.707106781186551,0.691654801480222));
#32794=DIRECTION('',(0.,-1.,0.));
#32795=DIRECTION('center_axis',(0.,-1.,0.));
#32796=DIRECTION('ref_axis',(0.,0.,1.));
#32797=DIRECTION('',(0.,1.,0.));
#32798=DIRECTION('center_axis',(-0.147015766465199,0.707106781186546,-0.691654801480227));
#32799=DIRECTION('ref_axis',(0.147015766465198,0.707106781186549,0.691654801480224));
#32800=DIRECTION('center_axis',(0.,1.,0.));
#32801=DIRECTION('ref_axis',(1.,0.,0.));
#32802=DIRECTION('center_axis',(0.,0.707106781186547,0.707106781186548));
#32803=DIRECTION('ref_axis',(0.,-0.707106781186548,0.707106781186547));
#32804=DIRECTION('',(0.,-1.,0.));
#32805=DIRECTION('center_axis',(0.,-1.,0.));
#32806=DIRECTION('ref_axis',(0.,0.,1.));
#32807=DIRECTION('',(0.,1.,0.));
#32808=DIRECTION('center_axis',(0.,0.707106781186547,-0.707106781186548));
#32809=DIRECTION('ref_axis',(0.,0.707106781186548,0.707106781186547));
#32810=DIRECTION('center_axis',(0.,1.,0.));
#32811=DIRECTION('ref_axis',(1.,0.,0.));
#32812=DIRECTION('center_axis',(-0.147015766465199,0.707106781186546,0.691654801480227));
#32813=DIRECTION('ref_axis',(-0.147015766465199,-0.707106781186549,0.691654801480224));
#32814=DIRECTION('',(0.,-1.,0.));
#32815=DIRECTION('center_axis',(0.,-1.,0.));
#32816=DIRECTION('ref_axis',(0.,0.,1.));
#32817=DIRECTION('',(0.,1.,0.));
#32818=DIRECTION('center_axis',(0.147015766465199,0.707106781186547,-0.691654801480226));
#32819=DIRECTION('ref_axis',(-0.147015766465199,0.707106781186549,0.691654801480225));
#32820=DIRECTION('center_axis',(0.,1.,0.));
#32821=DIRECTION('ref_axis',(1.,0.,0.));
#32822=DIRECTION('center_axis',(-0.287606238475952,0.707106781186546,0.645974188021252));
#32823=DIRECTION('ref_axis',(-0.287606238475951,-0.707106781186549,0.64597418802125));
#32824=DIRECTION('',(0.,-1.,0.));
#32825=DIRECTION('center_axis',(0.,-1.,0.));
#32826=DIRECTION('ref_axis',(0.,0.,1.));
#32827=DIRECTION('',(0.,1.,0.));
#32828=DIRECTION('center_axis',(0.287606238475951,0.707106781186549,-0.64597418802125));
#32829=DIRECTION('ref_axis',(-0.287606238475952,0.707106781186546,0.645974188021252));
#32830=DIRECTION('center_axis',(0.,1.,0.));
#32831=DIRECTION('ref_axis',(1.,0.,0.));
#32832=DIRECTION('center_axis',(-0.415626937777453,0.707106781186548,0.572061402817684));
#32833=DIRECTION('ref_axis',(-0.415626937777454,-0.707106781186547,0.572061402817684));
#32834=DIRECTION('',(0.,-1.,0.));
#32835=DIRECTION('center_axis',(0.,-1.,0.));
#32836=DIRECTION('ref_axis',(0.,0.,1.));
#32837=DIRECTION('',(0.,1.,0.));
#32838=DIRECTION('center_axis',(0.415626937777454,0.707106781186546,-0.572061402817685));
#32839=DIRECTION('ref_axis',(-0.415626937777453,0.707106781186549,0.572061402817683));
#32840=DIRECTION('center_axis',(0.,1.,0.));
#32841=DIRECTION('ref_axis',(1.,0.,0.));
#32842=DIRECTION('center_axis',(-0.525482745498764,0.707106781186541,0.473146789255819));
#32843=DIRECTION('ref_axis',(-0.525482745498755,-0.707106781186554,0.473146789255811));
#32844=DIRECTION('',(0.,-1.,0.));
#32845=DIRECTION('center_axis',(0.,-1.,0.));
#32846=DIRECTION('ref_axis',(0.,0.,1.));
#32847=DIRECTION('',(0.,1.,0.));
#32848=DIRECTION('center_axis',(0.52548274549876,0.707106781186547,-0.473146789255815));
#32849=DIRECTION('ref_axis',(-0.525482745498759,0.707106781186548,0.473146789255814));
#32850=DIRECTION('center_axis',(0.,1.,0.));
#32851=DIRECTION('ref_axis',(1.,0.,0.));
#32852=DIRECTION('center_axis',(-0.612372435695797,0.707106781186545,0.353553390593274));
#32853=DIRECTION('ref_axis',(-0.612372435695793,-0.70710678118655,0.353553390593272));
#32854=DIRECTION('',(0.,-1.,0.));
#32855=DIRECTION('center_axis',(0.,-1.,0.));
#32856=DIRECTION('ref_axis',(0.,0.,1.));
#32857=DIRECTION('',(0.,1.,0.));
#32858=DIRECTION('center_axis',(0.612372435695795,0.707106781186547,-0.353553390593274));
#32859=DIRECTION('ref_axis',(-0.612372435695794,0.707106781186548,0.353553390593273));
#32860=DIRECTION('center_axis',(0.,1.,0.));
#32861=DIRECTION('ref_axis',(1.,0.,0.));
#32862=DIRECTION('center_axis',(-0.672498511963955,0.70710678118655,0.21850801222441));
#32863=DIRECTION('ref_axis',(-0.672498511963959,-0.707106781186545,0.218508012224411));
#32864=DIRECTION('',(0.,-1.,0.));
#32865=DIRECTION('center_axis',(0.,-1.,0.));
#32866=DIRECTION('ref_axis',(0.,0.,1.));
#32867=DIRECTION('',(0.,1.,0.));
#32868=DIRECTION('center_axis',(0.672498511963957,0.707106781186548,-0.21850801222441));
#32869=DIRECTION('ref_axis',(-0.672498511963958,0.707106781186547,0.218508012224411));
#32870=DIRECTION('center_axis',(0.,1.,0.));
#32871=DIRECTION('ref_axis',(1.,0.,0.));
#32872=DIRECTION('center_axis',(-0.703233176253405,0.707106781186547,0.0739127852035665));
#32873=DIRECTION('ref_axis',(-0.703233176253403,-0.707106781186548,0.0739127852035663));
#32874=DIRECTION('',(0.,-1.,0.));
#32875=DIRECTION('center_axis',(0.,-1.,0.));
#32876=DIRECTION('ref_axis',(0.,0.,1.));
#32877=DIRECTION('',(0.,1.,0.));
#32878=DIRECTION('center_axis',(0.703233176253404,0.707106781186547,-0.0739127852035664));
#32879=DIRECTION('ref_axis',(-0.703233176253404,0.707106781186548,0.0739127852035664));
#32880=DIRECTION('center_axis',(0.,1.,0.));
#32881=DIRECTION('ref_axis',(1.,0.,0.));
#32882=DIRECTION('center_axis',(-0.703233176253405,0.707106781186547,-0.0739127852035674));
#32883=DIRECTION('ref_axis',(0.703233176253403,0.707106781186548,0.0739127852035672));
#32884=DIRECTION('',(0.,-1.,0.));
#32885=DIRECTION('center_axis',(0.,-1.,0.));
#32886=DIRECTION('ref_axis',(0.,0.,1.));
#32887=DIRECTION('',(0.,1.,0.));
#32888=DIRECTION('center_axis',(0.703233176253406,0.707106781186546,0.0739127852035675));
#32889=DIRECTION('ref_axis',(0.703233176253402,-0.707106781186549,0.0739127852035671));
#32890=DIRECTION('center_axis',(0.,1.,0.));
#32891=DIRECTION('ref_axis',(1.,0.,0.));
#32892=DIRECTION('center_axis',(-0.672498511963957,0.707106781186548,-0.218508012224411));
#32893=DIRECTION('ref_axis',(0.672498511963958,0.707106781186547,0.218508012224411));
#32894=DIRECTION('',(0.,-1.,0.));
#32895=DIRECTION('center_axis',(0.,-1.,0.));
#32896=DIRECTION('ref_axis',(0.,0.,1.));
#32897=DIRECTION('',(0.,1.,0.));
#32898=DIRECTION('center_axis',(0.672498511963954,0.707106781186551,0.21850801222441));
#32899=DIRECTION('ref_axis',(0.672498511963961,-0.707106781186544,0.218508012224412));
#32900=DIRECTION('center_axis',(0.,1.,0.));
#32901=DIRECTION('ref_axis',(1.,0.,0.));
#32902=DIRECTION('center_axis',(-0.612372435695796,0.707106781186545,-0.353553390593275));
#32903=DIRECTION('ref_axis',(0.612372435695792,0.70710678118655,0.353553390593273));
#32904=DIRECTION('',(0.,-1.,0.));
#32905=DIRECTION('center_axis',(0.,-1.,0.));
#32906=DIRECTION('ref_axis',(0.,0.,1.));
#32907=DIRECTION('',(0.,1.,0.));
#32908=DIRECTION('center_axis',(0.612372435695793,0.707106781186549,0.353553390593274));
#32909=DIRECTION('ref_axis',(0.612372435695795,-0.707106781186547,0.353553390593275));
#32910=DIRECTION('center_axis',(0.,1.,0.));
#32911=DIRECTION('ref_axis',(1.,0.,0.));
#32912=DIRECTION('center_axis',(-0.525482745498762,0.707106781186543,-0.473146789255818));
#32913=DIRECTION('ref_axis',(0.525482745498755,0.707106781186552,0.473146789255812));
#32914=DIRECTION('',(0.,-1.,0.));
#32915=DIRECTION('center_axis',(0.,-1.,0.));
#32916=DIRECTION('ref_axis',(0.,0.,1.));
#32917=DIRECTION('',(0.,1.,0.));
#32918=DIRECTION('center_axis',(0.525482745498759,0.707106781186547,0.473146789255815));
#32919=DIRECTION('ref_axis',(0.525482745498758,-0.707106781186548,0.473146789255815));
#32920=DIRECTION('center_axis',(0.,1.,0.));
#32921=DIRECTION('ref_axis',(1.,0.,0.));
#32922=DIRECTION('center_axis',(-0.415626937777449,0.707106781186555,-0.572061402817678));
#32923=DIRECTION('ref_axis',(0.415626937777458,0.70710678118654,0.57206140281769));
#32924=DIRECTION('',(0.,-1.,0.));
#32925=DIRECTION('center_axis',(0.,-1.,0.));
#32926=DIRECTION('ref_axis',(0.,0.,1.));
#32927=DIRECTION('',(0.,1.,0.));
#32928=DIRECTION('center_axis',(0.415626937777453,0.707106781186548,0.572061402817684));
#32929=DIRECTION('ref_axis',(0.415626937777453,-0.707106781186547,0.572061402817684));
#32930=DIRECTION('center_axis',(0.,1.,0.));
#32931=DIRECTION('ref_axis',(1.,0.,0.));
#32932=DIRECTION('center_axis',(-0.28760623847595,0.707106781186549,-0.64597418802125));
#32933=DIRECTION('ref_axis',(0.287606238475951,0.707106781186546,0.645974188021252));
#32934=DIRECTION('',(0.,-1.,0.));
#32935=DIRECTION('center_axis',(0.,-1.,0.));
#32936=DIRECTION('ref_axis',(0.,0.,1.));
#32937=DIRECTION('',(0.,1.,0.));
#32938=DIRECTION('center_axis',(0.287606238475948,0.707106781186554,0.645974188021245));
#32939=DIRECTION('ref_axis',(0.287606238475953,-0.707106781186541,0.645974188021257));
#32940=DIRECTION('center_axis',(0.,1.,0.));
#32941=DIRECTION('ref_axis',(1.,0.,0.));
#32942=DIRECTION('center_axis',(-0.147015766465198,0.707106781186547,-0.691654801480227));
#32943=DIRECTION('ref_axis',(0.147015766465198,0.707106781186548,0.691654801480225));
#32944=DIRECTION('',(0.,-1.,0.));
#32945=DIRECTION('center_axis',(0.,-1.,0.));
#32946=DIRECTION('ref_axis',(0.,0.,1.));
#32947=DIRECTION('',(0.,1.,0.));
#32948=DIRECTION('center_axis',(0.147015766465198,0.707106781186547,0.691654801480226));
#32949=DIRECTION('ref_axis',(0.147015766465198,-0.707106781186548,0.691654801480225));
#32950=DIRECTION('center_axis',(0.,1.,0.));
#32951=DIRECTION('ref_axis',(1.,0.,0.));
#32952=DIRECTION('center_axis',(8.65956056235494E-17,0.707106781186547,
-0.707106781186548));
#32953=DIRECTION('ref_axis',(0.,0.707106781186548,0.707106781186547));
#32954=DIRECTION('',(0.,-1.,0.));
#32955=DIRECTION('center_axis',(0.,-1.,0.));
#32956=DIRECTION('ref_axis',(0.,0.,1.));
#32957=DIRECTION('',(0.,1.,0.));
#32958=DIRECTION('center_axis',(-8.65956056235494E-17,0.707106781186547,
0.707106781186548));
#32959=DIRECTION('ref_axis',(0.,-0.707106781186548,0.707106781186547));
#32960=DIRECTION('center_axis',(0.,1.,0.));
#32961=DIRECTION('ref_axis',(1.,0.,0.));
#32962=DIRECTION('center_axis',(0.147015766465199,0.707106781186547,-0.691654801480226));
#32963=DIRECTION('ref_axis',(-0.147015766465199,0.707106781186548,0.691654801480225));
#32964=DIRECTION('',(0.,-1.,0.));
#32965=DIRECTION('center_axis',(0.,-1.,0.));
#32966=DIRECTION('ref_axis',(0.,0.,1.));
#32967=DIRECTION('',(0.,1.,0.));
#32968=DIRECTION('center_axis',(-0.147015766465199,0.707106781186549,0.691654801480225));
#32969=DIRECTION('ref_axis',(-0.147015766465199,-0.707106781186547,0.691654801480227));
#32970=DIRECTION('center_axis',(0.,1.,0.));
#32971=DIRECTION('ref_axis',(1.,0.,0.));
#32972=DIRECTION('center_axis',(0.287606238475951,0.707106781186546,-0.645974188021252));
#32973=DIRECTION('ref_axis',(-0.28760623847595,0.707106781186549,0.64597418802125));
#32974=DIRECTION('',(0.,-1.,0.));
#32975=DIRECTION('center_axis',(0.,-1.,0.));
#32976=DIRECTION('ref_axis',(0.,0.,1.));
#32977=DIRECTION('',(0.,1.,0.));
#32978=DIRECTION('center_axis',(-0.287606238475952,0.707106781186545,0.645974188021253));
#32979=DIRECTION('ref_axis',(-0.28760623847595,-0.70710678118655,0.645974188021249));
#32980=DIRECTION('center_axis',(0.,1.,0.));
#32981=DIRECTION('ref_axis',(1.,0.,0.));
#32982=DIRECTION('center_axis',(0.415626937777453,0.707106781186548,-0.572061402817684));
#32983=DIRECTION('ref_axis',(-0.415626937777454,0.707106781186547,0.572061402817684));
#32984=DIRECTION('',(0.,-1.,0.));
#32985=DIRECTION('center_axis',(0.,-1.,0.));
#32986=DIRECTION('ref_axis',(0.,0.,1.));
#32987=DIRECTION('',(0.,1.,0.));
#32988=DIRECTION('center_axis',(-0.415626937777449,0.707106781186555,0.572061402817678));
#32989=DIRECTION('ref_axis',(-0.415626937777458,-0.70710678118654,0.57206140281769));
#32990=DIRECTION('center_axis',(0.,1.,0.));
#32991=DIRECTION('ref_axis',(1.,0.,0.));
#32992=DIRECTION('center_axis',(0.525482745498762,0.707106781186544,-0.473146789255817));
#32993=DIRECTION('ref_axis',(-0.525482745498757,0.707106781186551,0.473146789255813));
#32994=DIRECTION('',(0.,-1.,0.));
#32995=DIRECTION('center_axis',(0.,-1.,0.));
#32996=DIRECTION('ref_axis',(0.,0.,1.));
#32997=DIRECTION('',(0.,1.,0.));
#32998=DIRECTION('center_axis',(-0.525482745498759,0.707106781186547,0.473146789255815));
#32999=DIRECTION('ref_axis',(-0.525482745498759,-0.707106781186548,0.473146789255814));
#33000=DIRECTION('center_axis',(0.,1.,0.));
#33001=DIRECTION('ref_axis',(1.,0.,0.));
#33002=DIRECTION('center_axis',(0.612372435695796,0.707106781186546,-0.353553390593274));
#33003=DIRECTION('ref_axis',(-0.612372435695793,0.707106781186549,0.353553390593273));
#33004=DIRECTION('',(0.,-1.,0.));
#33005=DIRECTION('center_axis',(0.,-1.,0.));
#33006=DIRECTION('ref_axis',(0.,0.,1.));
#33007=DIRECTION('center_axis',(0.672498511963959,0.707106781186546,-0.218508012224411));
#33008=DIRECTION('ref_axis',(-0.309016994374947,0.,-0.951056516295154));
#33009=DIRECTION('',(-0.309016994374947,0.,-0.951056516295154));
#33010=DIRECTION('',(0.309016994374947,0.,0.951056516295154));
#33011=DIRECTION('',(0.370681690811013,-0.577350269189625,-0.727503780584098));
#33012=DIRECTION('center_axis',(-0.218508012224414,0.707106781186536,-0.672498511963968));
#33013=DIRECTION('ref_axis',(-0.951056516295154,0.,0.309016994374947));
#33014=DIRECTION('',(0.951056516295154,0.,-0.309016994374947));
#33015=DIRECTION('',(-0.727503780584107,-0.57735026918963,-0.37068169081099));
#33016=DIRECTION('',(-0.951056516295154,0.,0.309016994374947));
#33017=DIRECTION('center_axis',(-0.672498511963953,0.707106781186552,0.218508012224409));
#33018=DIRECTION('ref_axis',(0.309016994374947,0.,0.951056516295154));
#33019=DIRECTION('',(-0.309016994374947,0.,-0.951056516295154));
#33020=DIRECTION('',(0.309016994374947,0.,0.951056516295154));
#33021=DIRECTION('center_axis',(-0.951056516295154,0.,0.309016994374947));
#33022=DIRECTION('ref_axis',(-0.309016994374947,0.,-0.951056516295154));
#33023=DIRECTION('',(0.,-1.,0.));
#33024=DIRECTION('',(-0.309016994374947,0.,-0.951056516295154));
#33025=DIRECTION('center_axis',(0.309016994374947,0.,0.951056516295154));
#33026=DIRECTION('ref_axis',(-0.951056516295154,0.,0.309016994374947));
#33027=DIRECTION('',(0.,-1.,0.));
#33028=DIRECTION('',(-0.951056516295154,0.,0.309016994374947));
#33029=DIRECTION('center_axis',(0.951056516295154,0.,-0.309016994374947));
#33030=DIRECTION('ref_axis',(0.309016994374947,0.,0.951056516295154));
#33031=DIRECTION('',(0.309016994374947,0.,0.951056516295154));
#33032=DIRECTION('center_axis',(0.703233176253404,0.707106781186548,-0.0739127852035666));
#33033=DIRECTION('ref_axis',(-0.104528463267653,0.,-0.994521895368273));
#33034=DIRECTION('',(-0.104528463267653,0.,-0.994521895368273));
#33035=DIRECTION('',(0.104528463267653,0.,0.994521895368273));
#33036=DIRECTION('',(0.513837947600291,-0.577350269189624,-0.634537020411409));
#33037=DIRECTION('center_axis',(-0.0739127852035671,0.707106781186543,-0.703233176253409));
#33038=DIRECTION('ref_axis',(-0.994521895368273,0.,0.104528463267653));
#33039=DIRECTION('',(0.994521895368273,0.,-0.104528463267653));
#33040=DIRECTION('',(-0.634537020411409,-0.577350269189628,-0.513837947600288));
#33041=DIRECTION('',(-0.994521895368273,0.,0.104528463267653));
#33042=DIRECTION('center_axis',(-0.703233176253404,0.707106781186547,0.0739127852035666));
#33043=DIRECTION('ref_axis',(0.104528463267653,0.,0.994521895368273));
#33044=DIRECTION('',(-0.104528463267653,0.,-0.994521895368273));
#33045=DIRECTION('',(0.104528463267653,0.,0.994521895368273));
#33046=DIRECTION('center_axis',(-0.994521895368273,0.,0.104528463267653));
#33047=DIRECTION('ref_axis',(-0.104528463267653,0.,-0.994521895368273));
#33048=DIRECTION('',(0.,-1.,0.));
#33049=DIRECTION('',(-0.104528463267653,0.,-0.994521895368273));
#33050=DIRECTION('center_axis',(0.104528463267653,0.,0.994521895368273));
#33051=DIRECTION('ref_axis',(-0.994521895368273,0.,0.104528463267653));
#33052=DIRECTION('',(0.,-1.,0.));
#33053=DIRECTION('',(-0.994521895368273,0.,0.104528463267653));
#33054=DIRECTION('center_axis',(0.994521895368273,0.,-0.104528463267653));
#33055=DIRECTION('ref_axis',(0.104528463267653,0.,0.994521895368273));
#33056=DIRECTION('',(0.104528463267653,0.,0.994521895368273));
#33057=DIRECTION('center_axis',(0.703233176253406,0.707106781186546,0.073912785203567));
#33058=DIRECTION('ref_axis',(0.104528463267654,0.,-0.994521895368273));
#33059=DIRECTION('',(0.104528463267654,0.,-0.994521895368273));
#33060=DIRECTION('',(-0.104528463267654,0.,0.994521895368273));
#33061=DIRECTION('',(0.634537020411404,-0.577350269189624,-0.513837947600297));
#33062=DIRECTION('center_axis',(0.0739127852035657,0.707106781186559,-0.703233176253393));
#33063=DIRECTION('ref_axis',(-0.994521895368273,0.,-0.104528463267654));
#33064=DIRECTION('',(0.994521895368273,0.,0.104528463267654));
#33065=DIRECTION('',(-0.513837947600281,-0.577350269189616,-0.634537020411425));
#33066=DIRECTION('',(-0.994521895368273,0.,-0.104528463267654));
#33067=DIRECTION('center_axis',(-0.703233176253405,0.707106781186547,-0.0739127852035669));
#33068=DIRECTION('ref_axis',(-0.104528463267654,0.,0.994521895368273));
#33069=DIRECTION('',(0.104528463267654,0.,-0.994521895368273));
#33070=DIRECTION('',(-0.104528463267654,0.,0.994521895368273));
#33071=DIRECTION('center_axis',(-0.994521895368273,0.,-0.104528463267654));
#33072=DIRECTION('ref_axis',(0.104528463267654,0.,-0.994521895368273));
#33073=DIRECTION('',(0.,-1.,0.));
#33074=DIRECTION('',(0.104528463267654,0.,-0.994521895368273));
#33075=DIRECTION('center_axis',(-0.104528463267654,0.,0.994521895368273));
#33076=DIRECTION('ref_axis',(-0.994521895368273,0.,-0.104528463267654));
#33077=DIRECTION('',(0.,-1.,0.));
#33078=DIRECTION('',(-0.994521895368273,0.,-0.104528463267654));
#33079=DIRECTION('center_axis',(0.994521895368273,0.,0.104528463267654));
#33080=DIRECTION('ref_axis',(-0.104528463267654,0.,0.994521895368273));
#33081=DIRECTION('',(-0.104528463267654,0.,0.994521895368273));
#33082=DIRECTION('center_axis',(0.672498511963959,0.707106781186546,0.218508012224411));
#33083=DIRECTION('ref_axis',(0.309016994374947,0.,-0.951056516295153));
#33084=DIRECTION('',(0.309016994374948,0.,-0.951056516295154));
#33085=DIRECTION('',(-0.309016994374948,0.,0.951056516295154));
#33086=DIRECTION('',(0.727503780584104,-0.577350269189638,-0.370681690810982));
#33087=DIRECTION('center_axis',(0.218508012224414,0.707106781186536,-0.672498511963969));
#33088=DIRECTION('ref_axis',(-0.951056516295153,0.,-0.309016994374947));
#33089=DIRECTION('',(0.951056516295153,0.,0.309016994374947));
#33090=DIRECTION('',(0.370681690811026,0.577350269189629,0.727503780584088));
#33091=DIRECTION('',(-0.951056516295154,0.,-0.309016994374948));
#33092=DIRECTION('center_axis',(-0.951056516295154,0.,-0.309016994374948));
#33093=DIRECTION('ref_axis',(0.309016994374948,0.,-0.951056516295154));
#33094=DIRECTION('',(0.,-1.,0.));
#33095=DIRECTION('',(0.309016994374948,0.,-0.951056516295154));
#33096=DIRECTION('center_axis',(-0.309016994374948,0.,0.951056516295154));
#33097=DIRECTION('ref_axis',(-0.951056516295154,0.,-0.309016994374948));
#33098=DIRECTION('',(0.,-1.,0.));
#33099=DIRECTION('',(-0.951056516295154,0.,-0.309016994374948));
#33100=DIRECTION('center_axis',(-0.672498511963952,0.707106781186553,-0.218508012224409));
#33101=DIRECTION('ref_axis',(-0.309016994374948,0.,0.951056516295154));
#33102=DIRECTION('',(-0.309016994374948,0.,0.951056516295154));
#33103=DIRECTION('',(0.309016994374948,0.,-0.951056516295154));
#33104=DIRECTION('center_axis',(0.,1.,0.));
#33105=DIRECTION('ref_axis',(0.,0.,1.));
#33106=DIRECTION('',(0.866025403784439,0.,-0.5));
#33107=DIRECTION('',(0.5,0.,0.866025403784439));
#33108=DIRECTION('',(-0.669130606358858,0.,-0.743144825477394));
#33109=DIRECTION('',(0.743144825477394,0.,-0.669130606358858));
#33110=DIRECTION('',(0.669130606358858,0.,0.743144825477394));
#33111=DIRECTION('',(-0.809016994374947,0.,-0.587785252292473));
#33112=DIRECTION('',(0.587785252292473,0.,-0.809016994374947));
#33113=DIRECTION('',(0.809016994374947,0.,0.587785252292473));
#33114=DIRECTION('',(-0.913545457642601,0.,-0.4067366430758));
#33115=DIRECTION('',(0.4067366430758,0.,-0.913545457642601));
#33116=DIRECTION('',(0.913545457642601,0.,0.4067366430758));
#33117=DIRECTION('',(-0.978147600733805,0.,-0.20791169081776));
#33118=DIRECTION('',(0.20791169081776,0.,-0.978147600733805));
#33119=DIRECTION('',(0.978147600733805,0.,0.20791169081776));
#33120=DIRECTION('',(-1.,0.,-1.22464679914735E-16));
#33121=DIRECTION('',(1.22464679914735E-16,0.,-1.));
#33122=DIRECTION('',(1.,0.,1.22464679914735E-16));
#33123=DIRECTION('',(-0.978147600733806,0.,0.207911690817759));
#33124=DIRECTION('',(-0.207911690817759,0.,-0.978147600733806));
#33125=DIRECTION('',(0.978147600733806,0.,-0.207911690817759));
#33126=DIRECTION('',(-0.913545457642601,0.,0.4067366430758));
#33127=DIRECTION('',(-0.4067366430758,0.,-0.913545457642601));
#33128=DIRECTION('',(0.913545457642601,0.,-0.4067366430758));
#33129=DIRECTION('',(-0.809016994374947,0.,0.587785252292473));
#33130=DIRECTION('',(-0.587785252292473,0.,-0.809016994374947));
#33131=DIRECTION('',(0.809016994374947,0.,-0.587785252292473));
#33132=DIRECTION('',(-0.669130606358858,0.,0.743144825477394));
#33133=DIRECTION('',(-0.743144825477394,0.,-0.669130606358858));
#33134=DIRECTION('',(0.669130606358858,0.,-0.743144825477394));
#33135=DIRECTION('',(-0.5,0.,0.866025403784438));
#33136=DIRECTION('',(-0.866025403784438,0.,-0.5));
#33137=DIRECTION('',(0.5,0.,-0.866025403784438));
#33138=DIRECTION('',(-0.309016994374948,0.,0.951056516295153));
#33139=DIRECTION('',(-0.951056516295153,0.,-0.309016994374948));
#33140=DIRECTION('',(0.309016994374948,0.,-0.951056516295153));
#33141=DIRECTION('',(-0.104528463267654,0.,0.994521895368273));
#33142=DIRECTION('',(-0.994521895368273,0.,-0.104528463267654));
#33143=DIRECTION('',(0.104528463267654,0.,-0.994521895368273));
#33144=DIRECTION('',(0.104528463267653,0.,0.994521895368273));
#33145=DIRECTION('',(-0.994521895368273,0.,0.104528463267653));
#33146=DIRECTION('',(-0.104528463267653,0.,-0.994521895368273));
#33147=DIRECTION('',(0.309016994374947,0.,0.951056516295154));
#33148=DIRECTION('',(-0.951056516295154,0.,0.309016994374947));
#33149=DIRECTION('',(-0.309016994374947,0.,-0.951056516295154));
#33150=DIRECTION('',(0.499999999999999,0.,0.866025403784439));
#33151=DIRECTION('',(-0.866025403784439,0.,0.499999999999999));
#33152=DIRECTION('',(-0.499999999999999,0.,-0.866025403784439));
#33153=DIRECTION('',(0.669130606358858,0.,0.743144825477395));
#33154=DIRECTION('',(-0.743144825477395,0.,0.669130606358858));
#33155=DIRECTION('',(-0.669130606358858,0.,-0.743144825477395));
#33156=DIRECTION('',(0.809016994374947,0.,0.587785252292473));
#33157=DIRECTION('',(-0.587785252292473,0.,0.809016994374947));
#33158=DIRECTION('',(-0.809016994374947,0.,-0.587785252292473));
#33159=DIRECTION('',(0.913545457642601,0.,0.406736643075801));
#33160=DIRECTION('',(-0.406736643075801,0.,0.913545457642601));
#33161=DIRECTION('',(-0.913545457642601,0.,-0.406736643075801));
#33162=DIRECTION('',(0.978147600733805,0.,0.20791169081776));
#33163=DIRECTION('',(-0.20791169081776,0.,0.978147600733805));
#33164=DIRECTION('',(-0.978147600733805,0.,-0.20791169081776));
#33165=DIRECTION('',(1.,0.,0.));
#33166=DIRECTION('',(0.,0.,1.));
#33167=DIRECTION('',(-1.,0.,0.));
#33168=DIRECTION('',(0.978147600733806,0.,-0.207911690817759));
#33169=DIRECTION('',(0.207911690817759,0.,0.978147600733806));
#33170=DIRECTION('',(-0.978147600733806,0.,0.207911690817759));
#33171=DIRECTION('',(0.913545457642601,0.,-0.4067366430758));
#33172=DIRECTION('',(0.4067366430758,0.,0.913545457642601));
#33173=DIRECTION('',(-0.913545457642601,0.,0.4067366430758));
#33174=DIRECTION('',(0.809016994374947,0.,-0.587785252292473));
#33175=DIRECTION('',(0.587785252292473,0.,0.809016994374947));
#33176=DIRECTION('',(-0.809016994374947,0.,0.587785252292473));
#33177=DIRECTION('',(0.669130606358858,0.,-0.743144825477394));
#33178=DIRECTION('',(0.743144825477394,0.,0.669130606358858));
#33179=DIRECTION('',(-0.669130606358858,0.,0.743144825477394));
#33180=DIRECTION('',(0.5,0.,-0.866025403784439));
#33181=DIRECTION('',(0.866025403784439,0.,0.5));
#33182=DIRECTION('',(-0.5,0.,0.866025403784439));
#33183=DIRECTION('',(-1.,0.,0.));
#33184=DIRECTION('center_axis',(0.,1.,0.));
#33185=DIRECTION('ref_axis',(1.,0.,0.));
#33186=DIRECTION('',(-1.,0.,0.));
#33187=DIRECTION('',(0.,0.,-1.));
#33188=DIRECTION('',(1.,0.,0.));
#33189=DIRECTION('center_axis',(0.,1.,0.));
#33190=DIRECTION('ref_axis',(1.,0.,0.));
#33191=DIRECTION('',(1.,0.,0.));
#33192=DIRECTION('',(0.,0.,1.));
#33193=DIRECTION('center_axis',(0.612372435695797,0.707106781186544,0.353553390593275));
#33194=DIRECTION('ref_axis',(0.5,0.,-0.866025403784439));
#33195=DIRECTION('',(0.5,0.,-0.866025403784439));
#33196=DIRECTION('',(0.788675134594807,-0.577350269189639,-0.211324865405175));
#33197=DIRECTION('center_axis',(0.353553390593278,0.70710678118654,-0.612372435695801));
#33198=DIRECTION('ref_axis',(-0.866025403784439,0.,-0.5));
#33199=DIRECTION('',(-0.211324865405192,-0.577350269189633,-0.788675134594806));
#33200=DIRECTION('',(-0.866025403784439,0.,-0.5));
#33201=DIRECTION('center_axis',(-0.612372435695796,0.707106781186545,-0.353553390593275));
#33202=DIRECTION('ref_axis',(-0.5,0.,0.866025403784439));
#33203=DIRECTION('',(-0.5,0.,0.866025403784439));
#33204=DIRECTION('center_axis',(0.525482745498763,0.707106781186542,0.473146789255819));
#33205=DIRECTION('ref_axis',(0.669130606358858,0.,-0.743144825477394));
#33206=DIRECTION('',(0.669130606358858,0.,-0.743144825477394));
#33207=DIRECTION('',(0.815377600740549,-0.577350269189636,-0.0427321293319401));
#33208=DIRECTION('center_axis',(0.473146789255821,0.707106781186539,-0.525482745498766));
#33209=DIRECTION('ref_axis',(-0.743144825477394,0.,-0.669130606358858));
#33210=DIRECTION('',(-0.0427321293319529,-0.577350269189635,-0.815377600740548));
#33211=DIRECTION('',(-0.743144825477394,0.,-0.669130606358858));
#33212=DIRECTION('center_axis',(-0.525482745498759,0.707106781186547,-0.473146789255815));
#33213=DIRECTION('ref_axis',(-0.669130606358858,0.,0.743144825477394));
#33214=DIRECTION('',(-0.669130606358858,0.,0.743144825477394));
#33215=DIRECTION('center_axis',(0.415626937777452,0.707106781186551,0.572061402817682));
#33216=DIRECTION('ref_axis',(0.809016994374947,0.,-0.587785252292473));
#33217=DIRECTION('',(0.809016994374947,0.,-0.587785252292473));
#33218=DIRECTION('',(0.806444153118105,-0.577350269189629,0.127728205844619));
#33219=DIRECTION('center_axis',(0.572061402817692,0.707106781186538,-0.415626937777459));
#33220=DIRECTION('ref_axis',(-0.587785252292473,0.,-0.809016994374947));
#33221=DIRECTION('',(0.127728205844585,-0.577350269189623,-0.806444153118115));
#33222=DIRECTION('',(-0.587785252292473,0.,-0.809016994374947));
#33223=DIRECTION('center_axis',(-0.41562693777745,0.707106781186553,-0.57206140281768));
#33224=DIRECTION('ref_axis',(-0.809016994374947,0.,0.587785252292473));
#33225=DIRECTION('',(-0.809016994374947,0.,0.587785252292473));
#33226=DIRECTION('center_axis',(0.28760623847595,0.707106781186549,0.64597418802125));
#33227=DIRECTION('ref_axis',(0.913545457642601,0.,-0.4067366430758));
#33228=DIRECTION('',(0.913545457642601,0.,-0.4067366430758));
#33229=DIRECTION('',(0.76226522625601,-0.577350269189626,0.292606205517827));
#33230=DIRECTION('center_axis',(0.645974188021254,0.707106781186545,-0.287606238475952));
#33231=DIRECTION('ref_axis',(-0.4067366430758,0.,-0.913545457642601));
#33232=DIRECTION('',(0.292606205517814,-0.577350269189627,-0.762265226256014));
#33233=DIRECTION('',(-0.4067366430758,0.,-0.913545457642601));
#33234=DIRECTION('center_axis',(-0.28760623847595,0.707106781186549,-0.64597418802125));
#33235=DIRECTION('ref_axis',(-0.913545457642601,0.,0.4067366430758));
#33236=DIRECTION('',(-0.913545457642601,0.,0.4067366430758));
#33237=DIRECTION('center_axis',(0.147015766465199,0.707106781186544,0.691654801480229));
#33238=DIRECTION('ref_axis',(0.978147600733806,0.,-0.207911690817759));
#33239=DIRECTION('',(0.978147600733806,0.,-0.207911690817759));
#33240=DIRECTION('',(0.68477165125216,-0.577350269189626,0.444695909929535));
#33241=DIRECTION('center_axis',(0.691654801480227,0.707106781186546,-0.147015766465199));
#33242=DIRECTION('ref_axis',(-0.207911690817759,0.,-0.978147600733806));
#33243=DIRECTION('',(0.444695909929538,-0.57735026918963,-0.684771651252155));
#33244=DIRECTION('',(-0.207911690817759,0.,-0.978147600733806));
#33245=DIRECTION('center_axis',(-0.147015766465199,0.707106781186546,-0.691654801480227));
#33246=DIRECTION('ref_axis',(-0.978147600733806,0.,0.207911690817759));
#33247=DIRECTION('',(-0.978147600733806,0.,0.207911690817759));
#33248=DIRECTION('center_axis',(0.,0.707106781186547,0.707106781186548));
#33249=DIRECTION('ref_axis',(1.,0.,0.));
#33250=DIRECTION('',(1.,0.,0.));
#33251=DIRECTION('',(0.577350269189627,-0.577350269189627,0.577350269189624));
#33252=DIRECTION('center_axis',(0.707106781186548,0.707106781186548,0.));
#33253=DIRECTION('ref_axis',(0.,0.,-1.));
#33254=DIRECTION('',(0.577350269189626,-0.577350269189626,-0.577350269189625));
#33255=DIRECTION('',(0.,0.,-1.));
#33256=DIRECTION('center_axis',(0.,0.707106781186547,-0.707106781186548));
#33257=DIRECTION('ref_axis',(-1.,0.,0.));
#33258=DIRECTION('',(-1.,0.,0.));
#33259=DIRECTION('center_axis',(-0.353553390593273,0.707106781186549,-0.612372435695794));
#33260=DIRECTION('ref_axis',(-0.866025403784439,0.,0.5));
#33261=DIRECTION('',(-0.866025403784439,0.,0.5));
#33262=DIRECTION('',(0.211324865405184,-0.577350269189626,-0.788675134594813));
#33263=DIRECTION('center_axis',(0.5,0.,0.866025403784439));
#33264=DIRECTION('ref_axis',(-0.866025403784439,0.,0.5));
#33265=DIRECTION('',(-0.866025403784439,0.,0.5));
#33266=DIRECTION('',(0.,-1.,0.));
#33267=DIRECTION('center_axis',(0.612372435695796,0.707106781186546,-0.353553390593274));
#33268=DIRECTION('ref_axis',(-0.5,0.,-0.866025403784439));
#33269=DIRECTION('',(-0.5,0.,-0.866025403784439));
#33270=DIRECTION('center_axis',(0.525482745498762,0.707106781186544,-0.473146789255817));
#33271=DIRECTION('ref_axis',(-0.669130606358858,0.,-0.743144825477394));
#33272=DIRECTION('',(-0.669130606358858,0.,-0.743144825477394));
#33273=DIRECTION('',(0.0427321293319396,-0.57735026918963,-0.815377600740553));
#33274=DIRECTION('center_axis',(-0.473146789255815,0.707106781186547,-0.525482745498759));
#33275=DIRECTION('ref_axis',(-0.743144825477394,0.,0.669130606358858));
#33276=DIRECTION('',(-0.743144825477394,0.,0.669130606358858));
#33277=DIRECTION('',(-0.815377600740555,-0.577350269189626,-0.0427321293319522));
#33278=DIRECTION('center_axis',(-0.525482745498759,0.707106781186547,0.473146789255815));
#33279=DIRECTION('ref_axis',(0.669130606358858,0.,0.743144825477394));
#33280=DIRECTION('',(0.669130606358858,0.,0.743144825477394));
#33281=DIRECTION('center_axis',(-0.743144825477394,0.,0.669130606358858));
#33282=DIRECTION('ref_axis',(-0.669130606358858,0.,-0.743144825477394));
#33283=DIRECTION('',(0.,-1.,0.));
#33284=DIRECTION('',(-0.669130606358858,0.,-0.743144825477394));
#33285=DIRECTION('center_axis',(0.669130606358858,0.,0.743144825477394));
#33286=DIRECTION('ref_axis',(-0.743144825477394,0.,0.669130606358858));
#33287=DIRECTION('',(0.,-1.,0.));
#33288=DIRECTION('',(-0.743144825477394,0.,0.669130606358858));
#33289=DIRECTION('center_axis',(0.743144825477394,0.,-0.669130606358858));
#33290=DIRECTION('ref_axis',(0.669130606358858,0.,0.743144825477394));
#33291=DIRECTION('',(0.669130606358858,0.,0.743144825477394));
#33292=DIRECTION('center_axis',(0.415626937777453,0.707106781186548,-0.572061402817684));
#33293=DIRECTION('ref_axis',(-0.809016994374947,0.,-0.587785252292473));
#33294=DIRECTION('',(-0.809016994374947,0.,-0.587785252292473));
#33295=DIRECTION('',(-0.127728205844611,-0.577350269189624,-0.80644415311811));
#33296=DIRECTION('center_axis',(-0.572061402817685,0.707106781186546,-0.415626937777454));
#33297=DIRECTION('ref_axis',(-0.587785252292473,0.,0.809016994374947));
#33298=DIRECTION('',(-0.587785252292473,0.,0.809016994374947));
#33299=DIRECTION('',(-0.80644415311811,-0.577350269189624,0.127728205844611));
#33300=DIRECTION('center_axis',(-0.415626937777449,0.707106781186555,0.572061402817678));
#33301=DIRECTION('ref_axis',(0.809016994374947,0.,0.587785252292473));
#33302=DIRECTION('',(0.809016994374947,0.,0.587785252292473));
#33303=DIRECTION('center_axis',(-0.587785252292473,0.,0.809016994374947));
#33304=DIRECTION('ref_axis',(-0.809016994374947,0.,-0.587785252292473));
#33305=DIRECTION('',(0.,-1.,0.));
#33306=DIRECTION('',(-0.809016994374947,0.,-0.587785252292473));
#33307=DIRECTION('center_axis',(0.809016994374947,0.,0.587785252292473));
#33308=DIRECTION('ref_axis',(-0.587785252292473,0.,0.809016994374947));
#33309=DIRECTION('',(0.,-1.,0.));
#33310=DIRECTION('',(-0.587785252292473,0.,0.809016994374947));
#33311=DIRECTION('center_axis',(0.587785252292473,0.,-0.809016994374947));
#33312=DIRECTION('ref_axis',(0.809016994374947,0.,0.587785252292473));
#33313=DIRECTION('',(0.809016994374947,0.,0.587785252292473));
#33314=DIRECTION('center_axis',(0.287606238475951,0.707106781186546,-0.645974188021252));
#33315=DIRECTION('ref_axis',(-0.913545457642601,0.,-0.4067366430758));
#33316=DIRECTION('',(-0.913545457642601,0.,-0.4067366430758));
#33317=DIRECTION('',(-0.292606205517816,-0.57735026918963,-0.762265226256011));
#33318=DIRECTION('center_axis',(-0.645974188021253,0.707106781186545,-0.287606238475952));
#33319=DIRECTION('ref_axis',(-0.4067366430758,0.,0.913545457642601));
#33320=DIRECTION('',(-0.4067366430758,0.,0.913545457642601));
#33321=DIRECTION('',(-0.762265226256014,-0.577350269189629,0.292606205517809));
#33322=DIRECTION('center_axis',(-0.287606238475952,0.707106781186545,0.645974188021253));
#33323=DIRECTION('ref_axis',(0.913545457642601,0.,0.4067366430758));
#33324=DIRECTION('',(0.913545457642601,0.,0.4067366430758));
#33325=DIRECTION('center_axis',(-0.4067366430758,0.,0.913545457642601));
#33326=DIRECTION('ref_axis',(-0.913545457642601,0.,-0.4067366430758));
#33327=DIRECTION('',(0.,-1.,0.));
#33328=DIRECTION('',(-0.913545457642601,0.,-0.4067366430758));
#33329=DIRECTION('center_axis',(0.913545457642601,0.,0.4067366430758));
#33330=DIRECTION('ref_axis',(-0.4067366430758,0.,0.913545457642601));
#33331=DIRECTION('',(0.,-1.,0.));
#33332=DIRECTION('',(-0.4067366430758,0.,0.913545457642601));
#33333=DIRECTION('center_axis',(0.4067366430758,0.,-0.913545457642601));
#33334=DIRECTION('ref_axis',(0.913545457642601,0.,0.4067366430758));
#33335=DIRECTION('',(0.913545457642601,0.,0.4067366430758));
#33336=DIRECTION('center_axis',(0.147015766465199,0.707106781186547,-0.691654801480226));
#33337=DIRECTION('ref_axis',(-0.978147600733805,0.,-0.20791169081776));
#33338=DIRECTION('',(-0.978147600733805,0.,-0.20791169081776));
#33339=DIRECTION('',(-0.444695909929548,-0.577350269189626,-0.684771651252151));
#33340=DIRECTION('center_axis',(-0.691654801480235,0.707106781186538,-0.147015766465201));
#33341=DIRECTION('ref_axis',(-0.20791169081776,0.,0.978147600733805));
#33342=DIRECTION('',(-0.20791169081776,0.,0.978147600733805));
#33343=DIRECTION('',(-0.684771651252149,-0.577350269189628,0.444695909929549));
#33344=DIRECTION('center_axis',(-0.147015766465199,0.707106781186549,0.691654801480225));
#33345=DIRECTION('ref_axis',(0.978147600733805,0.,0.20791169081776));
#33346=DIRECTION('',(0.978147600733805,0.,0.20791169081776));
#33347=DIRECTION('center_axis',(-0.20791169081776,0.,0.978147600733806));
#33348=DIRECTION('ref_axis',(-0.978147600733805,0.,-0.20791169081776));
#33349=DIRECTION('',(0.,-1.,0.));
#33350=DIRECTION('',(-0.978147600733805,0.,-0.20791169081776));
#33351=DIRECTION('center_axis',(0.978147600733806,0.,0.20791169081776));
#33352=DIRECTION('ref_axis',(-0.20791169081776,0.,0.978147600733805));
#33353=DIRECTION('',(0.,-1.,0.));
#33354=DIRECTION('',(-0.20791169081776,0.,0.978147600733805));
#33355=DIRECTION('center_axis',(0.20791169081776,0.,-0.978147600733806));
#33356=DIRECTION('ref_axis',(0.978147600733805,0.,0.20791169081776));
#33357=DIRECTION('',(0.978147600733805,0.,0.20791169081776));
#33358=DIRECTION('center_axis',(8.65956056235494E-17,0.707106781186547,
-0.707106781186548));
#33359=DIRECTION('ref_axis',(-1.,0.,-1.22464679914735E-16));
#33360=DIRECTION('',(-1.,0.,-1.22464679914735E-16));
#33361=DIRECTION('',(-0.577350269189626,-0.577350269189626,-0.577350269189625));
#33362=DIRECTION('center_axis',(-0.707106781186548,0.707106781186548,-8.65956056235493E-17));
#33363=DIRECTION('ref_axis',(-1.22464679914735E-16,0.,1.));
#33364=DIRECTION('',(-1.22464679914735E-16,0.,1.));
#33365=DIRECTION('',(-0.577350269189626,-0.577350269189626,0.577350269189625));
#33366=DIRECTION('center_axis',(-8.65956056235494E-17,0.707106781186547,
0.707106781186548));
#33367=DIRECTION('ref_axis',(1.,0.,1.22464679914735E-16));
#33368=DIRECTION('',(1.,0.,1.22464679914735E-16));
#33369=DIRECTION('center_axis',(-1.22464679914735E-16,0.,1.));
#33370=DIRECTION('ref_axis',(-1.,0.,-1.22464679914735E-16));
#33371=DIRECTION('',(0.,-1.,0.));
#33372=DIRECTION('',(-1.,0.,-1.22464679914735E-16));
#33373=DIRECTION('center_axis',(1.,0.,1.22464679914735E-16));
#33374=DIRECTION('ref_axis',(-1.22464679914735E-16,0.,1.));
#33375=DIRECTION('',(0.,-1.,0.));
#33376=DIRECTION('',(-1.22464679914735E-16,0.,1.));
#33377=DIRECTION('center_axis',(1.22464679914735E-16,0.,-1.));
#33378=DIRECTION('ref_axis',(1.,0.,1.22464679914735E-16));
#33379=DIRECTION('',(1.,0.,1.22464679914735E-16));
#33380=DIRECTION('center_axis',(-0.147015766465198,0.707106781186547,-0.691654801480227));
#33381=DIRECTION('ref_axis',(-0.978147600733806,0.,0.207911690817759));
#33382=DIRECTION('',(-0.978147600733806,0.,0.207911690817759));
#33383=DIRECTION('',(-0.684771651252158,-0.577350269189624,-0.44469590992954));
#33384=DIRECTION('center_axis',(-0.691654801480227,0.707106781186546,0.147015766465199));
#33385=DIRECTION('ref_axis',(0.207911690817759,0.,0.978147600733806));
#33386=DIRECTION('',(0.207911690817759,0.,0.978147600733806));
#33387=DIRECTION('',(-0.444695909929548,-0.577350269189626,0.684771651252151));
#33388=DIRECTION('center_axis',(0.147015766465198,0.707106781186547,0.691654801480226));
#33389=DIRECTION('ref_axis',(0.978147600733806,0.,-0.207911690817759));
#33390=DIRECTION('',(0.978147600733806,0.,-0.207911690817759));
#33391=DIRECTION('center_axis',(0.207911690817759,0.,0.978147600733806));
#33392=DIRECTION('ref_axis',(-0.978147600733806,0.,0.207911690817759));
#33393=DIRECTION('',(0.,-1.,0.));
#33394=DIRECTION('',(-0.978147600733806,0.,0.207911690817759));
#33395=DIRECTION('center_axis',(0.978147600733806,0.,-0.207911690817759));
#33396=DIRECTION('ref_axis',(0.207911690817759,0.,0.978147600733806));
#33397=DIRECTION('',(0.,-1.,0.));
#33398=DIRECTION('',(0.207911690817759,0.,0.978147600733806));
#33399=DIRECTION('center_axis',(-0.207911690817759,0.,-0.978147600733806));
#33400=DIRECTION('ref_axis',(0.978147600733806,0.,-0.207911690817759));
#33401=DIRECTION('',(0.978147600733806,0.,-0.207911690817759));
#33402=DIRECTION('center_axis',(0.287606238475948,0.707106781186554,0.645974188021245));
#33403=DIRECTION('ref_axis',(0.913545457642601,0.,-0.4067366430758));
#33404=DIRECTION('',(0.913545457642601,0.,-0.4067366430758));
#33405=DIRECTION('',(-0.292606205517798,-0.577350269189628,0.762265226256019));
#33406=DIRECTION('center_axis',(-0.4067366430758,0.,-0.913545457642601));
#33407=DIRECTION('ref_axis',(0.913545457642601,0.,-0.4067366430758));
#33408=DIRECTION('',(0.913545457642601,0.,-0.4067366430758));
#33409=DIRECTION('',(0.,-1.,0.));
#33410=DIRECTION('center_axis',(-0.28760623847595,0.707106781186549,-0.64597418802125));
#33411=DIRECTION('ref_axis',(-0.913545457642601,0.,0.4067366430758));
#33412=DIRECTION('',(-0.913545457642601,0.,0.4067366430758));
#33413=DIRECTION('',(-0.762265226256003,-0.577350269189631,-0.292606205517836));
#33414=DIRECTION('center_axis',(-0.645974188021261,0.707106781186537,0.287606238475955));
#33415=DIRECTION('ref_axis',(0.4067366430758,0.,0.913545457642601));
#33416=DIRECTION('',(0.4067366430758,0.,0.913545457642601));
#33417=DIRECTION('center_axis',(0.4067366430758,0.,0.913545457642601));
#33418=DIRECTION('ref_axis',(-0.913545457642601,0.,0.4067366430758));
#33419=DIRECTION('',(0.,-1.,0.));
#33420=DIRECTION('',(-0.913545457642601,0.,0.4067366430758));
#33421=DIRECTION('center_axis',(0.913545457642601,0.,-0.4067366430758));
#33422=DIRECTION('ref_axis',(0.4067366430758,0.,0.913545457642601));
#33423=DIRECTION('',(0.4067366430758,0.,0.913545457642601));
#33424=DIRECTION('center_axis',(-0.415626937777449,0.707106781186555,-0.572061402817678));
#33425=DIRECTION('ref_axis',(-0.809016994374947,0.,0.587785252292473));
#33426=DIRECTION('',(-0.809016994374947,0.,0.587785252292473));
#33427=DIRECTION('',(-0.806444153118099,-0.577350269189634,-0.127728205844633));
#33428=DIRECTION('center_axis',(-0.572061402817694,0.707106781186535,0.415626937777461));
#33429=DIRECTION('ref_axis',(0.587785252292473,0.,0.809016994374947));
#33430=DIRECTION('',(0.587785252292473,0.,0.809016994374947));
#33431=DIRECTION('',(-0.127728205844587,-0.577350269189629,0.80644415311811));
#33432=DIRECTION('center_axis',(0.415626937777453,0.707106781186548,0.572061402817684));
#33433=DIRECTION('ref_axis',(0.809016994374947,0.,-0.587785252292473));
#33434=DIRECTION('',(0.809016994374947,0.,-0.587785252292473));
#33435=DIRECTION('center_axis',(0.587785252292473,0.,0.809016994374948));
#33436=DIRECTION('ref_axis',(-0.809016994374947,0.,0.587785252292473));
#33437=DIRECTION('',(0.,-1.,0.));
#33438=DIRECTION('',(-0.809016994374947,0.,0.587785252292473));
#33439=DIRECTION('center_axis',(0.809016994374948,0.,-0.587785252292473));
#33440=DIRECTION('ref_axis',(0.587785252292473,0.,0.809016994374947));
#33441=DIRECTION('',(0.,-1.,0.));
#33442=DIRECTION('',(0.587785252292473,0.,0.809016994374947));
#33443=DIRECTION('center_axis',(-0.587785252292473,0.,-0.809016994374948));
#33444=DIRECTION('ref_axis',(0.809016994374947,0.,-0.587785252292473));
#33445=DIRECTION('',(0.809016994374947,0.,-0.587785252292473));
#33446=DIRECTION('center_axis',(-0.525482745498762,0.707106781186543,-0.473146789255818));
#33447=DIRECTION('ref_axis',(-0.669130606358858,0.,0.743144825477394));
#33448=DIRECTION('',(-0.669130606358858,0.,0.743144825477394));
#33449=DIRECTION('',(-0.815377600740551,-0.577350269189633,0.0427321293319399));
#33450=DIRECTION('center_axis',(-0.473146789255817,0.707106781186545,0.525482745498761));
#33451=DIRECTION('ref_axis',(0.743144825477394,0.,0.669130606358858));
#33452=DIRECTION('',(0.743144825477394,0.,0.669130606358858));
#33453=DIRECTION('',(0.0427321293319399,-0.577350269189633,0.815377600740551));
#33454=DIRECTION('center_axis',(0.525482745498759,0.707106781186547,0.473146789255815));
#33455=DIRECTION('ref_axis',(0.669130606358858,0.,-0.743144825477394));
#33456=DIRECTION('',(0.669130606358858,0.,-0.743144825477394));
#33457=DIRECTION('center_axis',(0.743144825477394,0.,0.669130606358858));
#33458=DIRECTION('ref_axis',(-0.669130606358858,0.,0.743144825477394));
#33459=DIRECTION('',(0.,-1.,0.));
#33460=DIRECTION('',(-0.669130606358858,0.,0.743144825477394));
#33461=DIRECTION('center_axis',(0.669130606358858,0.,-0.743144825477394));
#33462=DIRECTION('ref_axis',(0.743144825477394,0.,0.669130606358858));
#33463=DIRECTION('',(0.,-1.,0.));
#33464=DIRECTION('',(0.743144825477394,0.,0.669130606358858));
#33465=DIRECTION('center_axis',(-0.743144825477394,0.,-0.669130606358858));
#33466=DIRECTION('ref_axis',(0.669130606358858,0.,-0.743144825477394));
#33467=DIRECTION('',(0.669130606358858,0.,-0.743144825477394));
#33468=DIRECTION('center_axis',(-0.612372435695796,0.707106781186545,-0.353553390593275));
#33469=DIRECTION('ref_axis',(-0.5,0.,0.866025403784438));
#33470=DIRECTION('',(-0.5,0.,0.866025403784438));
#33471=DIRECTION('',(-0.788675134594813,-0.577350269189619,0.211324865405206));
#33472=DIRECTION('center_axis',(-0.353553390593269,0.707106781186557,0.612372435695786));
#33473=DIRECTION('ref_axis',(0.866025403784438,0.,0.5));
#33474=DIRECTION('',(0.866025403784438,0.,0.5));
#33475=DIRECTION('',(0.211324865405179,-0.577350269189617,0.788675134594822));
#33476=DIRECTION('center_axis',(0.612372435695793,0.707106781186549,0.353553390593274));
#33477=DIRECTION('ref_axis',(0.5,0.,-0.866025403784438));
#33478=DIRECTION('',(0.5,0.,-0.866025403784438));
#33479=DIRECTION('center_axis',(0.866025403784438,0.,0.5));
#33480=DIRECTION('ref_axis',(-0.5,0.,0.866025403784438));
#33481=DIRECTION('',(0.,-1.,0.));
#33482=DIRECTION('',(-0.5,0.,0.866025403784438));
#33483=DIRECTION('center_axis',(0.5,0.,-0.866025403784438));
#33484=DIRECTION('ref_axis',(0.866025403784438,0.,0.5));
#33485=DIRECTION('',(0.,-1.,0.));
#33486=DIRECTION('',(0.866025403784438,0.,0.5));
#33487=DIRECTION('center_axis',(-0.866025403784438,0.,-0.5));
#33488=DIRECTION('ref_axis',(0.5,0.,-0.866025403784438));
#33489=DIRECTION('',(0.5,0.,-0.866025403784438));
#33490=DIRECTION('center_axis',(-0.672498511963957,0.707106781186548,-0.218508012224411));
#33491=DIRECTION('ref_axis',(-0.309016994374948,0.,0.951056516295153));
#33492=DIRECTION('',(-0.309016994374948,0.,0.951056516295153));
#33493=DIRECTION('',(-0.7275037805841,-0.577350269189624,0.370681690811012));
#33494=DIRECTION('center_axis',(-0.218508012224412,0.707106781186544,0.67249851196396));
#33495=DIRECTION('ref_axis',(0.951056516295153,0.,0.309016994374948));
#33496=DIRECTION('',(0.951056516295153,0.,0.309016994374948));
#33497=DIRECTION('',(0.370681690811018,-0.577350269189624,0.727503780584097));
#33498=DIRECTION('center_axis',(0.672498511963954,0.707106781186551,0.21850801222441));
#33499=DIRECTION('ref_axis',(0.309016994374948,0.,-0.951056516295153));
#33500=DIRECTION('',(0.309016994374948,0.,-0.951056516295153));
#33501=DIRECTION('center_axis',(0.951056516295154,0.,0.309016994374948));
#33502=DIRECTION('ref_axis',(-0.309016994374948,0.,0.951056516295153));
#33503=DIRECTION('',(0.,-1.,0.));
#33504=DIRECTION('',(-0.309016994374948,0.,0.951056516295153));
#33505=DIRECTION('center_axis',(0.309016994374948,0.,-0.951056516295154));
#33506=DIRECTION('ref_axis',(0.951056516295153,0.,0.309016994374948));
#33507=DIRECTION('',(0.,-1.,0.));
#33508=DIRECTION('',(0.951056516295153,0.,0.309016994374948));
#33509=DIRECTION('center_axis',(-0.951056516295154,0.,-0.309016994374948));
#33510=DIRECTION('ref_axis',(0.309016994374948,0.,-0.951056516295153));
#33511=DIRECTION('',(0.309016994374948,0.,-0.951056516295153));
#33512=DIRECTION('center_axis',(-0.703233176253405,0.707106781186547,-0.0739127852035674));
#33513=DIRECTION('ref_axis',(-0.104528463267654,0.,0.994521895368273));
#33514=DIRECTION('',(-0.104528463267654,0.,0.994521895368273));
#33515=DIRECTION('',(-0.634537020411399,-0.577350269189621,0.513837947600307));
#33516=DIRECTION('center_axis',(-0.0739127852035669,0.707106781186551,0.703233176253401));
#33517=DIRECTION('ref_axis',(0.994521895368273,0.,0.104528463267654));
#33518=DIRECTION('',(0.994521895368273,0.,0.104528463267654));
#33519=DIRECTION('',(0.513837947600289,-0.577350269189625,0.63453702041141));
#33520=DIRECTION('center_axis',(0.703233176253406,0.707106781186546,0.0739127852035675));
#33521=DIRECTION('ref_axis',(0.104528463267654,0.,-0.994521895368273));
#33522=DIRECTION('',(0.104528463267654,0.,-0.994521895368273));
#33523=DIRECTION('center_axis',(0.994521895368273,0.,0.104528463267654));
#33524=DIRECTION('ref_axis',(-0.104528463267654,0.,0.994521895368273));
#33525=DIRECTION('',(0.,-1.,0.));
#33526=DIRECTION('',(-0.104528463267654,0.,0.994521895368273));
#33527=DIRECTION('center_axis',(0.104528463267654,0.,-0.994521895368273));
#33528=DIRECTION('ref_axis',(0.994521895368273,0.,0.104528463267654));
#33529=DIRECTION('',(0.,-1.,0.));
#33530=DIRECTION('',(0.994521895368273,0.,0.104528463267654));
#33531=DIRECTION('center_axis',(-0.994521895368273,0.,-0.104528463267654));
#33532=DIRECTION('ref_axis',(0.104528463267654,0.,-0.994521895368273));
#33533=DIRECTION('',(0.104528463267654,0.,-0.994521895368273));
#33534=DIRECTION('center_axis',(-0.703233176253405,0.707106781186547,0.0739127852035665));
#33535=DIRECTION('ref_axis',(0.104528463267653,0.,0.994521895368274));
#33536=DIRECTION('',(0.104528463267653,0.,0.994521895368273));
#33537=DIRECTION('',(-0.513837947600287,-0.57735026918962,0.634537020411416));
#33538=DIRECTION('center_axis',(0.0739127852035652,0.707106781186559,0.703233176253393));
#33539=DIRECTION('ref_axis',(0.994521895368273,0.,-0.104528463267653));
#33540=DIRECTION('',(0.994521895368273,0.,-0.104528463267653));
#33541=DIRECTION('',(0.634537020411404,-0.577350269189624,0.513837947600297));
#33542=DIRECTION('center_axis',(0.703233176253404,0.707106781186547,-0.0739127852035664));
#33543=DIRECTION('ref_axis',(-0.104528463267653,0.,-0.994521895368274));
#33544=DIRECTION('',(-0.104528463267653,0.,-0.994521895368273));
#33545=DIRECTION('center_axis',(0.994521895368273,0.,-0.104528463267653));
#33546=DIRECTION('ref_axis',(0.104528463267653,0.,0.994521895368273));
#33547=DIRECTION('',(0.,-1.,0.));
#33548=DIRECTION('',(0.104528463267653,0.,0.994521895368273));
#33549=DIRECTION('center_axis',(-0.104528463267653,0.,-0.994521895368273));
#33550=DIRECTION('ref_axis',(0.994521895368273,0.,-0.104528463267653));
#33551=DIRECTION('',(0.,-1.,0.));
#33552=DIRECTION('',(0.994521895368273,0.,-0.104528463267653));
#33553=DIRECTION('center_axis',(-0.994521895368273,0.,0.104528463267653));
#33554=DIRECTION('ref_axis',(-0.104528463267653,0.,-0.994521895368273));
#33555=DIRECTION('',(-0.104528463267653,0.,-0.994521895368273));
#33556=DIRECTION('center_axis',(-0.672498511963955,0.70710678118655,0.21850801222441));
#33557=DIRECTION('ref_axis',(0.309016994374947,0.,0.951056516295154));
#33558=DIRECTION('',(0.309016994374947,0.,0.951056516295154));
#33559=DIRECTION('',(-0.370681690810995,-0.577350269189617,0.727503780584114));
#33560=DIRECTION('center_axis',(0.218508012224409,0.707106781186553,0.672498511963952));
#33561=DIRECTION('ref_axis',(0.951056516295154,0.,-0.309016994374947));
#33562=DIRECTION('',(0.951056516295154,0.,-0.309016994374947));
#33563=DIRECTION('',(0.727503780584098,-0.57735026918962,0.370681690811022));
#33564=DIRECTION('center_axis',(0.672498511963957,0.707106781186548,-0.21850801222441));
#33565=DIRECTION('ref_axis',(-0.309016994374947,0.,-0.951056516295154));
#33566=DIRECTION('',(-0.309016994374947,0.,-0.951056516295154));
#33567=DIRECTION('center_axis',(0.951056516295154,0.,-0.309016994374947));
#33568=DIRECTION('ref_axis',(0.309016994374947,0.,0.951056516295154));
#33569=DIRECTION('',(0.,-1.,0.));
#33570=DIRECTION('',(0.309016994374947,0.,0.951056516295154));
#33571=DIRECTION('center_axis',(-0.309016994374947,0.,-0.951056516295154));
#33572=DIRECTION('ref_axis',(0.951056516295154,0.,-0.309016994374947));
#33573=DIRECTION('',(0.,-1.,0.));
#33574=DIRECTION('',(0.951056516295154,0.,-0.309016994374947));
#33575=DIRECTION('center_axis',(-0.951056516295154,0.,0.309016994374947));
#33576=DIRECTION('ref_axis',(-0.309016994374947,0.,-0.951056516295154));
#33577=DIRECTION('',(-0.309016994374947,0.,-0.951056516295154));
#33578=DIRECTION('center_axis',(-0.612372435695797,0.707106781186545,0.353553390593274));
#33579=DIRECTION('ref_axis',(0.499999999999999,0.,0.866025403784439));
#33580=DIRECTION('',(0.499999999999999,0.,0.866025403784439));
#33581=DIRECTION('',(-0.211324865405175,-0.577350269189623,0.788675134594818));
#33582=DIRECTION('center_axis',(0.353553390593268,0.707106781186557,0.612372435695786));
#33583=DIRECTION('ref_axis',(0.866025403784439,0.,-0.499999999999999));
#33584=DIRECTION('',(0.866025403784439,0.,-0.499999999999999));
#33585=DIRECTION('',(0.788675134594813,-0.577350269189619,0.211324865405206));
#33586=DIRECTION('center_axis',(0.612372435695795,0.707106781186547,-0.353553390593274));
#33587=DIRECTION('ref_axis',(-0.499999999999999,0.,-0.866025403784439));
#33588=DIRECTION('',(-0.499999999999999,0.,-0.866025403784439));
#33589=DIRECTION('center_axis',(0.866025403784439,0.,-0.499999999999999));
#33590=DIRECTION('ref_axis',(0.499999999999999,0.,0.866025403784439));
#33591=DIRECTION('',(0.,-1.,0.));
#33592=DIRECTION('',(0.499999999999999,0.,0.866025403784439));
#33593=DIRECTION('center_axis',(-0.499999999999999,0.,-0.866025403784439));
#33594=DIRECTION('ref_axis',(0.866025403784439,0.,-0.499999999999999));
#33595=DIRECTION('',(0.,-1.,0.));
#33596=DIRECTION('',(0.866025403784439,0.,-0.499999999999999));
#33597=DIRECTION('center_axis',(-0.866025403784439,0.,0.499999999999999));
#33598=DIRECTION('ref_axis',(-0.499999999999999,0.,-0.866025403784439));
#33599=DIRECTION('',(-0.499999999999999,0.,-0.866025403784439));
#33600=DIRECTION('center_axis',(-0.525482745498764,0.707106781186541,0.473146789255819));
#33601=DIRECTION('ref_axis',(0.669130606358858,0.,0.743144825477395));
#33602=DIRECTION('',(0.669130606358858,0.,0.743144825477395));
#33603=DIRECTION('',(-0.0427321293319654,-0.577350269189632,0.81537760074055));
#33604=DIRECTION('center_axis',(0.473146789255822,0.707106781186536,0.525482745498768));
#33605=DIRECTION('ref_axis',(0.743144825477395,0.,-0.669130606358858));
#33606=DIRECTION('',(0.743144825477395,0.,-0.669130606358858));
#33607=DIRECTION('',(0.815377600740551,-0.577350269189633,0.0427321293319271));
#33608=DIRECTION('center_axis',(0.52548274549876,0.707106781186547,-0.473146789255815));
#33609=DIRECTION('ref_axis',(-0.669130606358858,0.,-0.743144825477395));
#33610=DIRECTION('',(-0.669130606358858,0.,-0.743144825477395));
#33611=DIRECTION('center_axis',(0.743144825477395,0.,-0.669130606358858));
#33612=DIRECTION('ref_axis',(0.669130606358858,0.,0.743144825477395));
#33613=DIRECTION('',(0.,-1.,0.));
#33614=DIRECTION('',(0.669130606358858,0.,0.743144825477395));
#33615=DIRECTION('center_axis',(-0.669130606358858,0.,-0.743144825477395));
#33616=DIRECTION('ref_axis',(0.743144825477395,0.,-0.669130606358858));
#33617=DIRECTION('',(0.,-1.,0.));
#33618=DIRECTION('',(0.743144825477395,0.,-0.669130606358858));
#33619=DIRECTION('center_axis',(-0.743144825477395,0.,0.669130606358858));
#33620=DIRECTION('ref_axis',(-0.669130606358858,0.,-0.743144825477395));
#33621=DIRECTION('',(-0.669130606358858,0.,-0.743144825477395));
#33622=DIRECTION('center_axis',(-0.415626937777453,0.707106781186548,0.572061402817684));
#33623=DIRECTION('ref_axis',(0.809016994374947,0.,0.587785252292473));
#33624=DIRECTION('',(0.809016994374947,0.,0.587785252292473));
#33625=DIRECTION('',(0.127728205844587,-0.577350269189632,0.806444153118108));
#33626=DIRECTION('center_axis',(0.572061402817692,0.707106781186538,0.415626937777459));
#33627=DIRECTION('ref_axis',(0.587785252292473,0.,-0.809016994374947));
#33628=DIRECTION('',(0.587785252292473,0.,-0.809016994374947));
#33629=DIRECTION('',(0.806444153118105,-0.577350269189629,-0.127728205844619));
#33630=DIRECTION('center_axis',(0.415626937777454,0.707106781186546,-0.572061402817685));
#33631=DIRECTION('ref_axis',(-0.809016994374947,0.,-0.587785252292473));
#33632=DIRECTION('',(-0.809016994374947,0.,-0.587785252292473));
#33633=DIRECTION('center_axis',(0.587785252292473,0.,-0.809016994374947));
#33634=DIRECTION('ref_axis',(0.809016994374947,0.,0.587785252292473));
#33635=DIRECTION('',(0.,-1.,0.));
#33636=DIRECTION('',(0.809016994374947,0.,0.587785252292473));
#33637=DIRECTION('center_axis',(-0.809016994374947,0.,-0.587785252292473));
#33638=DIRECTION('ref_axis',(0.587785252292473,0.,-0.809016994374947));
#33639=DIRECTION('',(0.,-1.,0.));
#33640=DIRECTION('',(0.587785252292473,0.,-0.809016994374947));
#33641=DIRECTION('center_axis',(-0.587785252292473,0.,0.809016994374947));
#33642=DIRECTION('ref_axis',(-0.809016994374947,0.,-0.587785252292473));
#33643=DIRECTION('',(-0.809016994374947,0.,-0.587785252292473));
#33644=DIRECTION('center_axis',(-0.287606238475952,0.707106781186546,0.645974188021252));
#33645=DIRECTION('ref_axis',(0.913545457642601,0.,0.406736643075801));
#33646=DIRECTION('',(0.913545457642601,0.,0.406736643075801));
#33647=DIRECTION('',(0.292606205517837,-0.577350269189621,0.76226522625601));
#33648=DIRECTION('center_axis',(0.645974188021245,0.707106781186554,0.287606238475949));
#33649=DIRECTION('ref_axis',(0.406736643075801,0.,-0.913545457642601));
#33650=DIRECTION('',(0.406736643075801,0.,-0.913545457642601));
#33651=DIRECTION('',(0.762265226256017,-0.577350269189622,-0.292606205517818));
#33652=DIRECTION('center_axis',(0.287606238475951,0.707106781186549,-0.64597418802125));
#33653=DIRECTION('ref_axis',(-0.913545457642601,0.,-0.406736643075801));
#33654=DIRECTION('',(-0.913545457642601,0.,-0.406736643075801));
#33655=DIRECTION('center_axis',(0.406736643075801,0.,-0.913545457642601));
#33656=DIRECTION('ref_axis',(0.913545457642601,0.,0.406736643075801));
#33657=DIRECTION('',(0.,-1.,0.));
#33658=DIRECTION('',(0.913545457642601,0.,0.406736643075801));
#33659=DIRECTION('center_axis',(-0.913545457642601,0.,-0.406736643075801));
#33660=DIRECTION('ref_axis',(0.406736643075801,0.,-0.913545457642601));
#33661=DIRECTION('',(0.,-1.,0.));
#33662=DIRECTION('',(0.406736643075801,0.,-0.913545457642601));
#33663=DIRECTION('center_axis',(-0.406736643075801,0.,0.913545457642601));
#33664=DIRECTION('ref_axis',(-0.913545457642601,0.,-0.406736643075801));
#33665=DIRECTION('',(-0.913545457642601,0.,-0.406736643075801));
#33666=DIRECTION('center_axis',(-0.147015766465199,0.707106781186546,0.691654801480227));
#33667=DIRECTION('ref_axis',(0.978147600733805,0.,0.20791169081776));
#33668=DIRECTION('',(0.978147600733805,0.,0.20791169081776));
#33669=DIRECTION('',(0.444695909929548,-0.577350269189626,0.684771651252151));
#33670=DIRECTION('center_axis',(0.691654801480234,0.707106781186539,0.147015766465201));
#33671=DIRECTION('ref_axis',(0.20791169081776,0.,-0.978147600733805));
#33672=DIRECTION('',(0.20791169081776,0.,-0.978147600733805));
#33673=DIRECTION('',(0.68477165125215,-0.577350269189629,-0.444695909929547));
#33674=DIRECTION('center_axis',(0.147015766465199,0.707106781186547,-0.691654801480226));
#33675=DIRECTION('ref_axis',(-0.978147600733805,0.,-0.20791169081776));
#33676=DIRECTION('',(-0.978147600733805,0.,-0.20791169081776));
#33677=DIRECTION('center_axis',(0.20791169081776,0.,-0.978147600733806));
#33678=DIRECTION('ref_axis',(0.978147600733805,0.,0.20791169081776));
#33679=DIRECTION('',(0.,-1.,0.));
#33680=DIRECTION('',(0.978147600733805,0.,0.20791169081776));
#33681=DIRECTION('center_axis',(-0.978147600733806,0.,-0.20791169081776));
#33682=DIRECTION('ref_axis',(0.20791169081776,0.,-0.978147600733805));
#33683=DIRECTION('',(0.,-1.,0.));
#33684=DIRECTION('',(0.20791169081776,0.,-0.978147600733805));
#33685=DIRECTION('center_axis',(-0.20791169081776,0.,0.978147600733806));
#33686=DIRECTION('ref_axis',(-0.978147600733805,0.,-0.20791169081776));
#33687=DIRECTION('',(-0.978147600733805,0.,-0.20791169081776));
#33688=DIRECTION('center_axis',(0.707106781186548,-0.707106781186548,0.));
#33689=DIRECTION('ref_axis',(0.,0.,-1.));
#33690=DIRECTION('',(0.,0.,-1.));
#33691=DIRECTION('',(-0.577350269189625,-0.577350269189625,-0.577350269189627));
#33692=DIRECTION('',(0.,0.,1.));
#33693=DIRECTION('',(-0.577350269189625,-0.577350269189625,0.577350269189627));
#33694=DIRECTION('center_axis',(0.,-0.707106781186549,-0.707106781186546));
#33695=DIRECTION('ref_axis',(-1.,0.,0.));
#33696=DIRECTION('',(1.,0.,0.));
#33697=DIRECTION('',(-1.,0.,0.));
#33698=DIRECTION('center_axis',(0.,-1.,0.));
#33699=DIRECTION('ref_axis',(0.,0.,-1.));
#33700=DIRECTION('',(1.,0.,0.));
#33701=DIRECTION('',(0.978147600733805,0.,0.20791169081776));
#33702=DIRECTION('',(0.20791169081776,0.,-0.978147600733805));
#33703=DIRECTION('',(-0.978147600733805,0.,-0.20791169081776));
#33704=DIRECTION('',(0.913545457642601,0.,0.406736643075801));
#33705=DIRECTION('',(0.406736643075801,0.,-0.913545457642601));
#33706=DIRECTION('',(-0.913545457642601,0.,-0.406736643075801));
#33707=DIRECTION('',(0.809016994374947,0.,0.587785252292473));
#33708=DIRECTION('',(0.587785252292473,0.,-0.809016994374947));
#33709=DIRECTION('',(-0.809016994374947,0.,-0.587785252292473));
#33710=DIRECTION('',(0.669130606358858,0.,0.743144825477395));
#33711=DIRECTION('',(0.743144825477395,0.,-0.669130606358858));
#33712=DIRECTION('',(-0.669130606358858,0.,-0.743144825477395));
#33713=DIRECTION('',(0.499999999999999,0.,0.866025403784439));
#33714=DIRECTION('',(0.866025403784439,0.,-0.499999999999999));
#33715=DIRECTION('',(-0.499999999999999,0.,-0.866025403784439));
#33716=DIRECTION('',(0.309016994374947,0.,0.951056516295154));
#33717=DIRECTION('',(0.951056516295154,0.,-0.309016994374947));
#33718=DIRECTION('',(-0.309016994374947,0.,-0.951056516295154));
#33719=DIRECTION('',(0.104528463267653,0.,0.994521895368273));
#33720=DIRECTION('',(0.994521895368273,0.,-0.104528463267653));
#33721=DIRECTION('',(-0.104528463267653,0.,-0.994521895368273));
#33722=DIRECTION('',(-0.104528463267654,0.,0.994521895368273));
#33723=DIRECTION('',(0.994521895368273,0.,0.104528463267654));
#33724=DIRECTION('',(0.104528463267654,0.,-0.994521895368273));
#33725=DIRECTION('',(-0.309016994374948,0.,0.951056516295153));
#33726=DIRECTION('',(0.951056516295153,0.,0.309016994374948));
#33727=DIRECTION('',(0.309016994374948,0.,-0.951056516295153));
#33728=DIRECTION('',(-0.5,0.,0.866025403784438));
#33729=DIRECTION('',(0.866025403784438,0.,0.5));
#33730=DIRECTION('',(0.5,0.,-0.866025403784438));
#33731=DIRECTION('',(-0.669130606358858,0.,0.743144825477394));
#33732=DIRECTION('',(0.743144825477394,0.,0.669130606358858));
#33733=DIRECTION('',(0.669130606358858,0.,-0.743144825477394));
#33734=DIRECTION('',(-0.809016994374947,0.,0.587785252292473));
#33735=DIRECTION('',(0.587785252292473,0.,0.809016994374947));
#33736=DIRECTION('',(0.809016994374947,0.,-0.587785252292473));
#33737=DIRECTION('',(-0.913545457642601,0.,0.4067366430758));
#33738=DIRECTION('',(0.4067366430758,0.,0.913545457642601));
#33739=DIRECTION('',(0.913545457642601,0.,-0.4067366430758));
#33740=DIRECTION('',(-0.978147600733806,0.,0.207911690817759));
#33741=DIRECTION('',(0.207911690817759,0.,0.978147600733806));
#33742=DIRECTION('',(0.978147600733806,0.,-0.207911690817759));
#33743=DIRECTION('',(-1.,0.,-1.22464679914735E-16));
#33744=DIRECTION('',(-1.22464679914735E-16,0.,1.));
#33745=DIRECTION('',(1.,0.,1.22464679914735E-16));
#33746=DIRECTION('',(-0.978147600733805,0.,-0.20791169081776));
#33747=DIRECTION('',(-0.20791169081776,0.,0.978147600733805));
#33748=DIRECTION('',(0.978147600733805,0.,0.20791169081776));
#33749=DIRECTION('',(-0.913545457642601,0.,-0.4067366430758));
#33750=DIRECTION('',(-0.4067366430758,0.,0.913545457642601));
#33751=DIRECTION('',(0.913545457642601,0.,0.4067366430758));
#33752=DIRECTION('',(-0.809016994374947,0.,-0.587785252292473));
#33753=DIRECTION('',(-0.587785252292473,0.,0.809016994374947));
#33754=DIRECTION('',(0.809016994374947,0.,0.587785252292473));
#33755=DIRECTION('',(-0.669130606358858,0.,-0.743144825477394));
#33756=DIRECTION('',(-0.743144825477394,0.,0.669130606358858));
#33757=DIRECTION('',(0.669130606358858,0.,0.743144825477394));
#33758=DIRECTION('',(-0.5,0.,-0.866025403784439));
#33759=DIRECTION('',(-0.866025403784439,0.,0.5));
#33760=DIRECTION('',(0.5,0.,0.866025403784439));
#33761=DIRECTION('',(-0.309016994374947,0.,-0.951056516295154));
#33762=DIRECTION('',(-0.951056516295154,0.,0.309016994374947));
#33763=DIRECTION('',(0.309016994374947,0.,0.951056516295154));
#33764=DIRECTION('',(-0.104528463267653,0.,-0.994521895368273));
#33765=DIRECTION('',(-0.994521895368273,0.,0.104528463267653));
#33766=DIRECTION('',(0.104528463267653,0.,0.994521895368273));
#33767=DIRECTION('',(0.104528463267654,0.,-0.994521895368273));
#33768=DIRECTION('',(-0.994521895368273,0.,-0.104528463267654));
#33769=DIRECTION('',(-0.104528463267654,0.,0.994521895368273));
#33770=DIRECTION('',(0.309016994374948,0.,-0.951056516295154));
#33771=DIRECTION('',(-0.951056516295154,0.,-0.309016994374948));
#33772=DIRECTION('',(-0.309016994374948,0.,0.951056516295154));
#33773=DIRECTION('',(0.5,0.,-0.866025403784439));
#33774=DIRECTION('',(-0.866025403784439,0.,-0.5));
#33775=DIRECTION('',(-0.5,0.,0.866025403784439));
#33776=DIRECTION('',(0.669130606358858,0.,-0.743144825477394));
#33777=DIRECTION('',(-0.743144825477394,0.,-0.669130606358858));
#33778=DIRECTION('',(-0.669130606358858,0.,0.743144825477394));
#33779=DIRECTION('',(0.809016994374947,0.,-0.587785252292473));
#33780=DIRECTION('',(-0.587785252292473,0.,-0.809016994374947));
#33781=DIRECTION('',(-0.809016994374947,0.,0.587785252292473));
#33782=DIRECTION('',(0.913545457642601,0.,-0.4067366430758));
#33783=DIRECTION('',(-0.4067366430758,0.,-0.913545457642601));
#33784=DIRECTION('',(-0.913545457642601,0.,0.4067366430758));
#33785=DIRECTION('',(0.978147600733806,0.,-0.207911690817759));
#33786=DIRECTION('',(-0.207911690817759,0.,-0.978147600733806));
#33787=DIRECTION('',(-0.978147600733806,0.,0.207911690817759));
#33788=DIRECTION('',(1.,0.,0.));
#33789=DIRECTION('',(0.,0.,-1.));
#33790=DIRECTION('',(-1.,0.,0.));
#33791=DIRECTION('center_axis',(0.,1.,0.));
#33792=DIRECTION('ref_axis',(1.,0.,0.));
#33793=DIRECTION('',(-1.,0.,0.));
#33794=DIRECTION('',(0.,0.,1.));
#33795=DIRECTION('',(1.,0.,0.));
#33796=DIRECTION('center_axis',(0.,1.,0.));
#33797=DIRECTION('ref_axis',(1.,0.,0.));
#33798=DIRECTION('center_axis',(0.,-0.707106781186549,0.707106781186546));
#33799=DIRECTION('ref_axis',(1.,0.,0.));
#33800=DIRECTION('',(-1.,0.,0.));
#33801=DIRECTION('center_axis',(0.691654801480234,-0.707106781186539,-0.1470157664652));
#33802=DIRECTION('ref_axis',(-0.207911690817759,0.,-0.978147600733805));
#33803=DIRECTION('',(0.68477165125215,0.577350269189629,0.444695909929547));
#33804=DIRECTION('',(0.207911690817759,0.,0.978147600733806));
#33805=DIRECTION('',(-0.444695909929537,-0.577350269189628,0.684771651252156));
#33806=DIRECTION('center_axis',(0.147015766465198,-0.707106781186549,0.691654801480225));
#33807=DIRECTION('ref_axis',(0.978147600733806,0.,-0.207911690817759));
#33808=DIRECTION('',(-0.978147600733806,0.,0.207911690817759));
#33809=DIRECTION('center_axis',(-0.147015766465198,-0.70710678118655,-0.691654801480224));
#33810=DIRECTION('ref_axis',(-0.978147600733806,0.,0.207911690817759));
#33811=DIRECTION('',(0.978147600733806,0.,-0.207911690817759));
#33812=DIRECTION('center_axis',(0.64597418802127,-0.707106781186527,-0.287606238475959));
#33813=DIRECTION('ref_axis',(-0.4067366430758,0.,-0.913545457642601));
#33814=DIRECTION('',(0.76226522625599,0.577350269189631,0.292606205517868));
#33815=DIRECTION('',(0.4067366430758,0.,0.913545457642601));
#33816=DIRECTION('',(-0.292606205517786,-0.577350269189647,0.762265226256009));
#33817=DIRECTION('center_axis',(0.287606238475944,-0.707106781186565,0.645974188021235));
#33818=DIRECTION('ref_axis',(0.913545457642601,0.,-0.4067366430758));
#33819=DIRECTION('',(-0.913545457642601,0.,0.4067366430758));
#33820=DIRECTION('center_axis',(-0.287606238475955,-0.707106781186538,-0.64597418802126));
#33821=DIRECTION('ref_axis',(-0.913545457642601,0.,0.4067366430758));
#33822=DIRECTION('',(0.913545457642601,0.,-0.4067366430758));
#33823=DIRECTION('center_axis',(0.4067366430758,0.,0.913545457642601));
#33824=DIRECTION('ref_axis',(0.913545457642601,0.,-0.4067366430758));
#33825=DIRECTION('',(0.,1.,0.));
#33826=DIRECTION('',(0.913545457642601,0.,-0.4067366430758));
#33827=DIRECTION('center_axis',(-0.913545457642601,0.,0.4067366430758));
#33828=DIRECTION('ref_axis',(0.4067366430758,0.,0.913545457642601));
#33829=DIRECTION('',(0.,1.,0.));
#33830=DIRECTION('',(0.4067366430758,0.,0.913545457642601));
#33831=DIRECTION('center_axis',(0.572061402817685,-0.707106781186546,-0.415626937777454));
#33832=DIRECTION('ref_axis',(-0.587785252292473,0.,-0.809016994374947));
#33833=DIRECTION('',(0.806444153118111,0.577350269189624,0.127728205844605));
#33834=DIRECTION('',(0.587785252292473,0.,0.809016994374947));
#33835=DIRECTION('',(-0.127728205844611,-0.577350269189624,0.80644415311811));
#33836=DIRECTION('center_axis',(0.415626937777451,-0.707106781186551,0.572061402817681));
#33837=DIRECTION('ref_axis',(0.809016994374947,0.,-0.587785252292473));
#33838=DIRECTION('',(-0.809016994374947,0.,0.587785252292473));
#33839=DIRECTION('center_axis',(-0.415626937777456,-0.707106781186543,-0.572061402817688));
#33840=DIRECTION('ref_axis',(-0.809016994374947,0.,0.587785252292473));
#33841=DIRECTION('',(0.809016994374947,0.,-0.587785252292473));
#33842=DIRECTION('center_axis',(0.473146789255825,-0.707106781186533,-0.525482745498769));
#33843=DIRECTION('ref_axis',(-0.743144825477394,0.,-0.669130606358858));
#33844=DIRECTION('',(0.815377600740556,0.577350269189627,-0.0427321293319138));
#33845=DIRECTION('',(0.743144825477394,0.,0.669130606358858));
#33846=DIRECTION('',(0.0427321293319529,-0.577350269189635,0.815377600740548));
#33847=DIRECTION('center_axis',(0.525482745498748,-0.707106781186563,0.473146789255805));
#33848=DIRECTION('ref_axis',(0.669130606358858,0.,-0.743144825477394));
#33849=DIRECTION('',(-0.669130606358858,0.,0.743144825477394));
#33850=DIRECTION('center_axis',(-0.525482745498762,-0.707106781186544,-0.473146789255818));
#33851=DIRECTION('ref_axis',(-0.669130606358858,0.,0.743144825477394));
#33852=DIRECTION('',(0.669130606358858,0.,-0.743144825477394));
#33853=DIRECTION('center_axis',(0.743144825477394,0.,0.669130606358858));
#33854=DIRECTION('ref_axis',(0.669130606358858,0.,-0.743144825477394));
#33855=DIRECTION('',(0.,1.,0.));
#33856=DIRECTION('',(0.669130606358858,0.,-0.743144825477394));
#33857=DIRECTION('center_axis',(-0.669130606358858,0.,0.743144825477394));
#33858=DIRECTION('ref_axis',(0.743144825477394,0.,0.669130606358858));
#33859=DIRECTION('',(0.,1.,0.));
#33860=DIRECTION('',(0.743144825477394,0.,0.669130606358858));
#33861=DIRECTION('center_axis',(0.353553390593272,-0.707106781186551,-0.612372435695792));
#33862=DIRECTION('ref_axis',(-0.866025403784439,0.,-0.5));
#33863=DIRECTION('',(0.788675134594812,0.577350269189624,-0.211324865405195));
#33864=DIRECTION('',(0.866025403784439,0.,0.5));
#33865=DIRECTION('',(0.211324865405161,-0.577350269189619,0.788675134594825));
#33866=DIRECTION('center_axis',(0.612372435695798,-0.707106781186544,0.353553390593276));
#33867=DIRECTION('ref_axis',(0.5,0.,-0.866025403784439));
#33868=DIRECTION('',(-0.5,0.,0.866025403784439));
#33869=DIRECTION('center_axis',(-0.612372435695801,-0.70710678118654,-0.353553390593278));
#33870=DIRECTION('ref_axis',(-0.5,0.,0.866025403784439));
#33871=DIRECTION('',(0.5,0.,-0.866025403784439));
#33872=DIRECTION('center_axis',(0.218508012224414,-0.707106781186536,-0.672498511963969));
#33873=DIRECTION('ref_axis',(-0.951056516295153,0.,-0.309016994374947));
#33874=DIRECTION('',(0.727503780584104,0.577350269189638,-0.370681690810982));
#33875=DIRECTION('',(0.951056516295154,0.,0.309016994374948));
#33876=DIRECTION('',(0.370681690811009,-0.57735026918962,0.727503780584104));
#33877=DIRECTION('center_axis',(0.672498511963958,-0.707106781186547,0.218508012224411));
#33878=DIRECTION('ref_axis',(0.309016994374947,0.,-0.951056516295154));
#33879=DIRECTION('',(-0.309016994374948,0.,0.951056516295154));
#33880=DIRECTION('center_axis',(-0.672498511963955,-0.707106781186549,-0.21850801222441));
#33881=DIRECTION('ref_axis',(-0.309016994374947,0.,0.951056516295154));
#33882=DIRECTION('',(0.309016994374948,0.,-0.951056516295154));
#33883=DIRECTION('center_axis',(0.951056516295154,0.,0.309016994374948));
#33884=DIRECTION('ref_axis',(0.309016994374948,0.,-0.951056516295154));
#33885=DIRECTION('',(0.,1.,0.));
#33886=DIRECTION('',(0.309016994374948,0.,-0.951056516295154));
#33887=DIRECTION('center_axis',(-0.309016994374948,0.,0.951056516295154));
#33888=DIRECTION('ref_axis',(0.951056516295154,0.,0.309016994374948));
#33889=DIRECTION('',(0.,1.,0.));
#33890=DIRECTION('',(0.951056516295154,0.,0.309016994374948));
#33891=DIRECTION('center_axis',(-0.703233176253405,-0.707106781186547,-0.0739127852035669));
#33892=DIRECTION('ref_axis',(-0.104528463267654,0.,0.994521895368273));
#33893=DIRECTION('',(0.513837947600284,-0.57735026918962,0.634537020411419));
#33894=DIRECTION('',(0.104528463267654,0.,-0.994521895368273));
#33895=DIRECTION('center_axis',(0.0739127852035657,-0.707106781186559,-0.703233176253393));
#33896=DIRECTION('ref_axis',(-0.994521895368273,0.,-0.104528463267654));
#33897=DIRECTION('',(0.994521895368273,0.,0.104528463267654));
#33898=DIRECTION('',(0.634537020411406,0.577350269189623,-0.513837947600297));
#33899=DIRECTION('center_axis',(0.703233176253404,-0.707106781186547,0.0739127852035669));
#33900=DIRECTION('ref_axis',(0.104528463267654,0.,-0.994521895368273));
#33901=DIRECTION('',(-0.104528463267654,0.,0.994521895368273));
#33902=DIRECTION('center_axis',(-0.0739127852035663,-0.707106781186551,
-0.703233176253401));
#33903=DIRECTION('ref_axis',(-0.994521895368273,0.,0.104528463267653));
#33904=DIRECTION('',(0.513837947600291,0.577350269189624,-0.634537020411409));
#33905=DIRECTION('',(0.994521895368273,0.,-0.104528463267653));
#33906=DIRECTION('',(0.63453702041141,-0.577350269189627,0.513837947600287));
#33907=DIRECTION('center_axis',(0.703233176253405,-0.707106781186546,-0.0739127852035667));
#33908=DIRECTION('ref_axis',(-0.104528463267653,0.,-0.994521895368273));
#33909=DIRECTION('',(0.104528463267653,0.,0.994521895368273));
#33910=DIRECTION('center_axis',(-0.703233176253403,-0.707106781186549,0.0739127852035665));
#33911=DIRECTION('ref_axis',(0.104528463267653,0.,0.994521895368273));
#33912=DIRECTION('',(-0.104528463267653,0.,-0.994521895368273));
#33913=DIRECTION('center_axis',(-0.218508012224409,-0.707106781186552,-0.672498511963953));
#33914=DIRECTION('ref_axis',(-0.951056516295154,0.,0.309016994374947));
#33915=DIRECTION('',(0.370681690811016,0.577350269189631,-0.727503780584092));
#33916=DIRECTION('',(0.951056516295154,0.,-0.309016994374947));
#33917=DIRECTION('',(0.727503780584105,-0.577350269189631,0.370681690810991));
#33918=DIRECTION('center_axis',(0.672498511963956,-0.707106781186549,-0.21850801222441));
#33919=DIRECTION('ref_axis',(-0.309016994374947,0.,-0.951056516295154));
#33920=DIRECTION('',(0.309016994374947,0.,0.951056516295154));
#33921=DIRECTION('center_axis',(-0.672498511963956,-0.70710678118655,0.21850801222441));
#33922=DIRECTION('ref_axis',(0.309016994374947,0.,0.951056516295154));
#33923=DIRECTION('',(-0.309016994374947,0.,-0.951056516295154));
#33924=DIRECTION('center_axis',(0.951056516295154,0.,-0.309016994374947));
#33925=DIRECTION('ref_axis',(-0.309016994374947,0.,-0.951056516295154));
#33926=DIRECTION('',(0.,1.,0.));
#33927=DIRECTION('',(-0.309016994374947,0.,-0.951056516295154));
#33928=DIRECTION('center_axis',(0.309016994374947,0.,0.951056516295154));
#33929=DIRECTION('ref_axis',(0.951056516295154,0.,-0.309016994374947));
#33930=DIRECTION('',(0.,1.,0.));
#33931=DIRECTION('',(0.951056516295154,0.,-0.309016994374947));
#33932=DIRECTION('center_axis',(-0.353553390593278,-0.70710678118654,-0.612372435695801));
#33933=DIRECTION('ref_axis',(-0.866025403784439,0.,0.5));
#33934=DIRECTION('',(0.21132486540519,0.577350269189628,-0.788675134594811));
#33935=DIRECTION('',(0.866025403784439,0.,-0.5));
#33936=DIRECTION('',(0.788675134594814,-0.577350269189626,0.211324865405183));
#33937=DIRECTION('center_axis',(0.612372435695794,-0.707106781186548,-0.353553390593274));
#33938=DIRECTION('ref_axis',(-0.5,0.,-0.866025403784439));
#33939=DIRECTION('',(0.5,0.,0.866025403784439));
#33940=DIRECTION('center_axis',(-0.612372435695791,-0.707106781186552,0.353553390593272));
#33941=DIRECTION('ref_axis',(0.5,0.,0.866025403784439));
#33942=DIRECTION('',(-0.5,0.,-0.866025403784439));
#33943=DIRECTION('center_axis',(-0.473146789255817,-0.707106781186544,-0.525482745498761));
#33944=DIRECTION('ref_axis',(-0.743144825477394,0.,0.669130606358858));
#33945=DIRECTION('',(0.0427321293319396,0.57735026918963,-0.815377600740553));
#33946=DIRECTION('',(0.743144825477394,0.,-0.669130606358858));
#33947=DIRECTION('',(0.815377600740554,-0.577350269189626,0.0427321293319778));
#33948=DIRECTION('center_axis',(0.525482745498765,-0.70710678118654,-0.47314678925582));
#33949=DIRECTION('ref_axis',(-0.669130606358858,0.,-0.743144825477394));
#33950=DIRECTION('',(0.669130606358858,0.,0.743144825477394));
#33951=DIRECTION('center_axis',(-0.525482745498768,-0.707106781186536,0.473146789255823));
#33952=DIRECTION('ref_axis',(0.669130606358858,0.,0.743144825477394));
#33953=DIRECTION('',(-0.669130606358858,0.,-0.743144825477394));
#33954=DIRECTION('center_axis',(0.743144825477394,0.,-0.669130606358858));
#33955=DIRECTION('ref_axis',(-0.669130606358858,0.,-0.743144825477394));
#33956=DIRECTION('',(0.,1.,0.));
#33957=DIRECTION('',(-0.669130606358858,0.,-0.743144825477394));
#33958=DIRECTION('center_axis',(0.669130606358858,0.,0.743144825477394));
#33959=DIRECTION('ref_axis',(0.743144825477394,0.,-0.669130606358858));
#33960=DIRECTION('',(0.,1.,0.));
#33961=DIRECTION('',(0.743144825477394,0.,-0.669130606358858));
#33962=DIRECTION('center_axis',(-0.572061402817686,-0.707106781186545,-0.415626937777455));
#33963=DIRECTION('ref_axis',(-0.587785252292473,0.,0.809016994374947));
#33964=DIRECTION('',(-0.127728205844599,0.577350269189625,-0.806444153118111));
#33965=DIRECTION('',(0.587785252292473,0.,-0.809016994374947));
#33966=DIRECTION('',(0.806444153118105,-0.57735026918963,-0.127728205844613));
#33967=DIRECTION('center_axis',(0.415626937777452,-0.707106781186551,-0.572061402817682));
#33968=DIRECTION('ref_axis',(-0.809016994374947,0.,-0.587785252292473));
#33969=DIRECTION('',(0.809016994374947,0.,0.587785252292473));
#33970=DIRECTION('center_axis',(-0.415626937777454,-0.707106781186547,0.572061402817684));
#33971=DIRECTION('ref_axis',(0.809016994374947,0.,0.587785252292473));
#33972=DIRECTION('',(-0.809016994374947,0.,-0.587785252292473));
#33973=DIRECTION('center_axis',(-0.645974188021245,-0.707106781186554,-0.287606238475948));
#33974=DIRECTION('ref_axis',(-0.4067366430758,0.,0.913545457642601));
#33975=DIRECTION('',(-0.292606205517836,0.577350269189618,-0.762265226256012));
#33976=DIRECTION('',(0.4067366430758,0.,-0.913545457642601));
#33977=DIRECTION('',(0.762265226256022,-0.577350269189626,-0.292606205517795));
#33978=DIRECTION('center_axis',(0.287606238475952,-0.707106781186546,-0.645974188021253));
#33979=DIRECTION('ref_axis',(-0.913545457642601,0.,-0.4067366430758));
#33980=DIRECTION('',(0.913545457642601,0.,0.4067366430758));
#33981=DIRECTION('center_axis',(-0.287606238475956,-0.707106781186536,0.645974188021262));
#33982=DIRECTION('ref_axis',(0.913545457642601,0.,0.4067366430758));
#33983=DIRECTION('',(-0.913545457642601,0.,-0.4067366430758));
#33984=DIRECTION('center_axis',(0.4067366430758,0.,-0.913545457642601));
#33985=DIRECTION('ref_axis',(-0.913545457642601,0.,-0.4067366430758));
#33986=DIRECTION('',(0.,1.,0.));
#33987=DIRECTION('',(-0.913545457642601,0.,-0.4067366430758));
#33988=DIRECTION('center_axis',(0.913545457642601,0.,0.4067366430758));
#33989=DIRECTION('ref_axis',(0.4067366430758,0.,-0.913545457642601));
#33990=DIRECTION('',(0.,1.,0.));
#33991=DIRECTION('',(0.4067366430758,0.,-0.913545457642601));
#33992=DIRECTION('center_axis',(-0.691654801480242,-0.70710678118653,-0.147015766465202));
#33993=DIRECTION('ref_axis',(-0.20791169081776,0.,0.978147600733805));
#33994=DIRECTION('',(-0.44469590992953,0.577350269189636,-0.684771651252154));
#33995=DIRECTION('',(0.20791169081776,0.,-0.978147600733805));
#33996=DIRECTION('',(0.684771651252131,-0.577350269189634,-0.44469590992957));
#33997=DIRECTION('center_axis',(0.1470157664652,-0.707106781186543,-0.69165480148023));
#33998=DIRECTION('ref_axis',(-0.978147600733805,0.,-0.20791169081776));
#33999=DIRECTION('',(0.978147600733805,0.,0.20791169081776));
#34000=DIRECTION('center_axis',(-0.147015766465198,-0.707106781186553,0.69165480148022));
#34001=DIRECTION('ref_axis',(0.978147600733805,0.,0.20791169081776));
#34002=DIRECTION('',(-0.978147600733805,0.,-0.20791169081776));
#34003=DIRECTION('center_axis',(-0.707106781186548,-0.707106781186548,-8.65956056235493E-17));
#34004=DIRECTION('ref_axis',(-1.22464679914735E-16,0.,1.));
#34005=DIRECTION('',(-0.577350269189625,0.577350269189625,-0.577350269189627));
#34006=DIRECTION('',(1.22464679914735E-16,0.,-1.));
#34007=DIRECTION('',(0.577350269189633,-0.57735026918962,-0.577350269189624));
#34008=DIRECTION('center_axis',(8.65956056235492E-17,-0.707106781186549,
-0.707106781186546));
#34009=DIRECTION('ref_axis',(-1.,0.,-1.22464679914735E-16));
#34010=DIRECTION('',(1.,0.,1.22464679914735E-16));
#34011=DIRECTION('center_axis',(-8.65956056235491E-17,-0.707106781186549,
0.707106781186546));
#34012=DIRECTION('ref_axis',(1.,0.,1.22464679914735E-16));
#34013=DIRECTION('',(-1.,0.,-1.22464679914735E-16));
#34014=DIRECTION('center_axis',(1.22464679914735E-16,0.,-1.));
#34015=DIRECTION('ref_axis',(-1.,0.,-1.22464679914735E-16));
#34016=DIRECTION('',(0.,1.,0.));
#34017=DIRECTION('',(-1.,0.,-1.22464679914735E-16));
#34018=DIRECTION('center_axis',(1.,0.,1.22464679914735E-16));
#34019=DIRECTION('ref_axis',(1.22464679914735E-16,0.,-1.));
#34020=DIRECTION('',(0.,1.,0.));
#34021=DIRECTION('',(1.22464679914735E-16,0.,-1.));
#34022=DIRECTION('center_axis',(-0.691654801480235,-0.707106781186538,0.1470157664652));
#34023=DIRECTION('ref_axis',(0.207911690817759,0.,0.978147600733806));
#34024=DIRECTION('',(-0.68477165125214,0.577350269189631,-0.444695909929558));
#34025=DIRECTION('',(-0.207911690817759,0.,-0.978147600733806));
#34026=DIRECTION('',(0.444695909929528,-0.577350269189634,-0.684771651252158));
#34027=DIRECTION('center_axis',(-0.147015766465198,-0.707106781186548,-0.691654801480226));
#34028=DIRECTION('ref_axis',(-0.978147600733806,0.,0.207911690817759));
#34029=DIRECTION('',(0.978147600733806,0.,-0.207911690817759));
#34030=DIRECTION('center_axis',(0.147015766465198,-0.707106781186549,0.691654801480225));
#34031=DIRECTION('ref_axis',(0.978147600733806,0.,-0.207911690817759));
#34032=DIRECTION('',(-0.978147600733806,0.,0.207911690817759));
#34033=DIRECTION('center_axis',(-0.645974188021266,-0.707106781186531,0.287606238475957));
#34034=DIRECTION('ref_axis',(0.4067366430758,0.,0.913545457642601));
#34035=DIRECTION('',(-0.762265226255999,0.577350269189637,-0.292606205517833));
#34036=DIRECTION('',(-0.4067366430758,0.,-0.913545457642601));
#34037=DIRECTION('',(0.29260620551779,-0.57735026918963,-0.762265226256021));
#34038=DIRECTION('center_axis',(-0.28760623847595,-0.707106781186549,-0.64597418802125));
#34039=DIRECTION('ref_axis',(-0.913545457642601,0.,0.4067366430758));
#34040=DIRECTION('',(0.913545457642601,0.,-0.4067366430758));
#34041=DIRECTION('center_axis',(0.287606238475948,-0.707106781186554,0.645974188021245));
#34042=DIRECTION('ref_axis',(0.913545457642601,0.,-0.4067366430758));
#34043=DIRECTION('',(-0.913545457642601,0.,0.4067366430758));
#34044=DIRECTION('center_axis',(-0.4067366430758,0.,-0.913545457642601));
#34045=DIRECTION('ref_axis',(-0.913545457642601,0.,0.4067366430758));
#34046=DIRECTION('',(0.,1.,0.));
#34047=DIRECTION('',(-0.913545457642601,0.,0.4067366430758));
#34048=DIRECTION('center_axis',(0.913545457642601,0.,-0.4067366430758));
#34049=DIRECTION('ref_axis',(-0.4067366430758,0.,-0.913545457642601));
#34050=DIRECTION('',(0.,1.,0.));
#34051=DIRECTION('',(-0.4067366430758,0.,-0.913545457642601));
#34052=DIRECTION('center_axis',(-0.572061402817692,-0.707106781186538,0.415626937777459));
#34053=DIRECTION('ref_axis',(0.587785252292473,0.,0.809016994374947));
#34054=DIRECTION('',(-0.806444153118102,0.577350269189636,-0.127728205844608));
#34055=DIRECTION('',(-0.587785252292473,0.,-0.809016994374947));
#34056=DIRECTION('',(0.127728205844599,-0.577350269189625,-0.806444153118111));
#34057=DIRECTION('center_axis',(-0.415626937777457,-0.707106781186541,-0.57206140281769));
#34058=DIRECTION('ref_axis',(-0.809016994374947,0.,0.587785252292473));
#34059=DIRECTION('',(0.809016994374947,0.,-0.587785252292473));
#34060=DIRECTION('center_axis',(0.415626937777451,-0.707106781186552,0.572061402817681));
#34061=DIRECTION('ref_axis',(0.809016994374947,0.,-0.587785252292473));
#34062=DIRECTION('',(-0.809016994374947,0.,0.587785252292473));
#34063=DIRECTION('center_axis',(-0.473146789255816,-0.707106781186547,0.525482745498759));
#34064=DIRECTION('ref_axis',(0.743144825477394,0.,0.669130606358858));
#34065=DIRECTION('',(-0.815377600740555,0.577350269189626,0.0427321293319522));
#34066=DIRECTION('',(-0.743144825477394,0.,-0.669130606358858));
#34067=DIRECTION('',(-0.0427321293319396,-0.57735026918963,-0.815377600740553));
#34068=DIRECTION('center_axis',(-0.525482745498763,-0.707106781186542,-0.473146789255819));
#34069=DIRECTION('ref_axis',(-0.669130606358858,0.,0.743144825477394));
#34070=DIRECTION('',(0.669130606358858,0.,-0.743144825477394));
#34071=DIRECTION('center_axis',(0.525482745498763,-0.707106781186542,0.473146789255819));
#34072=DIRECTION('ref_axis',(0.669130606358858,0.,-0.743144825477394));
#34073=DIRECTION('',(-0.669130606358858,0.,0.743144825477394));
#34074=DIRECTION('center_axis',(-0.743144825477394,0.,-0.669130606358858));
#34075=DIRECTION('ref_axis',(-0.669130606358858,0.,0.743144825477394));
#34076=DIRECTION('',(0.,1.,0.));
#34077=DIRECTION('',(-0.669130606358858,0.,0.743144825477394));
#34078=DIRECTION('center_axis',(0.669130606358858,0.,-0.743144825477394));
#34079=DIRECTION('ref_axis',(-0.743144825477394,0.,-0.669130606358858));
#34080=DIRECTION('',(0.,1.,0.));
#34081=DIRECTION('',(-0.743144825477394,0.,-0.669130606358858));
#34082=DIRECTION('center_axis',(-0.353553390593269,-0.707106781186558,0.612372435695785));
#34083=DIRECTION('ref_axis',(0.866025403784438,0.,0.5));
#34084=DIRECTION('',(0.788675134594818,-0.577350269189616,-0.211324865405193));
#34085=DIRECTION('',(-0.866025403784438,0.,-0.5));
#34086=DIRECTION('',(-0.211324865405179,-0.577350269189617,-0.788675134594822));
#34087=DIRECTION('center_axis',(0.612372435695789,-0.707106781186554,0.353553390593271));
#34088=DIRECTION('ref_axis',(0.5,0.,-0.866025403784438));
#34089=DIRECTION('',(-0.5,0.,0.866025403784438));
#34090=DIRECTION('center_axis',(-0.612372435695789,-0.707106781186554,-0.353553390593271));
#34091=DIRECTION('ref_axis',(-0.5,0.,0.866025403784438));
#34092=DIRECTION('',(0.5,0.,-0.866025403784438));
#34093=DIRECTION('center_axis',(-0.218508012224412,-0.707106781186544,0.67249851196396));
#34094=DIRECTION('ref_axis',(0.951056516295153,0.,0.309016994374948));
#34095=DIRECTION('',(-0.727503780584099,0.577350269189631,0.370681690811003));
#34096=DIRECTION('',(-0.951056516295153,0.,-0.309016994374948));
#34097=DIRECTION('',(-0.370681690811016,-0.577350269189631,-0.727503780584092));
#34098=DIRECTION('center_axis',(-0.672498511963956,-0.707106781186549,-0.21850801222441));
#34099=DIRECTION('ref_axis',(-0.309016994374948,0.,0.951056516295154));
#34100=DIRECTION('',(0.309016994374948,0.,-0.951056516295153));
#34101=DIRECTION('center_axis',(0.672498511963956,-0.707106781186549,0.21850801222441));
#34102=DIRECTION('ref_axis',(0.309016994374948,0.,-0.951056516295154));
#34103=DIRECTION('',(-0.309016994374948,0.,0.951056516295153));
#34104=DIRECTION('center_axis',(-0.0739127852035669,-0.707106781186551,
0.703233176253401));
#34105=DIRECTION('ref_axis',(0.994521895368273,0.,0.104528463267654));
#34106=DIRECTION('',(-0.634537020411406,0.577350269189623,0.513837947600297));
#34107=DIRECTION('',(-0.994521895368273,0.,-0.104528463267654));
#34108=DIRECTION('',(-0.513837947600291,-0.577350269189624,-0.634537020411409));
#34109=DIRECTION('center_axis',(-0.703233176253405,-0.707106781186547,-0.0739127852035674));
#34110=DIRECTION('ref_axis',(-0.104528463267654,0.,0.994521895368273));
#34111=DIRECTION('',(0.104528463267654,0.,-0.994521895368273));
#34112=DIRECTION('center_axis',(0.703233176253405,-0.707106781186547,0.0739127852035674));
#34113=DIRECTION('ref_axis',(0.104528463267654,0.,-0.994521895368273));
#34114=DIRECTION('',(-0.104528463267654,0.,0.994521895368273));
#34115=DIRECTION('center_axis',(-0.994521895368273,0.,-0.104528463267654));
#34116=DIRECTION('ref_axis',(-0.104528463267654,0.,0.994521895368273));
#34117=DIRECTION('',(0.,1.,0.));
#34118=DIRECTION('',(-0.104528463267654,0.,0.994521895368273));
#34119=DIRECTION('center_axis',(0.104528463267654,0.,-0.994521895368273));
#34120=DIRECTION('ref_axis',(-0.994521895368273,0.,-0.104528463267654));
#34121=DIRECTION('',(0.,1.,0.));
#34122=DIRECTION('',(-0.994521895368273,0.,-0.104528463267654));
#34123=DIRECTION('center_axis',(0.0739127852035652,-0.707106781186559,0.703233176253393));
#34124=DIRECTION('ref_axis',(0.994521895368273,0.,-0.104528463267653));
#34125=DIRECTION('',(-0.513837947600285,0.577350269189621,0.634537020411417));
#34126=DIRECTION('',(-0.994521895368273,0.,0.104528463267653));
#34127=DIRECTION('',(-0.6345370204114,-0.57735026918962,-0.513837947600307));
#34128=DIRECTION('center_axis',(-0.703233176253405,-0.707106781186547,0.0739127852035665));
#34129=DIRECTION('ref_axis',(0.104528463267653,0.,0.994521895368274));
#34130=DIRECTION('',(-0.104528463267653,0.,-0.994521895368273));
#34131=DIRECTION('center_axis',(0.703233176253406,-0.707106781186546,-0.0739127852035666));
#34132=DIRECTION('ref_axis',(-0.104528463267653,0.,-0.994521895368273));
#34133=DIRECTION('',(0.104528463267653,0.,0.994521895368273));
#34134=DIRECTION('center_axis',(0.218508012224411,-0.707106781186545,0.67249851196396));
#34135=DIRECTION('ref_axis',(0.951056516295154,0.,-0.309016994374947));
#34136=DIRECTION('',(-0.370681690811007,0.577350269189627,0.7275037805841));
#34137=DIRECTION('',(-0.951056516295154,0.,0.309016994374947));
#34138=DIRECTION('',(-0.7275037805841,-0.577350269189629,-0.370681690811002));
#34139=DIRECTION('center_axis',(-0.672498511963959,-0.707106781186545,0.218508012224411));
#34140=DIRECTION('ref_axis',(0.309016994374947,0.,0.951056516295154));
#34141=DIRECTION('',(-0.309016994374947,0.,-0.951056516295154));
#34142=DIRECTION('center_axis',(0.672498511963956,-0.707106781186549,-0.21850801222441));
#34143=DIRECTION('ref_axis',(-0.309016994374947,0.,-0.951056516295154));
#34144=DIRECTION('',(0.309016994374947,0.,0.951056516295154));
#34145=DIRECTION('center_axis',(-0.951056516295154,0.,0.309016994374947));
#34146=DIRECTION('ref_axis',(0.309016994374947,0.,0.951056516295154));
#34147=DIRECTION('',(0.,1.,0.));
#34148=DIRECTION('',(0.309016994374947,0.,0.951056516295154));
#34149=DIRECTION('center_axis',(-0.309016994374947,0.,-0.951056516295154));
#34150=DIRECTION('ref_axis',(-0.951056516295154,0.,0.309016994374947));
#34151=DIRECTION('',(0.,1.,0.));
#34152=DIRECTION('',(-0.951056516295154,0.,0.309016994374947));
#34153=DIRECTION('center_axis',(0.353553390593277,-0.70710678118654,0.612372435695802));
#34154=DIRECTION('ref_axis',(0.866025403784439,0.,-0.499999999999999));
#34155=DIRECTION('',(-0.211324865405186,0.577350269189634,0.788675134594807));
#34156=DIRECTION('',(-0.866025403784439,0.,0.499999999999999));
#34157=DIRECTION('',(-0.788675134594814,-0.577350269189626,-0.211324865405183));
#34158=DIRECTION('center_axis',(-0.612372435695802,-0.70710678118654,0.353553390593277));
#34159=DIRECTION('ref_axis',(0.499999999999999,0.,0.866025403784439));
#34160=DIRECTION('',(-0.499999999999999,0.,-0.866025403784439));
#34161=DIRECTION('center_axis',(0.612372435695792,-0.707106781186551,-0.353553390593272));
#34162=DIRECTION('ref_axis',(-0.499999999999999,0.,-0.866025403784439));
#34163=DIRECTION('',(0.499999999999999,0.,0.866025403784439));
#34164=DIRECTION('center_axis',(0.473146789255817,-0.707106781186544,0.525482745498762));
#34165=DIRECTION('ref_axis',(0.743144825477395,0.,-0.669130606358858));
#34166=DIRECTION('',(-0.0427321293319524,0.577350269189629,0.815377600740553));
#34167=DIRECTION('',(-0.743144825477395,0.,0.669130606358858));
#34168=DIRECTION('',(-0.81537760074055,-0.577350269189632,-0.0427321293319527));
#34169=DIRECTION('center_axis',(-0.525482745498762,-0.707106781186544,0.473146789255817));
#34170=DIRECTION('ref_axis',(0.669130606358858,0.,0.743144825477395));
#34171=DIRECTION('',(-0.669130606358858,0.,-0.743144825477395));
#34172=DIRECTION('center_axis',(0.525482745498764,-0.707106781186541,-0.473146789255819));
#34173=DIRECTION('ref_axis',(-0.669130606358858,0.,-0.743144825477395));
#34174=DIRECTION('',(0.669130606358858,0.,0.743144825477395));
#34175=DIRECTION('center_axis',(-0.743144825477395,0.,0.669130606358858));
#34176=DIRECTION('ref_axis',(0.669130606358858,0.,0.743144825477395));
#34177=DIRECTION('',(0.,1.,0.));
#34178=DIRECTION('',(0.669130606358858,0.,0.743144825477395));
#34179=DIRECTION('center_axis',(-0.669130606358858,0.,-0.743144825477395));
#34180=DIRECTION('ref_axis',(-0.743144825477395,0.,0.669130606358858));
#34181=DIRECTION('',(0.,1.,0.));
#34182=DIRECTION('',(-0.743144825477395,0.,0.669130606358858));
#34183=DIRECTION('center_axis',(0.415626937777451,-0.707106781186552,-0.572061402817681));
#34184=DIRECTION('ref_axis',(-0.809016994374947,0.,-0.587785252292473));
#34185=DIRECTION('',(-0.806444153118105,-0.577350269189629,0.127728205844622));
#34186=DIRECTION('',(0.809016994374947,0.,0.587785252292473));
#34187=DIRECTION('center_axis',(0.572061402817692,-0.707106781186538,0.415626937777459));
#34188=DIRECTION('ref_axis',(0.587785252292473,0.,-0.809016994374947));
#34189=DIRECTION('',(-0.587785252292473,0.,0.809016994374947));
#34190=DIRECTION('',(0.1277282058446,0.577350269189631,0.806444153118107));
#34191=DIRECTION('center_axis',(-0.415626937777453,-0.707106781186549,0.572061402817683));
#34192=DIRECTION('ref_axis',(0.809016994374947,0.,0.587785252292473));
#34193=DIRECTION('',(-0.809016994374947,0.,-0.587785252292473));
#34194=DIRECTION('center_axis',(0.64597418802125,-0.707106781186549,0.287606238475951));
#34195=DIRECTION('ref_axis',(0.406736643075801,0.,-0.913545457642601));
#34196=DIRECTION('',(0.292606205517828,0.577350269189629,0.762265226256007));
#34197=DIRECTION('',(-0.406736643075801,0.,0.913545457642601));
#34198=DIRECTION('',(-0.762265226256014,-0.577350269189619,0.29260620551783));
#34199=DIRECTION('center_axis',(-0.287606238475954,-0.70710678118654,0.645974188021258));
#34200=DIRECTION('ref_axis',(0.913545457642601,0.,0.406736643075801));
#34201=DIRECTION('',(-0.913545457642601,0.,-0.406736643075801));
#34202=DIRECTION('center_axis',(0.287606238475947,-0.707106781186558,-0.645974188021242));
#34203=DIRECTION('ref_axis',(-0.913545457642601,0.,-0.406736643075801));
#34204=DIRECTION('',(0.913545457642601,0.,0.406736643075801));
#34205=DIRECTION('center_axis',(0.691654801480227,-0.707106781186546,0.147015766465199));
#34206=DIRECTION('ref_axis',(0.20791169081776,0.,-0.978147600733805));
#34207=DIRECTION('',(0.444695909929549,0.577350269189628,0.684771651252149));
#34208=DIRECTION('',(-0.20791169081776,0.,0.978147600733805));
#34209=DIRECTION('',(-0.68477165125215,-0.577350269189629,0.444695909929547));
#34210=DIRECTION('center_axis',(-0.1470157664652,-0.707106781186542,0.69165480148023));
#34211=DIRECTION('ref_axis',(0.978147600733805,0.,0.20791169081776));
#34212=DIRECTION('',(-0.978147600733805,0.,-0.20791169081776));
#34213=DIRECTION('center_axis',(0.147015766465199,-0.707106781186549,-0.691654801480225));
#34214=DIRECTION('ref_axis',(-0.978147600733805,0.,-0.20791169081776));
#34215=DIRECTION('',(0.978147600733805,0.,0.20791169081776));
#34216=DIRECTION('center_axis',(-0.20791169081776,0.,0.978147600733806));
#34217=DIRECTION('ref_axis',(0.978147600733805,0.,0.20791169081776));
#34218=DIRECTION('',(0.,1.,0.));
#34219=DIRECTION('',(0.978147600733805,0.,0.20791169081776));
#34220=DIRECTION('center_axis',(-0.978147600733806,0.,-0.20791169081776));
#34221=DIRECTION('ref_axis',(-0.20791169081776,0.,0.978147600733805));
#34222=DIRECTION('',(0.,1.,0.));
#34223=DIRECTION('',(-0.20791169081776,0.,0.978147600733805));
#34224=DIRECTION('center_axis',(0.707106781186548,0.707106781186548,0.));
#34225=DIRECTION('ref_axis',(0.,0.,-1.));
#34226=DIRECTION('',(0.577350269189626,-0.577350269189626,-0.577350269189625));
#34227=DIRECTION('',(0.,0.,-1.));
#34228=DIRECTION('',(-0.577350269189624,0.577350269189627,-0.577350269189626));
#34229=DIRECTION('center_axis',(0.,0.707106781186547,-0.707106781186548));
#34230=DIRECTION('ref_axis',(-1.,0.,0.));
#34231=DIRECTION('center_axis',(0.,-0.707106781186547,0.707106781186548));
#34232=DIRECTION('ref_axis',(0.,0.707106781186548,0.707106781186546));
#34233=DIRECTION('',(-1.,0.,0.));
#34234=DIRECTION('center_axis',(0.,0.707106781186547,0.707106781186548));
#34235=DIRECTION('ref_axis',(1.,0.,0.));
#34236=DIRECTION('',(1.,0.,0.));
#34237=DIRECTION('center_axis',(0.,-0.707106781186547,-0.707106781186548));
#34238=DIRECTION('ref_axis',(0.,-0.707106781186548,0.707106781186546));
#34239=DIRECTION('center_axis',(0.,0.,-1.));
#34240=DIRECTION('ref_axis',(-1.,0.,0.));
#34241=DIRECTION('',(0.,1.,0.));
#34242=DIRECTION('',(-1.,0.,0.));
#34243=DIRECTION('',(0.,-1.,0.));
#34244=DIRECTION('center_axis',(-1.,0.,0.));
#34245=DIRECTION('ref_axis',(0.,0.,1.));
#34246=DIRECTION('',(0.,1.,0.));
#34247=DIRECTION('',(0.,0.,1.));
#34248=DIRECTION('center_axis',(0.,0.,1.));
#34249=DIRECTION('ref_axis',(1.,0.,0.));
#34250=DIRECTION('',(0.,1.,0.));
#34251=DIRECTION('',(1.,0.,0.));
#34252=DIRECTION('center_axis',(0.,1.,0.));
#34253=DIRECTION('ref_axis',(0.,0.,1.));
#34254=DIRECTION('center_axis',(0.,-0.707106781186547,0.707106781186548));
#34255=DIRECTION('ref_axis',(0.,0.707106781186548,0.707106781186546));
#34256=DIRECTION('',(0.,-1.,0.));
#34257=DIRECTION('center_axis',(0.,0.707106781186547,0.707106781186548));
#34258=DIRECTION('ref_axis',(0.,-0.707106781186548,0.707106781186546));
#34259=DIRECTION('center_axis',(0.,0.707106781186547,0.707106781186548));
#34260=DIRECTION('ref_axis',(0.,-0.707106781186548,0.707106781186546));
#34261=DIRECTION('center_axis',(0.707106781186548,-0.707106781186548,0.));
#34262=DIRECTION('ref_axis',(0.,0.,-1.));
#34263=DIRECTION('',(-0.577350269189626,-0.577350269189626,0.577350269189625));
#34264=DIRECTION('',(0.577350269189624,0.577350269189627,0.577350269189626));
#34265=DIRECTION('center_axis',(0.,-0.707106781186547,-0.707106781186548));
#34266=DIRECTION('ref_axis',(-1.,0.,0.));
#34267=DIRECTION('center_axis',(0.,-0.707106781186547,0.707106781186548));
#34268=DIRECTION('ref_axis',(1.,0.,0.));
#34269=DIRECTION('center_axis',(0.,0.707106781186547,-0.707106781186548));
#34270=DIRECTION('ref_axis',(0.,0.707106781186548,0.707106781186546));
#34271=DIRECTION('center_axis',(0.,-0.707106781186547,0.707106781186548));
#34272=DIRECTION('ref_axis',(1.,0.,0.));
#34273=DIRECTION('',(-1.,0.,0.));
#34274=DIRECTION('center_axis',(0.,0.707106781186547,-0.707106781186548));
#34275=DIRECTION('ref_axis',(0.,0.707106781186548,0.707106781186546));
#34276=DIRECTION('',(-0.577350269189626,0.577350269189626,0.577350269189625));
#34277=DIRECTION('center_axis',(-0.707106781186548,-0.707106781186548,0.));
#34278=DIRECTION('ref_axis',(0.,0.,1.));
#34279=DIRECTION('',(-0.577350269189624,0.577350269189627,-0.577350269189626));
#34280=DIRECTION('',(0.,0.,-1.));
#34281=DIRECTION('center_axis',(0.,-0.707106781186547,-0.707106781186548));
#34282=DIRECTION('ref_axis',(-1.,0.,0.));
#34283=DIRECTION('',(1.,0.,0.));
#34284=DIRECTION('center_axis',(0.,0.,-1.));
#34285=DIRECTION('ref_axis',(-1.,0.,0.));
#34286=DIRECTION('',(0.,1.,0.));
#34287=DIRECTION('',(1.,0.,0.));
#34288=DIRECTION('',(0.,1.,0.));
#34289=DIRECTION('center_axis',(1.,0.,0.));
#34290=DIRECTION('ref_axis',(0.,0.,-1.));
#34291=DIRECTION('',(0.,1.,0.));
#34292=DIRECTION('',(0.,0.,1.));
#34293=DIRECTION('center_axis',(0.,0.,1.));
#34294=DIRECTION('ref_axis',(1.,0.,0.));
#34295=DIRECTION('',(-1.,0.,0.));
#34296=DIRECTION('center_axis',(0.,0.707106781186547,0.707106781186548));
#34297=DIRECTION('ref_axis',(1.,0.,0.));
#34298=DIRECTION('center_axis',(0.,-0.707106781186547,-0.707106781186548));
#34299=DIRECTION('ref_axis',(0.,-0.707106781186548,0.707106781186546));
#34300=DIRECTION('',(0.577350269189626,0.577350269189626,-0.577350269189625));
#34301=DIRECTION('center_axis',(-0.707106781186548,0.707106781186548,0.));
#34302=DIRECTION('ref_axis',(0.,0.,1.));
#34303=DIRECTION('',(0.577350269189624,0.577350269189627,0.577350269189626));
#34304=DIRECTION('center_axis',(0.,0.707106781186547,-0.707106781186548));
#34305=DIRECTION('ref_axis',(-1.,0.,0.));
#34306=DIRECTION('center_axis',(0.,-1.,0.));
#34307=DIRECTION('ref_axis',(0.20791169081776,0.,-0.978147600733805));
#34308=DIRECTION('center_axis',(0.20791169081776,0.,-0.978147600733806));
#34309=DIRECTION('ref_axis',(-0.978147600733805,0.,-0.20791169081776));
#34310=DIRECTION('',(-0.978147600733805,0.,-0.20791169081776));
#34311=DIRECTION('center_axis',(0.,1.,0.));
#34312=DIRECTION('ref_axis',(-0.20791169081776,0.,0.978147600733805));
#34313=DIRECTION('center_axis',(0.,-1.,0.));
#34314=DIRECTION('ref_axis',(0.406736643075801,0.,-0.913545457642601));
#34315=DIRECTION('center_axis',(-0.913545457642601,0.,-0.406736643075801));
#34316=DIRECTION('ref_axis',(-0.406736643075801,0.,0.913545457642601));
#34317=DIRECTION('',(0.,1.,0.));
#34318=DIRECTION('',(-0.406736643075801,0.,0.913545457642601));
#34319=DIRECTION('',(0.,1.,0.));
#34320=DIRECTION('center_axis',(0.406736643075801,0.,-0.913545457642601));
#34321=DIRECTION('ref_axis',(-0.913545457642601,0.,-0.406736643075801));
#34322=DIRECTION('',(-0.913545457642601,0.,-0.406736643075801));
#34323=DIRECTION('center_axis',(-0.406736643075801,0.,0.913545457642601));
#34324=DIRECTION('ref_axis',(0.913545457642601,0.,0.406736643075801));
#34325=DIRECTION('',(0.913545457642601,0.,0.406736643075801));
#34326=DIRECTION('center_axis',(0.,1.,0.));
#34327=DIRECTION('ref_axis',(-0.406736643075801,0.,0.913545457642601));
#34328=DIRECTION('center_axis',(0.,-1.,0.));
#34329=DIRECTION('ref_axis',(0.587785252292473,0.,-0.809016994374947));
#34330=DIRECTION('center_axis',(-0.809016994374947,0.,-0.587785252292473));
#34331=DIRECTION('ref_axis',(-0.587785252292473,0.,0.809016994374947));
#34332=DIRECTION('',(0.,1.,0.));
#34333=DIRECTION('',(-0.587785252292473,0.,0.809016994374947));
#34334=DIRECTION('',(0.,1.,0.));
#34335=DIRECTION('center_axis',(0.587785252292473,0.,-0.809016994374947));
#34336=DIRECTION('ref_axis',(-0.809016994374947,0.,-0.587785252292473));
#34337=DIRECTION('',(-0.809016994374947,0.,-0.587785252292473));
#34338=DIRECTION('center_axis',(-0.587785252292473,0.,0.809016994374947));
#34339=DIRECTION('ref_axis',(0.809016994374947,0.,0.587785252292473));
#34340=DIRECTION('',(0.809016994374947,0.,0.587785252292473));
#34341=DIRECTION('center_axis',(0.,1.,0.));
#34342=DIRECTION('ref_axis',(-0.587785252292473,0.,0.809016994374947));
#34343=DIRECTION('center_axis',(0.,-1.,0.));
#34344=DIRECTION('ref_axis',(0.743144825477395,0.,-0.669130606358858));
#34345=DIRECTION('center_axis',(0.743144825477395,0.,-0.669130606358858));
#34346=DIRECTION('ref_axis',(-0.669130606358858,0.,-0.743144825477395));
#34347=DIRECTION('',(-0.669130606358858,0.,-0.743144825477395));
#34348=DIRECTION('center_axis',(0.,1.,0.));
#34349=DIRECTION('ref_axis',(-0.743144825477395,0.,0.669130606358858));
#34350=DIRECTION('center_axis',(0.,-1.,0.));
#34351=DIRECTION('ref_axis',(0.866025403784439,0.,-0.499999999999999));
#34352=DIRECTION('center_axis',(-0.499999999999999,0.,-0.866025403784439));
#34353=DIRECTION('ref_axis',(-0.866025403784439,0.,0.499999999999999));
#34354=DIRECTION('',(0.,1.,0.));
#34355=DIRECTION('',(-0.866025403784439,0.,0.499999999999999));
#34356=DIRECTION('',(0.,1.,0.));
#34357=DIRECTION('center_axis',(0.866025403784439,0.,-0.499999999999999));
#34358=DIRECTION('ref_axis',(-0.499999999999999,0.,-0.866025403784439));
#34359=DIRECTION('',(-0.499999999999999,0.,-0.866025403784439));
#34360=DIRECTION('center_axis',(-0.866025403784439,0.,0.499999999999999));
#34361=DIRECTION('ref_axis',(0.499999999999999,0.,0.866025403784439));
#34362=DIRECTION('',(0.499999999999999,0.,0.866025403784439));
#34363=DIRECTION('center_axis',(0.,1.,0.));
#34364=DIRECTION('ref_axis',(-0.866025403784439,0.,0.499999999999999));
#34365=DIRECTION('center_axis',(0.,-1.,0.));
#34366=DIRECTION('ref_axis',(0.951056516295154,0.,-0.309016994374947));
#34367=DIRECTION('center_axis',(0.951056516295154,0.,-0.309016994374947));
#34368=DIRECTION('ref_axis',(-0.309016994374947,0.,-0.951056516295154));
#34369=DIRECTION('',(-0.309016994374947,0.,-0.951056516295154));
#34370=DIRECTION('center_axis',(0.,1.,0.));
#34371=DIRECTION('ref_axis',(-0.951056516295154,0.,0.309016994374947));
#34372=DIRECTION('center_axis',(0.,-1.,0.));
#34373=DIRECTION('ref_axis',(0.994521895368273,0.,-0.104528463267653));
#34374=DIRECTION('center_axis',(-0.104528463267653,0.,-0.994521895368273));
#34375=DIRECTION('ref_axis',(-0.994521895368273,0.,0.104528463267653));
#34376=DIRECTION('',(0.,1.,0.));
#34377=DIRECTION('',(-0.994521895368273,0.,0.104528463267653));
#34378=DIRECTION('',(0.,1.,0.));
#34379=DIRECTION('center_axis',(0.994521895368273,0.,-0.104528463267653));
#34380=DIRECTION('ref_axis',(-0.104528463267653,0.,-0.994521895368273));
#34381=DIRECTION('',(-0.104528463267653,0.,-0.994521895368273));
#34382=DIRECTION('center_axis',(-0.994521895368273,0.,0.104528463267653));
#34383=DIRECTION('ref_axis',(0.104528463267653,0.,0.994521895368273));
#34384=DIRECTION('',(0.104528463267653,0.,0.994521895368273));
#34385=DIRECTION('center_axis',(0.,1.,0.));
#34386=DIRECTION('ref_axis',(-0.994521895368273,0.,0.104528463267653));
#34387=DIRECTION('center_axis',(0.,-1.,0.));
#34388=DIRECTION('ref_axis',(0.994521895368273,0.,0.104528463267654));
#34389=DIRECTION('center_axis',(0.994521895368273,0.,0.104528463267654));
#34390=DIRECTION('ref_axis',(0.104528463267654,0.,-0.994521895368273));
#34391=DIRECTION('',(0.104528463267654,0.,-0.994521895368273));
#34392=DIRECTION('center_axis',(0.,1.,0.));
#34393=DIRECTION('ref_axis',(-0.994521895368273,0.,-0.104528463267654));
#34394=DIRECTION('center_axis',(0.,-1.,0.));
#34395=DIRECTION('ref_axis',(0.951056516295153,0.,0.309016994374948));
#34396=DIRECTION('center_axis',(0.309016994374948,0.,-0.951056516295154));
#34397=DIRECTION('ref_axis',(-0.951056516295153,0.,-0.309016994374948));
#34398=DIRECTION('',(0.,1.,0.));
#34399=DIRECTION('',(-0.951056516295153,0.,-0.309016994374948));
#34400=DIRECTION('',(0.,1.,0.));
#34401=DIRECTION('center_axis',(0.951056516295154,0.,0.309016994374948));
#34402=DIRECTION('ref_axis',(0.309016994374948,0.,-0.951056516295153));
#34403=DIRECTION('',(0.309016994374948,0.,-0.951056516295153));
#34404=DIRECTION('center_axis',(-0.951056516295154,0.,-0.309016994374948));
#34405=DIRECTION('ref_axis',(-0.309016994374948,0.,0.951056516295153));
#34406=DIRECTION('',(-0.309016994374948,0.,0.951056516295153));
#34407=DIRECTION('center_axis',(0.,1.,0.));
#34408=DIRECTION('ref_axis',(-0.951056516295153,0.,-0.309016994374948));
#34409=DIRECTION('center_axis',(0.,-1.,0.));
#34410=DIRECTION('ref_axis',(0.866025403784438,0.,0.5));
#34411=DIRECTION('center_axis',(0.5,0.,-0.866025403784438));
#34412=DIRECTION('ref_axis',(-0.866025403784438,0.,-0.5));
#34413=DIRECTION('',(0.,1.,0.));
#34414=DIRECTION('',(-0.866025403784438,0.,-0.5));
#34415=DIRECTION('',(0.,1.,0.));
#34416=DIRECTION('center_axis',(0.866025403784438,0.,0.5));
#34417=DIRECTION('ref_axis',(0.5,0.,-0.866025403784438));
#34418=DIRECTION('',(0.5,0.,-0.866025403784438));
#34419=DIRECTION('center_axis',(-0.866025403784438,0.,-0.5));
#34420=DIRECTION('ref_axis',(-0.5,0.,0.866025403784438));
#34421=DIRECTION('',(-0.5,0.,0.866025403784438));
#34422=DIRECTION('center_axis',(0.,1.,0.));
#34423=DIRECTION('ref_axis',(-0.866025403784438,0.,-0.5));
#34424=DIRECTION('center_axis',(0.,-1.,0.));
#34425=DIRECTION('ref_axis',(0.743144825477394,0.,0.669130606358858));
#34426=DIRECTION('center_axis',(0.743144825477394,0.,0.669130606358858));
#34427=DIRECTION('ref_axis',(0.669130606358858,0.,-0.743144825477394));
#34428=DIRECTION('',(0.669130606358858,0.,-0.743144825477394));
#34429=DIRECTION('center_axis',(0.,1.,0.));
#34430=DIRECTION('ref_axis',(-0.743144825477394,0.,-0.669130606358858));
#34431=DIRECTION('center_axis',(0.,-1.,0.));
#34432=DIRECTION('ref_axis',(0.587785252292473,0.,0.809016994374947));
#34433=DIRECTION('center_axis',(0.809016994374948,0.,-0.587785252292473));
#34434=DIRECTION('ref_axis',(-0.587785252292473,0.,-0.809016994374947));
#34435=DIRECTION('',(0.,1.,0.));
#34436=DIRECTION('',(-0.587785252292473,0.,-0.809016994374947));
#34437=DIRECTION('',(0.,1.,0.));
#34438=DIRECTION('center_axis',(0.587785252292473,0.,0.809016994374948));
#34439=DIRECTION('ref_axis',(0.809016994374947,0.,-0.587785252292473));
#34440=DIRECTION('',(0.809016994374947,0.,-0.587785252292473));
#34441=DIRECTION('center_axis',(-0.587785252292473,0.,-0.809016994374948));
#34442=DIRECTION('ref_axis',(-0.809016994374947,0.,0.587785252292473));
#34443=DIRECTION('',(-0.809016994374947,0.,0.587785252292473));
#34444=DIRECTION('center_axis',(0.,1.,0.));
#34445=DIRECTION('ref_axis',(-0.587785252292473,0.,-0.809016994374947));
#34446=DIRECTION('center_axis',(0.,-1.,0.));
#34447=DIRECTION('ref_axis',(0.4067366430758,0.,0.913545457642601));
#34448=DIRECTION('center_axis',(0.4067366430758,0.,0.913545457642601));
#34449=DIRECTION('ref_axis',(0.913545457642601,0.,-0.4067366430758));
#34450=DIRECTION('',(0.913545457642601,0.,-0.4067366430758));
#34451=DIRECTION('center_axis',(0.,1.,0.));
#34452=DIRECTION('ref_axis',(-0.4067366430758,0.,-0.913545457642601));
#34453=DIRECTION('center_axis',(0.,-1.,0.));
#34454=DIRECTION('ref_axis',(0.207911690817759,0.,0.978147600733806));
#34455=DIRECTION('center_axis',(0.978147600733806,0.,-0.207911690817759));
#34456=DIRECTION('ref_axis',(-0.207911690817759,0.,-0.978147600733806));
#34457=DIRECTION('',(0.,1.,0.));
#34458=DIRECTION('',(-0.207911690817759,0.,-0.978147600733806));
#34459=DIRECTION('',(0.,1.,0.));
#34460=DIRECTION('center_axis',(0.207911690817759,0.,0.978147600733806));
#34461=DIRECTION('ref_axis',(0.978147600733806,0.,-0.207911690817759));
#34462=DIRECTION('',(0.978147600733806,0.,-0.207911690817759));
#34463=DIRECTION('center_axis',(-0.207911690817759,0.,-0.978147600733806));
#34464=DIRECTION('ref_axis',(-0.978147600733806,0.,0.207911690817759));
#34465=DIRECTION('',(-0.978147600733806,0.,0.207911690817759));
#34466=DIRECTION('center_axis',(0.,1.,0.));
#34467=DIRECTION('ref_axis',(-0.207911690817759,0.,-0.978147600733806));
#34468=DIRECTION('center_axis',(0.,-1.,0.));
#34469=DIRECTION('ref_axis',(-1.22464679914735E-16,0.,1.));
#34470=DIRECTION('center_axis',(-1.22464679914735E-16,0.,1.));
#34471=DIRECTION('ref_axis',(1.,0.,1.22464679914735E-16));
#34472=DIRECTION('',(1.,0.,1.22464679914735E-16));
#34473=DIRECTION('center_axis',(0.,1.,0.));
#34474=DIRECTION('ref_axis',(1.22464679914735E-16,0.,-1.));
#34475=DIRECTION('center_axis',(0.,-1.,0.));
#34476=DIRECTION('ref_axis',(-0.20791169081776,0.,0.978147600733805));
#34477=DIRECTION('center_axis',(0.978147600733806,0.,0.20791169081776));
#34478=DIRECTION('ref_axis',(0.20791169081776,0.,-0.978147600733805));
#34479=DIRECTION('',(0.,1.,0.));
#34480=DIRECTION('',(0.20791169081776,0.,-0.978147600733805));
#34481=DIRECTION('',(0.,1.,0.));
#34482=DIRECTION('center_axis',(-0.20791169081776,0.,0.978147600733806));
#34483=DIRECTION('ref_axis',(0.978147600733805,0.,0.20791169081776));
#34484=DIRECTION('',(0.978147600733805,0.,0.20791169081776));
#34485=DIRECTION('center_axis',(0.20791169081776,0.,-0.978147600733806));
#34486=DIRECTION('ref_axis',(-0.978147600733805,0.,-0.20791169081776));
#34487=DIRECTION('',(-0.978147600733805,0.,-0.20791169081776));
#34488=DIRECTION('center_axis',(0.,1.,0.));
#34489=DIRECTION('ref_axis',(0.20791169081776,0.,-0.978147600733805));
#34490=DIRECTION('center_axis',(0.,-1.,0.));
#34491=DIRECTION('ref_axis',(-0.4067366430758,0.,0.913545457642601));
#34492=DIRECTION('center_axis',(-0.4067366430758,0.,0.913545457642601));
#34493=DIRECTION('ref_axis',(0.913545457642601,0.,0.4067366430758));
#34494=DIRECTION('',(0.913545457642601,0.,0.4067366430758));
#34495=DIRECTION('center_axis',(0.,1.,0.));
#34496=DIRECTION('ref_axis',(0.4067366430758,0.,-0.913545457642601));
#34497=DIRECTION('center_axis',(0.,-1.,0.));
#34498=DIRECTION('ref_axis',(-0.587785252292473,0.,0.809016994374947));
#34499=DIRECTION('center_axis',(0.809016994374947,0.,0.587785252292473));
#34500=DIRECTION('ref_axis',(0.587785252292473,0.,-0.809016994374947));
#34501=DIRECTION('',(0.,1.,0.));
#34502=DIRECTION('',(0.587785252292473,0.,-0.809016994374947));
#34503=DIRECTION('',(0.,1.,0.));
#34504=DIRECTION('center_axis',(-0.587785252292473,0.,0.809016994374947));
#34505=DIRECTION('ref_axis',(0.809016994374947,0.,0.587785252292473));
#34506=DIRECTION('',(0.809016994374947,0.,0.587785252292473));
#34507=DIRECTION('center_axis',(0.587785252292473,0.,-0.809016994374947));
#34508=DIRECTION('ref_axis',(-0.809016994374947,0.,-0.587785252292473));
#34509=DIRECTION('',(-0.809016994374947,0.,-0.587785252292473));
#34510=DIRECTION('center_axis',(0.,1.,0.));
#34511=DIRECTION('ref_axis',(0.587785252292473,0.,-0.809016994374947));
#34512=DIRECTION('center_axis',(0.,-1.,0.));
#34513=DIRECTION('ref_axis',(-0.743144825477394,0.,0.669130606358858));
#34514=DIRECTION('center_axis',(-0.743144825477394,0.,0.669130606358858));
#34515=DIRECTION('ref_axis',(0.669130606358858,0.,0.743144825477394));
#34516=DIRECTION('',(0.669130606358858,0.,0.743144825477394));
#34517=DIRECTION('center_axis',(0.,1.,0.));
#34518=DIRECTION('ref_axis',(0.743144825477394,0.,-0.669130606358858));
#34519=DIRECTION('center_axis',(-0.866025403784439,0.,0.5));
#34520=DIRECTION('ref_axis',(-0.5,0.,-0.866025403784439));
#34521=DIRECTION('',(-0.5,0.,-0.866025403784439));
#34522=DIRECTION('center_axis',(0.,-1.,0.));
#34523=DIRECTION('ref_axis',(-0.866025403784439,0.,0.5));
#34524=DIRECTION('center_axis',(0.5,0.,0.866025403784439));
#34525=DIRECTION('ref_axis',(0.866025403784439,0.,-0.5));
#34526=DIRECTION('',(0.,1.,0.));
#34527=DIRECTION('',(0.866025403784439,0.,-0.5));
#34528=DIRECTION('',(0.,1.,0.));
#34529=DIRECTION('center_axis',(-0.866025403784439,0.,0.5));
#34530=DIRECTION('ref_axis',(0.5,0.,0.866025403784439));
#34531=DIRECTION('',(0.5,0.,0.866025403784439));
#34532=DIRECTION('center_axis',(0.866025403784439,0.,-0.5));
#34533=DIRECTION('ref_axis',(-0.5,0.,-0.866025403784439));
#34534=DIRECTION('',(-0.5,0.,-0.866025403784439));
#34535=DIRECTION('center_axis',(0.,1.,0.));
#34536=DIRECTION('ref_axis',(0.866025403784439,0.,-0.5));
#34537=DIRECTION('center_axis',(0.,-1.,0.));
#34538=DIRECTION('ref_axis',(-0.951056516295154,0.,0.309016994374947));
#34539=DIRECTION('center_axis',(-0.951056516295154,0.,0.309016994374947));
#34540=DIRECTION('ref_axis',(0.309016994374947,0.,0.951056516295154));
#34541=DIRECTION('',(0.309016994374947,0.,0.951056516295154));
#34542=DIRECTION('center_axis',(0.,1.,0.));
#34543=DIRECTION('ref_axis',(0.951056516295154,0.,-0.309016994374947));
#34544=DIRECTION('center_axis',(0.,-1.,0.));
#34545=DIRECTION('ref_axis',(-0.994521895368273,0.,0.104528463267653));
#34546=DIRECTION('center_axis',(0.104528463267653,0.,0.994521895368273));
#34547=DIRECTION('ref_axis',(0.994521895368273,0.,-0.104528463267653));
#34548=DIRECTION('',(0.,1.,0.));
#34549=DIRECTION('',(0.994521895368273,0.,-0.104528463267653));
#34550=DIRECTION('',(0.,1.,0.));
#34551=DIRECTION('center_axis',(-0.994521895368273,0.,0.104528463267653));
#34552=DIRECTION('ref_axis',(0.104528463267653,0.,0.994521895368273));
#34553=DIRECTION('',(0.104528463267653,0.,0.994521895368273));
#34554=DIRECTION('center_axis',(0.994521895368273,0.,-0.104528463267653));
#34555=DIRECTION('ref_axis',(-0.104528463267653,0.,-0.994521895368273));
#34556=DIRECTION('',(-0.104528463267653,0.,-0.994521895368273));
#34557=DIRECTION('center_axis',(0.,1.,0.));
#34558=DIRECTION('ref_axis',(0.994521895368273,0.,-0.104528463267653));
#34559=DIRECTION('center_axis',(0.,-1.,0.));
#34560=DIRECTION('ref_axis',(-0.994521895368273,0.,-0.104528463267654));
#34561=DIRECTION('center_axis',(-0.104528463267654,0.,0.994521895368273));
#34562=DIRECTION('ref_axis',(0.994521895368273,0.,0.104528463267654));
#34563=DIRECTION('',(0.,1.,0.));
#34564=DIRECTION('',(0.994521895368273,0.,0.104528463267654));
#34565=DIRECTION('',(0.,1.,0.));
#34566=DIRECTION('center_axis',(-0.994521895368273,0.,-0.104528463267654));
#34567=DIRECTION('ref_axis',(-0.104528463267654,0.,0.994521895368273));
#34568=DIRECTION('',(-0.104528463267654,0.,0.994521895368273));
#34569=DIRECTION('center_axis',(0.994521895368273,0.,0.104528463267654));
#34570=DIRECTION('ref_axis',(0.104528463267654,0.,-0.994521895368273));
#34571=DIRECTION('',(0.104528463267654,0.,-0.994521895368273));
#34572=DIRECTION('center_axis',(0.,1.,0.));
#34573=DIRECTION('ref_axis',(0.994521895368273,0.,0.104528463267654));
#34574=DIRECTION('center_axis',(0.,-1.,0.));
#34575=DIRECTION('ref_axis',(-0.951056516295154,0.,-0.309016994374948));
#34576=DIRECTION('',(-0.309016994374948,0.,0.951056516295154));
#34577=DIRECTION('center_axis',(0.951056516295154,0.,0.309016994374948));
#34578=DIRECTION('ref_axis',(-0.309016994374948,0.,0.951056516295154));
#34579=DIRECTION('center_axis',(-0.951056516295154,0.,-0.309016994374948));
#34580=DIRECTION('ref_axis',(-0.309016994374948,0.,0.951056516295154));
#34581=DIRECTION('',(-0.309016994374948,0.,0.951056516295154));
#34582=DIRECTION('center_axis',(0.,1.,0.));
#34583=DIRECTION('ref_axis',(0.951056516295154,0.,0.309016994374948));
#34584=DIRECTION('center_axis',(-0.866025403784439,0.,-0.5));
#34585=DIRECTION('ref_axis',(0.5,0.,-0.866025403784439));
#34586=DIRECTION('',(0.,-1.,0.));
#34587=DIRECTION('',(0.5,0.,-0.866025403784439));
#34588=DIRECTION('center_axis',(0.,-1.,0.));
#34589=DIRECTION('ref_axis',(-0.866025403784439,0.,-0.5));
#34590=DIRECTION('',(-0.866025403784439,0.,-0.5));
#34591=DIRECTION('',(-0.5,0.,0.866025403784439));
#34592=DIRECTION('center_axis',(-0.5,0.,0.866025403784439));
#34593=DIRECTION('ref_axis',(-0.866025403784439,0.,-0.5));
#34594=DIRECTION('',(0.,-1.,0.));
#34595=DIRECTION('center_axis',(0.866025403784439,0.,0.5));
#34596=DIRECTION('ref_axis',(-0.5,0.,0.866025403784439));
#34597=DIRECTION('center_axis',(-0.5,0.,0.866025403784439));
#34598=DIRECTION('ref_axis',(0.866025403784439,0.,0.5));
#34599=DIRECTION('',(0.,1.,0.));
#34600=DIRECTION('',(0.866025403784439,0.,0.5));
#34601=DIRECTION('',(0.,1.,0.));
#34602=DIRECTION('center_axis',(-0.866025403784439,0.,-0.5));
#34603=DIRECTION('ref_axis',(-0.5,0.,0.866025403784439));
#34604=DIRECTION('',(-0.5,0.,0.866025403784439));
#34605=DIRECTION('center_axis',(0.866025403784439,0.,0.5));
#34606=DIRECTION('ref_axis',(0.5,0.,-0.866025403784439));
#34607=DIRECTION('',(0.5,0.,-0.866025403784439));
#34608=DIRECTION('center_axis',(0.,1.,0.));
#34609=DIRECTION('ref_axis',(0.866025403784439,0.,0.5));
#34610=DIRECTION('center_axis',(-0.743144825477394,0.,-0.669130606358858));
#34611=DIRECTION('ref_axis',(0.669130606358858,0.,-0.743144825477394));
#34612=DIRECTION('',(0.,-1.,0.));
#34613=DIRECTION('',(0.669130606358858,0.,-0.743144825477394));
#34614=DIRECTION('center_axis',(0.,-1.,0.));
#34615=DIRECTION('ref_axis',(-0.743144825477394,0.,-0.669130606358858));
#34616=DIRECTION('',(-0.743144825477394,0.,-0.669130606358858));
#34617=DIRECTION('',(-0.669130606358858,0.,0.743144825477394));
#34618=DIRECTION('center_axis',(-0.669130606358858,0.,0.743144825477394));
#34619=DIRECTION('ref_axis',(-0.743144825477394,0.,-0.669130606358858));
#34620=DIRECTION('',(0.,-1.,0.));
#34621=DIRECTION('center_axis',(0.743144825477394,0.,0.669130606358858));
#34622=DIRECTION('ref_axis',(-0.669130606358858,0.,0.743144825477394));
#34623=DIRECTION('center_axis',(-0.743144825477394,0.,-0.669130606358858));
#34624=DIRECTION('ref_axis',(-0.669130606358858,0.,0.743144825477394));
#34625=DIRECTION('',(-0.669130606358858,0.,0.743144825477394));
#34626=DIRECTION('center_axis',(0.,1.,0.));
#34627=DIRECTION('ref_axis',(0.743144825477394,0.,0.669130606358858));
#34628=DIRECTION('center_axis',(-0.587785252292473,0.,-0.809016994374947));
#34629=DIRECTION('ref_axis',(0.809016994374947,0.,-0.587785252292473));
#34630=DIRECTION('',(0.,-1.,0.));
#34631=DIRECTION('',(0.809016994374947,0.,-0.587785252292473));
#34632=DIRECTION('center_axis',(0.,-1.,0.));
#34633=DIRECTION('ref_axis',(-0.587785252292473,0.,-0.809016994374947));
#34634=DIRECTION('',(-0.587785252292473,0.,-0.809016994374947));
#34635=DIRECTION('',(-0.809016994374947,0.,0.587785252292473));
#34636=DIRECTION('center_axis',(-0.809016994374947,0.,0.587785252292473));
#34637=DIRECTION('ref_axis',(-0.587785252292473,0.,-0.809016994374947));
#34638=DIRECTION('',(0.,-1.,0.));
#34639=DIRECTION('center_axis',(0.587785252292473,0.,0.809016994374947));
#34640=DIRECTION('ref_axis',(-0.809016994374947,0.,0.587785252292473));
#34641=DIRECTION('center_axis',(-0.809016994374947,0.,0.587785252292473));
#34642=DIRECTION('ref_axis',(0.587785252292473,0.,0.809016994374947));
#34643=DIRECTION('',(0.,1.,0.));
#34644=DIRECTION('',(0.587785252292473,0.,0.809016994374947));
#34645=DIRECTION('',(0.,1.,0.));
#34646=DIRECTION('center_axis',(-0.587785252292473,0.,-0.809016994374947));
#34647=DIRECTION('ref_axis',(-0.809016994374947,0.,0.587785252292473));
#34648=DIRECTION('',(-0.809016994374947,0.,0.587785252292473));
#34649=DIRECTION('center_axis',(0.587785252292473,0.,0.809016994374947));
#34650=DIRECTION('ref_axis',(0.809016994374947,0.,-0.587785252292473));
#34651=DIRECTION('',(0.809016994374947,0.,-0.587785252292473));
#34652=DIRECTION('center_axis',(0.,1.,0.));
#34653=DIRECTION('ref_axis',(0.587785252292473,0.,0.809016994374947));
#34654=DIRECTION('center_axis',(-0.4067366430758,0.,-0.913545457642601));
#34655=DIRECTION('ref_axis',(0.913545457642601,0.,-0.4067366430758));
#34656=DIRECTION('',(0.,-1.,0.));
#34657=DIRECTION('',(0.913545457642601,0.,-0.4067366430758));
#34658=DIRECTION('center_axis',(0.,-1.,0.));
#34659=DIRECTION('ref_axis',(-0.4067366430758,0.,-0.913545457642601));
#34660=DIRECTION('',(-0.4067366430758,0.,-0.913545457642601));
#34661=DIRECTION('',(-0.913545457642601,0.,0.4067366430758));
#34662=DIRECTION('center_axis',(-0.913545457642601,0.,0.4067366430758));
#34663=DIRECTION('ref_axis',(-0.4067366430758,0.,-0.913545457642601));
#34664=DIRECTION('',(0.,-1.,0.));
#34665=DIRECTION('center_axis',(0.4067366430758,0.,0.913545457642601));
#34666=DIRECTION('ref_axis',(-0.913545457642601,0.,0.4067366430758));
#34667=DIRECTION('center_axis',(-0.4067366430758,0.,-0.913545457642601));
#34668=DIRECTION('ref_axis',(-0.913545457642601,0.,0.4067366430758));
#34669=DIRECTION('',(-0.913545457642601,0.,0.4067366430758));
#34670=DIRECTION('center_axis',(0.,1.,0.));
#34671=DIRECTION('ref_axis',(0.4067366430758,0.,0.913545457642601));
#34672=DIRECTION('center_axis',(-0.207911690817759,0.,-0.978147600733806));
#34673=DIRECTION('ref_axis',(0.978147600733806,0.,-0.207911690817759));
#34674=DIRECTION('',(0.,-1.,0.));
#34675=DIRECTION('',(0.978147600733806,0.,-0.207911690817759));
#34676=DIRECTION('center_axis',(0.,-1.,0.));
#34677=DIRECTION('ref_axis',(-0.207911690817759,0.,-0.978147600733806));
#34678=DIRECTION('',(-0.207911690817759,0.,-0.978147600733806));
#34679=DIRECTION('',(-0.978147600733806,0.,0.207911690817759));
#34680=DIRECTION('center_axis',(-0.978147600733806,0.,0.207911690817759));
#34681=DIRECTION('ref_axis',(-0.207911690817759,0.,-0.978147600733806));
#34682=DIRECTION('',(0.,-1.,0.));
#34683=DIRECTION('center_axis',(0.207911690817759,0.,0.978147600733806));
#34684=DIRECTION('ref_axis',(-0.978147600733806,0.,0.207911690817759));
#34685=DIRECTION('center_axis',(-0.978147600733806,0.,0.207911690817759));
#34686=DIRECTION('ref_axis',(0.207911690817759,0.,0.978147600733806));
#34687=DIRECTION('',(0.,1.,0.));
#34688=DIRECTION('',(0.207911690817759,0.,0.978147600733806));
#34689=DIRECTION('',(0.,1.,0.));
#34690=DIRECTION('center_axis',(-0.207911690817759,0.,-0.978147600733806));
#34691=DIRECTION('ref_axis',(-0.978147600733806,0.,0.207911690817759));
#34692=DIRECTION('',(-0.978147600733806,0.,0.207911690817759));
#34693=DIRECTION('center_axis',(0.207911690817759,0.,0.978147600733806));
#34694=DIRECTION('ref_axis',(0.978147600733806,0.,-0.207911690817759));
#34695=DIRECTION('',(0.978147600733806,0.,-0.207911690817759));
#34696=DIRECTION('center_axis',(0.,1.,0.));
#34697=DIRECTION('ref_axis',(0.207911690817759,0.,0.978147600733806));
#34698=DIRECTION('center_axis',(0.,0.,-1.));
#34699=DIRECTION('ref_axis',(1.,0.,0.));
#34700=DIRECTION('',(0.,-1.,0.));
#34701=DIRECTION('',(1.,0.,0.));
#34702=DIRECTION('center_axis',(0.,-1.,0.));
#34703=DIRECTION('ref_axis',(0.,0.,-1.));
#34704=DIRECTION('',(0.,0.,-1.));
#34705=DIRECTION('',(-1.,0.,0.));
#34706=DIRECTION('center_axis',(-1.,0.,0.));
#34707=DIRECTION('ref_axis',(0.,0.,-1.));
#34708=DIRECTION('',(0.,-1.,0.));
#34709=DIRECTION('center_axis',(0.,0.,1.));
#34710=DIRECTION('ref_axis',(-1.,0.,0.));
#34711=DIRECTION('center_axis',(0.,1.,0.));
#34712=DIRECTION('ref_axis',(0.,0.,1.));
#34713=DIRECTION('',(1.,0.,0.));
#34714=DIRECTION('',(0.,0.,1.));
#34715=DIRECTION('',(-1.,0.,0.));
#34716=DIRECTION('center_axis',(0.,0.,-1.));
#34717=DIRECTION('ref_axis',(-1.,0.,0.));
#34718=DIRECTION('',(0.,1.,0.));
#34719=DIRECTION('center_axis',(-1.,0.,0.));
#34720=DIRECTION('ref_axis',(0.,0.,1.));
#34721=DIRECTION('',(0.,1.,0.));
#34722=DIRECTION('center_axis',(0.,0.,1.));
#34723=DIRECTION('ref_axis',(1.,0.,0.));
#34724=DIRECTION('center_axis',(0.,1.,0.));
#34725=DIRECTION('ref_axis',(-1.22464679914735E-16,0.,-1.));
#42565=CARTESIAN_POINT('',(0.,0.,0.));
#42566=CARTESIAN_POINT('Origin',(-11.5124520292426,4.75,-29.3401518343476));
#42567=CARTESIAN_POINT('',(-30.6706202195582,4.95,-62.9230725199241));
#42568=CARTESIAN_POINT('',(-31.0304893797597,4.55,-62.7463841894704));
#42569=CARTESIAN_POINT('Origin',(0.,0.0499999999999893,0.));
#42570=CARTESIAN_POINT('',(-24.60288568297,4.55,-51.613448015713));
#42571=CARTESIAN_POINT('',(-11.6856571099995,4.55,-29.2401518343476));
#42572=CARTESIAN_POINT('',(-24.0564755214562,4.95,-51.4670378541992));
#42573=CARTESIAN_POINT('',(-19.6210007919903,8.19699285765687,-50.2785559823902));
#42574=CARTESIAN_POINT('',(-11.3392469484857,4.95,-29.4401518343476));
#42575=CARTESIAN_POINT('Origin',(-31.60288568297,4.95,-63.7378036686952));
#42576=CARTESIAN_POINT('',(-31.0304893797597,0.75,-62.7463841894704));
#42577=CARTESIAN_POINT('',(-31.0304893797597,0.,-62.7463841894704));
#42578=CARTESIAN_POINT('',(-24.60288568297,0.75,-51.613448015713));
#42579=CARTESIAN_POINT('',(-31.60288568297,0.75,-63.7378036686952));
#42580=CARTESIAN_POINT('',(-24.60288568297,4.95,-51.613448015713));
#42581=CARTESIAN_POINT('Origin',(0.,0.,0.));
#42582=CARTESIAN_POINT('',(-26.2383050414052,4.95,-64.8964663795662));
#42583=CARTESIAN_POINT('Origin',(0.,4.95,0.));
#42584=CARTESIAN_POINT('',(-25.8662005535307,4.55,-65.0456737141259));
#42585=CARTESIAN_POINT('Origin',(0.,0.0499999999999791,0.));
#42586=CARTESIAN_POINT('',(-25.8662005535307,0.75,-65.0456737141259));
#42587=CARTESIAN_POINT('',(-25.8662005535307,0.,-65.0456737141259));
#42588=CARTESIAN_POINT('',(-17.3066919068743,0.75,-67.8268266635004));
#42589=CARTESIAN_POINT('Origin',(0.,0.75,0.));
#42590=CARTESIAN_POINT('',(-17.3066919068743,4.55,-67.8268266635004));
#42591=CARTESIAN_POINT('',(-17.3066919068743,0.,-67.8268266635004));
#42592=CARTESIAN_POINT('',(-16.9179511817127,4.95,-67.9248329244407));
#42593=CARTESIAN_POINT('Origin',(0.,0.0500000000000549,0.));
#42594=CARTESIAN_POINT('',(-12.1722010704987,4.95,-68.9335732506255));
#42595=CARTESIAN_POINT('Origin',(0.,4.95,0.));
#42596=CARTESIAN_POINT('',(-11.7772060092513,4.55,-69.0021551737021));
#42597=CARTESIAN_POINT('Origin',(0.,0.0500000000000049,0.));
#42598=CARTESIAN_POINT('',(-11.7772060092513,0.75,-69.0021551737021));
#42599=CARTESIAN_POINT('',(-11.7772060092513,0.,-69.0021551737021));
#42600=CARTESIAN_POINT('',(-2.82650895093685,0.75,-69.9429113431109));
#42601=CARTESIAN_POINT('Origin',(0.,0.75,0.));
#42602=CARTESIAN_POINT('',(-2.82650895093685,4.55,-69.9429113431109));
#42603=CARTESIAN_POINT('',(-2.82650895093685,0.,-69.9429113431109));
#42604=CARTESIAN_POINT('',(-2.42588649588962,4.95,-69.9579521906485));
#42605=CARTESIAN_POINT('Origin',(0.,0.0499999999999979,0.));
#42606=CARTESIAN_POINT('',(-8.57252759403147E-15,4.95000000000004,-70.));
#42607=CARTESIAN_POINT('Origin',(0.,4.95,0.));
#42608=CARTESIAN_POINT('',(-8.57252759403147E-15,-4.95000000000002,-70.));
#42609=CARTESIAN_POINT('',(-8.57252759403147E-15,0.,-70.));
#42610=CARTESIAN_POINT('',(-2.42588649588962,-4.95,-69.9579521906485));
#42611=CARTESIAN_POINT('Origin',(0.,-4.95,0.));
#42612=CARTESIAN_POINT('',(-2.82650895093685,-4.55,-69.9429113431109));
#42613=CARTESIAN_POINT('Origin',(0.,-0.0500000000000168,0.));
#42614=CARTESIAN_POINT('',(-2.82650895093685,-0.75,-69.9429113431109));
#42615=CARTESIAN_POINT('',(-2.82650895093685,0.,-69.9429113431109));
#42616=CARTESIAN_POINT('',(-11.7772060092513,-0.75,-69.0021551737021));
#42617=CARTESIAN_POINT('Origin',(0.,-0.75,0.));
#42618=CARTESIAN_POINT('',(-11.7772060092513,-4.55,-69.0021551737021));
#42619=CARTESIAN_POINT('',(-11.7772060092513,0.,-69.0021551737021));
#42620=CARTESIAN_POINT('',(-12.1722010704987,-4.95,-68.9335732506255));
#42621=CARTESIAN_POINT('Origin',(0.,-0.0499999999999852,0.));
#42622=CARTESIAN_POINT('',(-16.9179511817127,-4.95,-67.9248329244407));
#42623=CARTESIAN_POINT('Origin',(0.,-4.95,0.));
#42624=CARTESIAN_POINT('',(-17.3066919068743,-4.55,-67.8268266635004));
#42625=CARTESIAN_POINT('Origin',(0.,-0.0500000000000244,0.));
#42626=CARTESIAN_POINT('',(-17.3066919068743,-0.75,-67.8268266635004));
#42627=CARTESIAN_POINT('',(-17.3066919068743,0.,-67.8268266635004));
#42628=CARTESIAN_POINT('',(-25.8662005535307,-0.75,-65.0456737141259));
#42629=CARTESIAN_POINT('Origin',(0.,-0.75,0.));
#42630=CARTESIAN_POINT('',(-25.8662005535307,-4.55,-65.0456737141259));
#42631=CARTESIAN_POINT('',(-25.8662005535307,0.,-65.0456737141259));
#42632=CARTESIAN_POINT('',(-26.2383050414052,-4.95,-64.8964663795662));
#42633=CARTESIAN_POINT('Origin',(0.,-0.0500000000000249,0.));
#42634=CARTESIAN_POINT('',(-30.6706202195582,-4.95,-62.9230725199241));
#42635=CARTESIAN_POINT('Origin',(0.,-4.95,0.));
#42636=CARTESIAN_POINT('',(-31.0304893797597,-4.55,-62.7463841894704));
#42637=CARTESIAN_POINT('Origin',(0.,-0.0500000000000491,0.));
#42638=CARTESIAN_POINT('',(-31.0304893797597,-0.75,-62.7463841894704));
#42639=CARTESIAN_POINT('',(-31.0304893797597,0.,-62.7463841894704));
#42640=CARTESIAN_POINT('',(-38.8247180138197,-0.75,-58.2463841894704));
#42641=CARTESIAN_POINT('Origin',(0.,-0.75,0.));
#42642=CARTESIAN_POINT('',(-38.8247180138197,-4.55,-58.2463841894704));
#42643=CARTESIAN_POINT('',(-38.8247180138197,0.,-58.2463841894704));
#42644=CARTESIAN_POINT('',(-39.1576691766457,-4.95,-58.0230725199241));
#42645=CARTESIAN_POINT('Origin',(0.,-0.0500000000000088,0.));
#42646=CARTESIAN_POINT('',(-43.0828359798445,-4.95,-55.1712719078853));
#42647=CARTESIAN_POINT('Origin',(0.,-4.95,0.));
#42648=CARTESIAN_POINT('',(-43.3981055659413,-4.55,-54.9236236358037));
#42649=CARTESIAN_POINT('Origin',(0.,-0.0499999999998519,0.));
#42650=CARTESIAN_POINT('',(-43.3981055659413,-0.75,-54.9236236358037));
#42651=CARTESIAN_POINT('',(-43.3981055659413,0.,-54.9236236358037));
#42652=CARTESIAN_POINT('',(-50.0864089952379,-0.75,-48.901448178574));
#42653=CARTESIAN_POINT('Origin',(0.,-0.75,0.));
#42654=CARTESIAN_POINT('',(-50.0864089952379,-4.55,-48.901448178574));
#42655=CARTESIAN_POINT('',(-50.0864089952379,0.,-48.901448178574));
#42656=CARTESIAN_POINT('',(-50.3656552695229,-4.95,-48.6137919655685));
#42657=CARTESIAN_POINT('Origin',(0.,-0.0499999999999022,0.));
#42658=CARTESIAN_POINT('',(-53.6121250734278,-4.95,-45.0082219723368));
#42659=CARTESIAN_POINT('Origin',(0.,-4.95,0.));
#42660=CARTESIAN_POINT('',(-53.8690162916761,-4.55,-44.7004371764654));
#42661=CARTESIAN_POINT('Origin',(0.,-0.0499999999999979,0.));
#42662=CARTESIAN_POINT('',(-53.8690162916761,-0.75,-44.7004371764654));
#42663=CARTESIAN_POINT('',(-53.8690162916761,0.,-44.7004371764654));
#42664=CARTESIAN_POINT('',(-59.1590835623084,-0.75,-37.4192842270909));
#42665=CARTESIAN_POINT('Origin',(0.,-0.75,0.));
#42666=CARTESIAN_POINT('',(-59.1590835623084,-4.55,-37.4192842270909));
#42667=CARTESIAN_POINT('',(-59.1590835623084,0.,-37.4192842270909));
#42668=CARTESIAN_POINT('',(-59.372420545894,-4.95,-37.0798554274623));
#42669=CARTESIAN_POINT('Origin',(0.,-0.0500000000000306,0.));
#42670=CARTESIAN_POINT('',(-61.7983070417836,-4.95,-32.8780967631862));
#42671=CARTESIAN_POINT('Origin',(0.,-4.95,0.));
#42672=CARTESIAN_POINT('',(-61.9855925132453,-4.55,-32.5236271160201));
#42673=CARTESIAN_POINT('Origin',(0.,-0.0499999999998472,0.));
#42674=CARTESIAN_POINT('',(-61.9855925132453,-0.75,-32.5236271160201));
#42675=CARTESIAN_POINT('',(-61.9855925132453,0.,-32.5236271160201));
#42676=CARTESIAN_POINT('',(-65.6462223009275,-0.75,-24.3017179972367));
#42677=CARTESIAN_POINT('Origin',(0.,-0.75,0.));
#42678=CARTESIAN_POINT('',(-65.6462223009274,-4.55,-24.3017179972366));
#42679=CARTESIAN_POINT('',(-65.6462223009274,0.,-24.3017179972366));
#42680=CARTESIAN_POINT('',(-65.7843261439265,-4.95,-23.9253512782887));
#42681=CARTESIAN_POINT('Origin',(0.,-0.049999999999976,0.));
#42682=CARTESIAN_POINT('',(-67.2836064512356,-4.95,-19.3110409588722));
#42683=CARTESIAN_POINT('Origin',(0.,-4.95,0.));
#42684=CARTESIAN_POINT('',(-67.3931009021123,-4.55,-18.9253784849265));
#42685=CARTESIAN_POINT('Origin',(0.,-0.0500000000000752,0.));
#42686=CARTESIAN_POINT('',(-67.3931009021122,-0.75,-18.9253784849265));
#42687=CARTESIAN_POINT('',(-67.3931009021123,0.,-18.9253784849265));
#42688=CARTESIAN_POINT('',(-69.2643061194721,-0.75,-10.1220500783223));
#42689=CARTESIAN_POINT('Origin',(0.,-0.75,0.));
#42690=CARTESIAN_POINT('',(-69.2643061194721,-4.55,-10.1220500783223));
#42691=CARTESIAN_POINT('',(-69.2643061194721,0.,-10.1220500783223));
#42692=CARTESIAN_POINT('',(-69.3211410212497,-4.95,-9.72519447168095));
#42693=CARTESIAN_POINT('Origin',(0.,-0.0499999999999407,0.));
#42694=CARTESIAN_POINT('',(-69.8282893962039,-4.95,-4.90000000000001));
#42695=CARTESIAN_POINT('Origin',(0.,-4.95,0.));
#42696=CARTESIAN_POINT('',(-69.8552073935795,-4.55,-4.50000000000001));
#42697=CARTESIAN_POINT('Origin',(0.,-0.0500000000000236,0.));
#42698=CARTESIAN_POINT('',(-69.8552073935795,-0.75,-4.50000000000001));
#42699=CARTESIAN_POINT('',(-69.8552073935795,0.,-4.50000000000001));
#42700=CARTESIAN_POINT('',(-69.8552073935795,-0.75,4.49999999999999));
#42701=CARTESIAN_POINT('Origin',(0.,-0.75,0.));
#42702=CARTESIAN_POINT('',(-69.8552073935795,-4.55,4.49999999999999));
#42703=CARTESIAN_POINT('',(-69.8552073935795,0.,4.49999999999999));
#42704=CARTESIAN_POINT('',(-69.8282893962039,-4.95,4.89999999999999));
#42705=CARTESIAN_POINT('Origin',(0.,-0.0500000000000182,0.));
#42706=CARTESIAN_POINT('',(-69.3211410212497,-4.95,9.7251944716809));
#42707=CARTESIAN_POINT('Origin',(0.,-4.95,0.));
#42708=CARTESIAN_POINT('',(-69.2643061194721,-4.55,10.1220500783222));
#42709=CARTESIAN_POINT('Origin',(0.,-0.0500000000000127,0.));
#42710=CARTESIAN_POINT('',(-69.2643061194721,-0.75,10.1220500783222));
#42711=CARTESIAN_POINT('',(-69.2643061194721,0.,10.1220500783222));
#42712=CARTESIAN_POINT('',(-67.3931009021123,-0.75,18.9253784849265));
#42713=CARTESIAN_POINT('Origin',(0.,-0.75,0.));
#42714=CARTESIAN_POINT('',(-67.3931009021123,-4.55,18.9253784849265));
#42715=CARTESIAN_POINT('',(-67.3931009021123,0.,18.9253784849265));
#42716=CARTESIAN_POINT('',(-67.2836064512357,-4.95,19.3110409588722));
#42717=CARTESIAN_POINT('Origin',(0.,-0.0500000000000002,0.));
#42718=CARTESIAN_POINT('',(-65.7843261439265,-4.95,23.9253512782887));
#42719=CARTESIAN_POINT('Origin',(0.,-4.95,0.));
#42720=CARTESIAN_POINT('',(-65.6462223009275,-4.55,24.3017179972366));
#42721=CARTESIAN_POINT('Origin',(0.,-0.0500000000000877,0.));
#42722=CARTESIAN_POINT('',(-65.6462223009275,-0.75,24.3017179972366));
#42723=CARTESIAN_POINT('',(-65.6462223009275,0.,24.3017179972366));
#42724=CARTESIAN_POINT('',(-61.9855925132453,-0.75,32.52362711602));
#42725=CARTESIAN_POINT('Origin',(0.,-0.75,0.));
#42726=CARTESIAN_POINT('',(-61.9855925132453,-4.55,32.52362711602));
#42727=CARTESIAN_POINT('',(-61.9855925132453,0.,32.52362711602));
#42728=CARTESIAN_POINT('',(-61.7983070417837,-4.95,32.8780967631862));
#42729=CARTESIAN_POINT('Origin',(0.,-0.0500000000000174,0.));
#42730=CARTESIAN_POINT('',(-59.372420545894,-4.95,37.0798554274623));
#42731=CARTESIAN_POINT('Origin',(0.,-4.95,0.));
#42732=CARTESIAN_POINT('',(-59.1590835623084,-4.55,37.4192842270909));
#42733=CARTESIAN_POINT('Origin',(0.,-0.0500000000000454,0.));
#42734=CARTESIAN_POINT('',(-59.1590835623084,-0.75,37.4192842270909));
#42735=CARTESIAN_POINT('',(-59.1590835623084,0.,37.4192842270909));
#42736=CARTESIAN_POINT('',(-53.8690162916761,-0.75,44.7004371764654));
#42737=CARTESIAN_POINT('Origin',(0.,-0.75,0.));
#42738=CARTESIAN_POINT('',(-53.8690162916761,-4.55,44.7004371764654));
#42739=CARTESIAN_POINT('',(-53.8690162916761,0.,44.7004371764654));
#42740=CARTESIAN_POINT('',(-53.6121250734278,-4.95,45.0082219723368));
#42741=CARTESIAN_POINT('Origin',(0.,-0.0499999999999049,0.));
#42742=CARTESIAN_POINT('',(-50.365655269523,-4.95,48.6137919655685));
#42743=CARTESIAN_POINT('Origin',(0.,-4.95,0.));
#42744=CARTESIAN_POINT('',(-50.0864089952379,-4.55,48.9014481785739));
#42745=CARTESIAN_POINT('Origin',(0.,-0.0499999999999206,0.));
#42746=CARTESIAN_POINT('',(-50.0864089952379,-0.75,48.9014481785739));
#42747=CARTESIAN_POINT('',(-50.0864089952379,0.,48.9014481785739));
#42748=CARTESIAN_POINT('',(-43.3981055659414,-0.75,54.9236236358036));
#42749=CARTESIAN_POINT('Origin',(0.,-0.75,0.));
#42750=CARTESIAN_POINT('',(-43.3981055659414,-4.55,54.9236236358036));
#42751=CARTESIAN_POINT('',(-43.3981055659414,0.,54.9236236358036));
#42752=CARTESIAN_POINT('',(-43.0828359798445,-4.95,55.1712719078853));
#42753=CARTESIAN_POINT('Origin',(0.,-0.0499999999999237,0.));
#42754=CARTESIAN_POINT('',(-39.1576691766457,-4.95,58.0230725199241));
#42755=CARTESIAN_POINT('Origin',(0.,-4.95,0.));
#42756=CARTESIAN_POINT('',(-38.8247180138197,-4.55,58.2463841894704));
#42757=CARTESIAN_POINT('Origin',(0.,-0.0500000000000736,0.));
#42758=CARTESIAN_POINT('',(-38.8247180138197,-0.75,58.2463841894704));
#42759=CARTESIAN_POINT('',(-38.8247180138197,0.,58.2463841894704));
#42760=CARTESIAN_POINT('',(-31.0304893797598,-0.75,62.7463841894704));
#42761=CARTESIAN_POINT('Origin',(0.,-0.75,0.));
#42762=CARTESIAN_POINT('',(-31.0304893797598,-4.55,62.7463841894704));
#42763=CARTESIAN_POINT('',(-31.0304893797598,0.,62.7463841894704));
#42764=CARTESIAN_POINT('',(-30.6706202195582,-4.95,62.9230725199241));
#42765=CARTESIAN_POINT('Origin',(0.,-0.0500000000000798,0.));
#42766=CARTESIAN_POINT('',(-26.2383050414052,-4.95,64.8964663795662));
#42767=CARTESIAN_POINT('Origin',(0.,-4.95,0.));
#42768=CARTESIAN_POINT('',(-25.8662005535307,-4.55,65.0456737141259));
#42769=CARTESIAN_POINT('Origin',(0.,-0.0500000000000174,0.));
#42770=CARTESIAN_POINT('',(-25.8662005535307,-0.75,65.0456737141259));
#42771=CARTESIAN_POINT('',(-25.8662005535307,0.,65.0456737141259));
#42772=CARTESIAN_POINT('',(-17.3066919068743,-0.75,67.8268266635004));
#42773=CARTESIAN_POINT('Origin',(0.,-0.75,0.));
#42774=CARTESIAN_POINT('',(-17.3066919068744,-4.55,67.8268266635004));
#42775=CARTESIAN_POINT('',(-17.3066919068744,0.,67.8268266635004));
#42776=CARTESIAN_POINT('',(-16.9179511817127,-4.95,67.9248329244407));
#42777=CARTESIAN_POINT('Origin',(0.,-0.0500000000000237,0.));
#42778=CARTESIAN_POINT('',(-12.1722010704988,-4.95,68.9335732506255));
#42779=CARTESIAN_POINT('Origin',(0.,-4.95,0.));
#42780=CARTESIAN_POINT('',(-11.7772060092514,-4.55,69.002155173702));
#42781=CARTESIAN_POINT('Origin',(0.,-0.0499999999999869,0.));
#42782=CARTESIAN_POINT('',(-11.7772060092514,-0.75,69.002155173702));
#42783=CARTESIAN_POINT('',(-11.7772060092514,0.,69.002155173702));
#42784=CARTESIAN_POINT('',(-2.82650895093691,-0.75,69.9429113431109));
#42785=CARTESIAN_POINT('Origin',(0.,-0.75,0.));
#42786=CARTESIAN_POINT('',(-2.82650895093691,-4.55,69.9429113431109));
#42787=CARTESIAN_POINT('',(-2.82650895093691,0.,69.9429113431109));
#42788=CARTESIAN_POINT('',(-2.42588649588969,-4.95,69.9579521906485));
#42789=CARTESIAN_POINT('Origin',(0.,-0.0499999999999861,0.));
#42790=CARTESIAN_POINT('',(2.4258864958896,-4.95,69.9579521906485));
#42791=CARTESIAN_POINT('Origin',(0.,-4.95,0.));
#42792=CARTESIAN_POINT('',(2.82650895093682,-4.55,69.9429113431109));
#42793=CARTESIAN_POINT('Origin',(0.,-0.049999999999976,0.));
#42794=CARTESIAN_POINT('',(2.82650895093682,-0.75,69.9429113431109));
#42795=CARTESIAN_POINT('',(2.82650895093682,0.,69.9429113431109));
#42796=CARTESIAN_POINT('',(11.7772060092513,-0.75,69.0021551737021));
#42797=CARTESIAN_POINT('Origin',(0.,-0.75,0.));
#42798=CARTESIAN_POINT('',(11.7772060092513,-4.55,69.0021551737021));
#42799=CARTESIAN_POINT('',(11.7772060092513,0.,69.0021551737021));
#42800=CARTESIAN_POINT('',(12.1722010704987,-4.95,68.9335732506255));
#42801=CARTESIAN_POINT('Origin',(0.,-0.0499999999999893,0.));
#42802=CARTESIAN_POINT('',(16.9179511817127,-4.95,67.9248329244407));
#42803=CARTESIAN_POINT('Origin',(0.,-4.95,0.));
#42804=CARTESIAN_POINT('',(17.3066919068743,-4.55,67.8268266635004));
#42805=CARTESIAN_POINT('Origin',(0.,-0.0500000000000205,0.));
#42806=CARTESIAN_POINT('',(17.3066919068743,-0.75,67.8268266635004));
#42807=CARTESIAN_POINT('',(17.3066919068743,0.,67.8268266635004));
#42808=CARTESIAN_POINT('',(25.8662005535307,-0.75,65.0456737141259));
#42809=CARTESIAN_POINT('Origin',(0.,-0.75,0.));
#42810=CARTESIAN_POINT('',(25.8662005535307,-4.55,65.0456737141259));
#42811=CARTESIAN_POINT('',(25.8662005535307,0.,65.0456737141259));
#42812=CARTESIAN_POINT('',(26.2383050414052,-4.95,64.8964663795662));
#42813=CARTESIAN_POINT('Origin',(0.,-0.0499999999999705,0.));
#42814=CARTESIAN_POINT('',(30.6706202195581,-4.95,62.9230725199241));
#42815=CARTESIAN_POINT('Origin',(0.,-4.95,0.));
#42816=CARTESIAN_POINT('',(31.0304893797597,-4.55,62.7463841894704));
#42817=CARTESIAN_POINT('Origin',(0.,-0.0500000000000393,0.));
#42818=CARTESIAN_POINT('',(31.0304893797597,-0.75,62.7463841894704));
#42819=CARTESIAN_POINT('',(31.0304893797597,0.,62.7463841894704));
#42820=CARTESIAN_POINT('',(38.8247180138197,-0.75,58.2463841894704));
#42821=CARTESIAN_POINT('Origin',(0.,-0.75,0.));
#42822=CARTESIAN_POINT('',(38.8247180138197,-4.55,58.2463841894704));
#42823=CARTESIAN_POINT('',(38.8247180138197,0.,58.2463841894704));
#42824=CARTESIAN_POINT('',(39.1576691766456,-4.95,58.0230725199241));
#42825=CARTESIAN_POINT('Origin',(0.,-0.0499999999998987,0.));
#42826=CARTESIAN_POINT('',(43.0828359798445,-4.95,55.1712719078853));
#42827=CARTESIAN_POINT('Origin',(0.,-4.95,0.));
#42828=CARTESIAN_POINT('',(43.3981055659413,-4.55,54.9236236358037));
#42829=CARTESIAN_POINT('Origin',(0.,-0.0499999999999174,0.));
#42830=CARTESIAN_POINT('',(43.3981055659413,-0.75,54.9236236358037));
#42831=CARTESIAN_POINT('',(43.3981055659413,0.,54.9236236358037));
#42832=CARTESIAN_POINT('',(50.0864089952379,-0.75,48.901448178574));
#42833=CARTESIAN_POINT('Origin',(0.,-0.75,0.));
#42834=CARTESIAN_POINT('',(50.0864089952379,-4.55,48.901448178574));
#42835=CARTESIAN_POINT('',(50.0864089952379,0.,48.901448178574));
#42836=CARTESIAN_POINT('',(50.3656552695229,-4.95,48.6137919655685));
#42837=CARTESIAN_POINT('Origin',(0.,-0.0499999999999612,0.));
#42838=CARTESIAN_POINT('',(53.6121250734277,-4.95,45.0082219723368));
#42839=CARTESIAN_POINT('Origin',(0.,-4.95,0.));
#42840=CARTESIAN_POINT('',(53.8690162916761,-4.55,44.7004371764654));
#42841=CARTESIAN_POINT('Origin',(0.,-0.0500000000000486,0.));
#42842=CARTESIAN_POINT('',(53.8690162916761,-0.75,44.7004371764654));
#42843=CARTESIAN_POINT('',(53.8690162916761,0.,44.7004371764654));
#42844=CARTESIAN_POINT('',(59.1590835623084,-0.75,37.4192842270909));
#42845=CARTESIAN_POINT('Origin',(0.,-0.75,0.));
#42846=CARTESIAN_POINT('',(59.1590835623084,-4.55,37.4192842270909));
#42847=CARTESIAN_POINT('',(59.1590835623084,0.,37.4192842270909));
#42848=CARTESIAN_POINT('',(59.372420545894,-4.95,37.0798554274623));
#42849=CARTESIAN_POINT('Origin',(0.,-0.0500000000000174,0.));
#42850=CARTESIAN_POINT('',(61.7983070417836,-4.95,32.8780967631863));
#42851=CARTESIAN_POINT('Origin',(0.,-4.95,0.));
#42852=CARTESIAN_POINT('',(61.9855925132452,-4.55,32.5236271160201));
#42853=CARTESIAN_POINT('Origin',(0.,-0.0500000000001204,0.));
#42854=CARTESIAN_POINT('',(61.9855925132452,-0.75,32.5236271160201));
#42855=CARTESIAN_POINT('',(61.9855925132452,0.,32.5236271160201));
#42856=CARTESIAN_POINT('',(65.6462223009274,-0.75,24.3017179972367));
#42857=CARTESIAN_POINT('Origin',(0.,-0.75,0.));
#42858=CARTESIAN_POINT('',(65.6462223009274,-4.55,24.3017179972367));
#42859=CARTESIAN_POINT('',(65.6462223009274,0.,24.3017179972367));
#42860=CARTESIAN_POINT('',(65.7843261439265,-4.95,23.9253512782888));
#42861=CARTESIAN_POINT('Origin',(0.,-0.049999999999905,0.));
#42862=CARTESIAN_POINT('',(67.2836064512356,-4.95,19.3110409588723));
#42863=CARTESIAN_POINT('Origin',(0.,-4.95,0.));
#42864=CARTESIAN_POINT('',(67.3931009021122,-4.55,18.9253784849265));
#42865=CARTESIAN_POINT('Origin',(0.,-0.0500000000000127,0.));
#42866=CARTESIAN_POINT('',(67.3931009021122,-0.75,18.9253784849265));
#42867=CARTESIAN_POINT('',(67.3931009021122,0.,18.9253784849265));
#42868=CARTESIAN_POINT('',(69.2643061194721,-0.75,10.1220500783223));
#42869=CARTESIAN_POINT('Origin',(0.,-0.75,0.));
#42870=CARTESIAN_POINT('',(69.2643061194721,-4.55,10.1220500783223));
#42871=CARTESIAN_POINT('',(69.2643061194721,0.,10.1220500783223));
#42872=CARTESIAN_POINT('',(69.3211410212497,-4.95,9.72519447168096));
#42873=CARTESIAN_POINT('Origin',(0.,-0.0499999999999331,0.));
#42874=CARTESIAN_POINT('',(69.8282893962039,-4.95,4.9));
#42875=CARTESIAN_POINT('Origin',(0.,-4.95,0.));
#42876=CARTESIAN_POINT('',(69.8552073935795,-4.55,4.5));
#42877=CARTESIAN_POINT('Origin',(0.,-0.0500000000000182,0.));
#42878=CARTESIAN_POINT('',(69.8552073935795,-0.75,4.5));
#42879=CARTESIAN_POINT('',(69.8552073935795,0.,4.5));
#42880=CARTESIAN_POINT('',(69.8552073935795,-0.75,-4.5));
#42881=CARTESIAN_POINT('Origin',(0.,-0.75,0.));
#42882=CARTESIAN_POINT('',(69.8552073935795,-4.55,-4.5));
#42883=CARTESIAN_POINT('',(69.8552073935795,0.,-4.5));
#42884=CARTESIAN_POINT('',(69.8282893962039,-4.95,-4.9));
#42885=CARTESIAN_POINT('Origin',(0.,-0.0500000000000182,0.));
#42886=CARTESIAN_POINT('',(69.3211410212497,-4.95,-9.72519447168091));
#42887=CARTESIAN_POINT('Origin',(0.,-4.95,0.));
#42888=CARTESIAN_POINT('',(69.2643061194721,-4.55,-10.1220500783222));
#42889=CARTESIAN_POINT('Origin',(0.,-0.0500000000000287,0.));
#42890=CARTESIAN_POINT('',(69.2643061194721,-0.75,-10.1220500783222));
#42891=CARTESIAN_POINT('',(69.2643061194721,0.,-10.1220500783222));
#42892=CARTESIAN_POINT('',(67.3931009021123,-0.75,-18.9253784849265));
#42893=CARTESIAN_POINT('Origin',(0.,-0.75,0.));
#42894=CARTESIAN_POINT('',(67.3931009021123,-4.55,-18.9253784849265));
#42895=CARTESIAN_POINT('',(67.3931009021123,0.,-18.9253784849265));
#42896=CARTESIAN_POINT('',(67.2836064512357,-4.95,-19.3110409588722));
#42897=CARTESIAN_POINT('Origin',(0.,-0.0500000000000143,0.));
#42898=CARTESIAN_POINT('',(65.7843261439265,-4.95,-23.9253512782887));
#42899=CARTESIAN_POINT('Origin',(0.,-4.95,0.));
#42900=CARTESIAN_POINT('',(65.6462223009275,-4.55,-24.3017179972366));
#42901=CARTESIAN_POINT('Origin',(0.,-0.049999999999873,0.));
#42902=CARTESIAN_POINT('',(65.6462223009275,-0.75,-24.3017179972366));
#42903=CARTESIAN_POINT('',(65.6462223009275,0.,-24.3017179972366));
#42904=CARTESIAN_POINT('',(61.9855925132453,-0.75,-32.52362711602));
#42905=CARTESIAN_POINT('Origin',(0.,-0.75,0.));
#42906=CARTESIAN_POINT('',(61.9855925132453,-4.55,-32.52362711602));
#42907=CARTESIAN_POINT('',(61.9855925132453,0.,-32.52362711602));
#42908=CARTESIAN_POINT('',(61.7983070417836,-4.95,-32.8780967631862));
#42909=CARTESIAN_POINT('Origin',(0.,-0.0500000000002188,0.));
#42910=CARTESIAN_POINT('',(59.372420545894,-4.95,-37.0798554274623));
#42911=CARTESIAN_POINT('Origin',(0.,-4.95,0.));
#42912=CARTESIAN_POINT('',(59.1590835623084,-4.55,-37.4192842270909));
#42913=CARTESIAN_POINT('Origin',(0.,-0.0499999999999441,0.));
#42914=CARTESIAN_POINT('',(59.1590835623084,-0.75,-37.4192842270909));
#42915=CARTESIAN_POINT('',(59.1590835623084,0.,-37.4192842270909));
#42916=CARTESIAN_POINT('',(53.8690162916761,-0.75,-44.7004371764654));
#42917=CARTESIAN_POINT('Origin',(0.,-0.75,0.));
#42918=CARTESIAN_POINT('',(53.8690162916761,-4.55,-44.7004371764654));
#42919=CARTESIAN_POINT('',(53.8690162916761,0.,-44.7004371764654));
#42920=CARTESIAN_POINT('',(53.6121250734278,-4.95,-45.0082219723368));
#42921=CARTESIAN_POINT('Origin',(0.,-0.0500000000000424,0.));
#42922=CARTESIAN_POINT('',(50.365655269523,-4.95,-48.6137919655685));
#42923=CARTESIAN_POINT('Origin',(0.,-4.95,0.));
#42924=CARTESIAN_POINT('',(50.0864089952379,-4.55,-48.9014481785739));
#42925=CARTESIAN_POINT('Origin',(0.,-0.0499999999999559,0.));
#42926=CARTESIAN_POINT('',(50.0864089952379,-0.75,-48.9014481785739));
#42927=CARTESIAN_POINT('',(50.0864089952379,0.,-48.9014481785739));
#42928=CARTESIAN_POINT('',(43.3981055659414,-0.75,-54.9236236358037));
#42929=CARTESIAN_POINT('Origin',(0.,-0.75,0.));
#42930=CARTESIAN_POINT('',(43.3981055659414,-4.55,-54.9236236358037));
#42931=CARTESIAN_POINT('',(43.3981055659414,0.,-54.9236236358037));
#42932=CARTESIAN_POINT('',(43.0828359798445,-4.95,-55.1712719078853));
#42933=CARTESIAN_POINT('Origin',(0.,-0.050000000000197,0.));
#42934=CARTESIAN_POINT('',(39.1576691766457,-4.95,-58.0230725199241));
#42935=CARTESIAN_POINT('Origin',(0.,-4.95,0.));
#42936=CARTESIAN_POINT('',(38.8247180138197,-4.55,-58.2463841894704));
#42937=CARTESIAN_POINT('Origin',(0.,-0.0499999999998999,0.));
#42938=CARTESIAN_POINT('',(38.8247180138197,-0.75,-58.2463841894704));
#42939=CARTESIAN_POINT('',(38.8247180138197,0.,-58.2463841894704));
#42940=CARTESIAN_POINT('',(31.0304893797598,-0.75,-62.7463841894704));
#42941=CARTESIAN_POINT('Origin',(0.,-0.75,0.));
#42942=CARTESIAN_POINT('',(31.0304893797598,-4.55,-62.7463841894704));
#42943=CARTESIAN_POINT('',(31.0304893797598,0.,-62.7463841894704));
#42944=CARTESIAN_POINT('',(30.6706202195582,-4.95,-62.9230725199241));
#42945=CARTESIAN_POINT('Origin',(0.,-0.0499999999999463,0.));
#42946=CARTESIAN_POINT('',(26.2383050414052,-4.95,-64.8964663795662));
#42947=CARTESIAN_POINT('Origin',(0.,-4.95,0.));
#42948=CARTESIAN_POINT('',(25.8662005535307,-4.55,-65.0456737141259));
#42949=CARTESIAN_POINT('Origin',(0.,-0.0500000000000244,0.));
#42950=CARTESIAN_POINT('',(25.8662005535307,-0.75,-65.0456737141259));
#42951=CARTESIAN_POINT('',(25.8662005535307,0.,-65.0456737141259));
#42952=CARTESIAN_POINT('',(17.3066919068743,-0.75,-67.8268266635004));
#42953=CARTESIAN_POINT('Origin',(0.,-0.75,0.));
#42954=CARTESIAN_POINT('',(17.3066919068743,-4.55,-67.8268266635004));
#42955=CARTESIAN_POINT('',(17.3066919068743,0.,-67.8268266635004));
#42956=CARTESIAN_POINT('',(16.9179511817127,-4.95,-67.9248329244407));
#42957=CARTESIAN_POINT('Origin',(0.,-0.0499999999999975,0.));
#42958=CARTESIAN_POINT('',(12.1722010704987,-4.95,-68.9335732506255));
#42959=CARTESIAN_POINT('Origin',(0.,-4.95,0.));
#42960=CARTESIAN_POINT('',(11.7772060092513,-4.55,-69.002155173702));
#42961=CARTESIAN_POINT('Origin',(0.,-0.0499999999999915,0.));
#42962=CARTESIAN_POINT('',(11.7772060092513,-0.75,-69.002155173702));
#42963=CARTESIAN_POINT('',(11.7772060092513,0.,-69.002155173702));
#42964=CARTESIAN_POINT('',(2.82650895093687,-0.75,-69.9429113431109));
#42965=CARTESIAN_POINT('Origin',(0.,-0.75,0.));
#42966=CARTESIAN_POINT('',(2.82650895093687,-4.55,-69.9429113431109));
#42967=CARTESIAN_POINT('',(2.82650895093687,0.,-69.9429113431109));
#42968=CARTESIAN_POINT('',(2.42588649588965,-4.95,-69.9579521906485));
#42969=CARTESIAN_POINT('Origin',(0.,-0.0499999999999968,0.));
#42970=CARTESIAN_POINT('Origin',(0.,-4.95,0.));
#42971=CARTESIAN_POINT('',(2.42588649588965,4.95,-69.9579521906485));
#42972=CARTESIAN_POINT('Origin',(0.,4.95,0.));
#42973=CARTESIAN_POINT('',(2.82650895093687,4.55,-69.9429113431109));
#42974=CARTESIAN_POINT('Origin',(0.,0.0499999999999799,0.));
#42975=CARTESIAN_POINT('',(2.82650895093687,0.75,-69.9429113431109));
#42976=CARTESIAN_POINT('',(2.82650895093687,0.,-69.9429113431109));
#42977=CARTESIAN_POINT('',(11.7772060092513,0.75,-69.002155173702));
#42978=CARTESIAN_POINT('Origin',(0.,0.75,0.));
#42979=CARTESIAN_POINT('',(11.7772060092513,4.55,-69.002155173702));
#42980=CARTESIAN_POINT('',(11.7772060092513,0.,-69.002155173702));
#42981=CARTESIAN_POINT('',(12.1722010704987,4.95,-68.9335732506255));
#42982=CARTESIAN_POINT('Origin',(0.,0.0499999999999889,0.));
#42983=CARTESIAN_POINT('',(16.9179511817127,4.95,-67.9248329244407));
#42984=CARTESIAN_POINT('Origin',(0.,4.95,0.));
#42985=CARTESIAN_POINT('',(17.3066919068743,4.55,-67.8268266635004));
#42986=CARTESIAN_POINT('Origin',(0.,0.0499999999999752,0.));
#42987=CARTESIAN_POINT('',(17.3066919068743,0.75,-67.8268266635004));
#42988=CARTESIAN_POINT('',(17.3066919068743,0.,-67.8268266635004));
#42989=CARTESIAN_POINT('',(25.8662005535307,0.75,-65.0456737141259));
#42990=CARTESIAN_POINT('Origin',(0.,0.75,0.));
#42991=CARTESIAN_POINT('',(25.8662005535307,4.55,-65.0456737141259));
#42992=CARTESIAN_POINT('',(25.8662005535307,0.,-65.0456737141259));
#42993=CARTESIAN_POINT('',(26.2383050414052,4.95,-64.8964663795662));
#42994=CARTESIAN_POINT('Origin',(0.,0.0500000000000658,0.));
#42995=CARTESIAN_POINT('',(30.6706202195582,4.95,-62.9230725199241));
#42996=CARTESIAN_POINT('Origin',(0.,4.95,0.));
#42997=CARTESIAN_POINT('',(31.0304893797598,4.55,-62.7463841894704));
#42998=CARTESIAN_POINT('Origin',(0.,0.0499999999999612,0.));
#42999=CARTESIAN_POINT('',(31.0304893797598,0.75,-62.7463841894704));
#43000=CARTESIAN_POINT('',(31.0304893797598,0.,-62.7463841894704));
#43001=CARTESIAN_POINT('',(38.8247180138197,0.75,-58.2463841894704));
#43002=CARTESIAN_POINT('Origin',(0.,0.75,0.));
#43003=CARTESIAN_POINT('',(38.8247180138197,4.55,-58.2463841894704));
#43004=CARTESIAN_POINT('',(38.8247180138197,0.,-58.2463841894704));
#43005=CARTESIAN_POINT('',(39.1576691766457,4.95,-58.0230725199241));
#43006=CARTESIAN_POINT('Origin',(0.,0.0499999999999753,0.));
#43007=CARTESIAN_POINT('',(43.0828359798445,4.95,-55.1712719078853));
#43008=CARTESIAN_POINT('Origin',(0.,4.95,0.));
#43009=CARTESIAN_POINT('',(43.3981055659414,4.55,-54.9236236358037));
#43010=CARTESIAN_POINT('Origin',(0.,0.0499999999999174,0.));
#43011=CARTESIAN_POINT('',(43.3981055659414,0.75,-54.9236236358037));
#43012=CARTESIAN_POINT('',(43.3981055659414,0.,-54.9236236358037));
#43013=CARTESIAN_POINT('',(50.0864089952379,0.75,-48.9014481785739));
#43014=CARTESIAN_POINT('Origin',(0.,0.75,0.));
#43015=CARTESIAN_POINT('',(50.0864089952379,4.55,-48.9014481785739));
#43016=CARTESIAN_POINT('',(50.0864089952379,0.,-48.9014481785739));
#43017=CARTESIAN_POINT('',(50.365655269523,4.95,-48.6137919655685));
#43018=CARTESIAN_POINT('Origin',(0.,0.0499999999999987,0.));
#43019=CARTESIAN_POINT('',(53.6121250734278,4.95,-45.0082219723368));
#43020=CARTESIAN_POINT('Origin',(0.,4.95,0.));
#43021=CARTESIAN_POINT('',(53.8690162916761,4.55,-44.7004371764654));
#43022=CARTESIAN_POINT('Origin',(0.,0.0500000000000361,0.));
#43023=CARTESIAN_POINT('',(53.8690162916761,0.75,-44.7004371764654));
#43024=CARTESIAN_POINT('',(53.8690162916761,0.,-44.7004371764654));
#43025=CARTESIAN_POINT('',(59.1590835623084,0.75,-37.4192842270909));
#43026=CARTESIAN_POINT('Origin',(0.,0.75,0.));
#43027=CARTESIAN_POINT('',(59.1590835623084,4.55,-37.4192842270909));
#43028=CARTESIAN_POINT('',(59.1590835623084,0.,-37.4192842270909));
#43029=CARTESIAN_POINT('',(59.372420545894,4.95,-37.0798554274623));
#43030=CARTESIAN_POINT('Origin',(0.,0.0500000000000689,0.));
#43031=CARTESIAN_POINT('',(61.7983070417836,4.95,-32.8780967631862));
#43032=CARTESIAN_POINT('Origin',(0.,4.95,0.));
#43033=CARTESIAN_POINT('',(61.9855925132453,4.55,-32.52362711602));
#43034=CARTESIAN_POINT('Origin',(0.,0.0500000000000205,0.));
#43035=CARTESIAN_POINT('',(61.9855925132453,0.75,-32.52362711602));
#43036=CARTESIAN_POINT('',(61.9855925132453,0.,-32.52362711602));
#43037=CARTESIAN_POINT('',(65.6462223009275,0.75,-24.3017179972366));
#43038=CARTESIAN_POINT('Origin',(0.,0.75,0.));
#43039=CARTESIAN_POINT('',(65.6462223009275,4.55,-24.3017179972366));
#43040=CARTESIAN_POINT('',(65.6462223009275,0.,-24.3017179972366));
#43041=CARTESIAN_POINT('',(65.7843261439265,4.95,-23.9253512782887));
#43042=CARTESIAN_POINT('Origin',(0.,0.0500000000000158,0.));
#43043=CARTESIAN_POINT('',(67.2836064512357,4.95,-19.3110409588722));
#43044=CARTESIAN_POINT('Origin',(0.,4.95,0.));
#43045=CARTESIAN_POINT('',(67.3931009021123,4.55,-18.9253784849265));
#43046=CARTESIAN_POINT('Origin',(0.,0.0499999999999518,0.));
#43047=CARTESIAN_POINT('',(67.3931009021123,0.75,-18.9253784849265));
#43048=CARTESIAN_POINT('',(67.3931009021123,0.,-18.9253784849265));
#43049=CARTESIAN_POINT('',(69.2643061194721,0.75,-10.1220500783222));
#43050=CARTESIAN_POINT('Origin',(0.,0.75,0.));
#43051=CARTESIAN_POINT('',(69.2643061194721,4.55,-10.1220500783222));
#43052=CARTESIAN_POINT('',(69.2643061194721,0.,-10.1220500783222));
#43053=CARTESIAN_POINT('',(69.3211410212497,4.95,-9.72519447168092));
#43054=CARTESIAN_POINT('Origin',(0.,0.0499999999999783,0.));
#43055=CARTESIAN_POINT('',(69.8282893962039,4.95,-4.9));
#43056=CARTESIAN_POINT('Origin',(0.,4.95,0.));
#43057=CARTESIAN_POINT('',(69.8552073935795,4.55,-4.5));
#43058=CARTESIAN_POINT('Origin',(0.,0.0499999999999932,0.));
#43059=CARTESIAN_POINT('',(69.8552073935795,0.75,-4.5));
#43060=CARTESIAN_POINT('',(69.8552073935795,0.,-4.5));
#43061=CARTESIAN_POINT('',(69.8552073935795,0.75,4.5));
#43062=CARTESIAN_POINT('Origin',(0.,0.75,0.));
#43063=CARTESIAN_POINT('',(69.8552073935795,4.55,4.5));
#43064=CARTESIAN_POINT('',(69.8552073935795,0.,4.5));
#43065=CARTESIAN_POINT('',(69.8282893962039,4.95,4.9));
#43066=CARTESIAN_POINT('Origin',(0.,0.0499999999999932,0.));
#43067=CARTESIAN_POINT('',(69.3211410212497,4.95,9.72519447168096));
#43068=CARTESIAN_POINT('Origin',(0.,4.95,0.));
#43069=CARTESIAN_POINT('',(69.2643061194721,4.55,10.1220500783223));
#43070=CARTESIAN_POINT('Origin',(0.,0.0499999999999797,0.));
#43071=CARTESIAN_POINT('',(69.2643061194721,0.75,10.1220500783223));
#43072=CARTESIAN_POINT('',(69.2643061194721,0.,10.1220500783223));
#43073=CARTESIAN_POINT('',(67.3931009021122,0.75,18.9253784849265));
#43074=CARTESIAN_POINT('Origin',(0.,0.75,0.));
#43075=CARTESIAN_POINT('',(67.3931009021122,4.55,18.9253784849265));
#43076=CARTESIAN_POINT('',(67.3931009021122,0.,18.9253784849265));
#43077=CARTESIAN_POINT('',(67.2836064512356,4.95,19.3110409588723));
#43078=CARTESIAN_POINT('Origin',(0.,0.0499999999999877,0.));
#43079=CARTESIAN_POINT('',(65.7843261439265,4.95,23.9253512782888));
#43080=CARTESIAN_POINT('Origin',(0.,4.95,0.));
#43081=CARTESIAN_POINT('',(65.6462223009274,4.55,24.3017179972367));
#43082=CARTESIAN_POINT('Origin',(0.,0.0499999999999846,0.));
#43083=CARTESIAN_POINT('',(65.6462223009274,0.75,24.3017179972367));
#43084=CARTESIAN_POINT('',(65.6462223009274,0.,24.3017179972367));
#43085=CARTESIAN_POINT('',(61.9855925132452,0.75,32.5236271160201));
#43086=CARTESIAN_POINT('Origin',(0.,0.75,0.));
#43087=CARTESIAN_POINT('',(61.9855925132452,4.55,32.5236271160201));
#43088=CARTESIAN_POINT('',(61.9855925132452,0.,32.5236271160201));
#43089=CARTESIAN_POINT('',(61.7983070417836,4.95,32.8780967631863));
#43090=CARTESIAN_POINT('Origin',(0.,0.0500000000000143,0.));
#43091=CARTESIAN_POINT('',(59.372420545894,4.95,37.0798554274623));
#43092=CARTESIAN_POINT('Origin',(0.,4.95,0.));
#43093=CARTESIAN_POINT('',(59.1590835623084,4.55,37.4192842270909));
#43094=CARTESIAN_POINT('Origin',(0.,0.0500000000000002,0.));
#43095=CARTESIAN_POINT('',(59.1590835623084,0.75,37.4192842270909));
#43096=CARTESIAN_POINT('',(59.1590835623084,0.,37.4192842270909));
#43097=CARTESIAN_POINT('',(53.8690162916761,0.75,44.7004371764654));
#43098=CARTESIAN_POINT('Origin',(0.,0.75,0.));
#43099=CARTESIAN_POINT('',(53.8690162916761,4.55,44.7004371764654));
#43100=CARTESIAN_POINT('',(53.8690162916761,0.,44.7004371764654));
#43101=CARTESIAN_POINT('',(53.6121250734277,4.95,45.0082219723368));
#43102=CARTESIAN_POINT('Origin',(0.,0.0499999999999736,0.));
#43103=CARTESIAN_POINT('',(50.3656552695229,4.95,48.6137919655685));
#43104=CARTESIAN_POINT('Origin',(0.,4.95,0.));
#43105=CARTESIAN_POINT('',(50.0864089952379,4.55,48.901448178574));
#43106=CARTESIAN_POINT('Origin',(0.,0.0499999999999143,0.));
#43107=CARTESIAN_POINT('',(50.0864089952379,0.75,48.901448178574));
#43108=CARTESIAN_POINT('',(50.0864089952379,0.,48.901448178574));
#43109=CARTESIAN_POINT('',(43.3981055659413,0.75,54.9236236358037));
#43110=CARTESIAN_POINT('Origin',(0.,0.75,0.));
#43111=CARTESIAN_POINT('',(43.3981055659413,4.55,54.9236236358037));
#43112=CARTESIAN_POINT('',(43.3981055659413,0.,54.9236236358037));
#43113=CARTESIAN_POINT('',(43.0828359798445,4.95,55.1712719078853));
#43114=CARTESIAN_POINT('Origin',(0.,0.0499999999999924,0.));
#43115=CARTESIAN_POINT('',(39.1576691766456,4.95,58.0230725199241));
#43116=CARTESIAN_POINT('Origin',(0.,4.95,0.));
#43117=CARTESIAN_POINT('',(38.8247180138197,4.55,58.2463841894704));
#43118=CARTESIAN_POINT('Origin',(0.,0.0499999999999674,0.));
#43119=CARTESIAN_POINT('',(38.8247180138197,0.75,58.2463841894704));
#43120=CARTESIAN_POINT('',(38.8247180138197,0.,58.2463841894704));
#43121=CARTESIAN_POINT('',(31.0304893797597,0.75,62.7463841894704));
#43122=CARTESIAN_POINT('Origin',(0.,0.75,0.));
#43123=CARTESIAN_POINT('',(31.0304893797597,4.55,62.7463841894704));
#43124=CARTESIAN_POINT('',(31.0304893797597,0.,62.7463841894704));
#43125=CARTESIAN_POINT('',(30.6706202195581,4.95,62.9230725199241));
#43126=CARTESIAN_POINT('Origin',(0.,0.0499999999999924,0.));
#43127=CARTESIAN_POINT('',(26.2383050414052,4.95,64.8964663795662));
#43128=CARTESIAN_POINT('Origin',(0.,4.95,0.));
#43129=CARTESIAN_POINT('',(25.8662005535307,4.55,65.0456737141259));
#43130=CARTESIAN_POINT('Origin',(0.,0.0500000000000315,0.));
#43131=CARTESIAN_POINT('',(25.8662005535307,0.75,65.0456737141259));
#43132=CARTESIAN_POINT('',(25.8662005535307,0.,65.0456737141259));
#43133=CARTESIAN_POINT('',(17.3066919068743,0.75,67.8268266635004));
#43134=CARTESIAN_POINT('Origin',(0.,0.75,0.));
#43135=CARTESIAN_POINT('',(17.3066919068743,4.55,67.8268266635004));
#43136=CARTESIAN_POINT('',(17.3066919068743,0.,67.8268266635004));
#43137=CARTESIAN_POINT('',(16.9179511817127,4.95,67.9248329244407));
#43138=CARTESIAN_POINT('Origin',(0.,0.0500000000000018,0.));
#43139=CARTESIAN_POINT('',(12.1722010704987,4.95,68.9335732506255));
#43140=CARTESIAN_POINT('Origin',(0.,4.95,0.));
#43141=CARTESIAN_POINT('',(11.7772060092513,4.55,69.0021551737021));
#43142=CARTESIAN_POINT('Origin',(0.,0.0499999999999881,0.));
#43143=CARTESIAN_POINT('',(11.7772060092513,0.75,69.0021551737021));
#43144=CARTESIAN_POINT('',(11.7772060092513,0.,69.0021551737021));
#43145=CARTESIAN_POINT('',(2.82650895093682,0.75,69.9429113431109));
#43146=CARTESIAN_POINT('Origin',(0.,0.75,0.));
#43147=CARTESIAN_POINT('',(2.82650895093682,4.55,69.9429113431109));
#43148=CARTESIAN_POINT('',(2.82650895093682,0.,69.9429113431109));
#43149=CARTESIAN_POINT('',(2.4258864958896,4.95,69.9579521906485));
#43150=CARTESIAN_POINT('Origin',(0.,0.0499999999999979,0.));
#43151=CARTESIAN_POINT('',(-2.42588649588969,4.95,69.9579521906485));
#43152=CARTESIAN_POINT('Origin',(0.,4.95,0.));
#43153=CARTESIAN_POINT('',(-2.82650895093691,4.55,69.9429113431109));
#43154=CARTESIAN_POINT('Origin',(0.,0.0499999999999881,0.));
#43155=CARTESIAN_POINT('',(-2.82650895093691,0.75,69.9429113431109));
#43156=CARTESIAN_POINT('',(-2.82650895093691,0.,69.9429113431109));
#43157=CARTESIAN_POINT('',(-11.7772060092514,0.75,69.002155173702));
#43158=CARTESIAN_POINT('Origin',(0.,0.75,0.));
#43159=CARTESIAN_POINT('',(-11.7772060092514,4.55,69.002155173702));
#43160=CARTESIAN_POINT('',(-11.7772060092514,0.,69.002155173702));
#43161=CARTESIAN_POINT('',(-12.1722010704988,4.95,68.9335732506255));
#43162=CARTESIAN_POINT('Origin',(0.,0.0499999999999768,0.));
#43163=CARTESIAN_POINT('',(-16.9179511817127,4.95,67.9248329244407));
#43164=CARTESIAN_POINT('Origin',(0.,4.95,0.));
#43165=CARTESIAN_POINT('',(-17.3066919068743,4.55,67.8268266635004));
#43166=CARTESIAN_POINT('Origin',(0.,0.0500000000000018,0.));
#43167=CARTESIAN_POINT('',(-17.3066919068743,0.75,67.8268266635004));
#43168=CARTESIAN_POINT('',(-17.3066919068743,0.,67.8268266635004));
#43169=CARTESIAN_POINT('',(-25.8662005535307,0.75,65.0456737141259));
#43170=CARTESIAN_POINT('Origin',(0.,0.75,0.));
#43171=CARTESIAN_POINT('',(-25.8662005535307,4.55,65.0456737141259));
#43172=CARTESIAN_POINT('',(-25.8662005535307,0.,65.0456737141259));
#43173=CARTESIAN_POINT('',(-26.2383050414052,4.95,64.8964663795662));
#43174=CARTESIAN_POINT('Origin',(0.,0.0500000000000455,0.));
#43175=CARTESIAN_POINT('',(-30.6706202195582,4.95,62.9230725199241));
#43176=CARTESIAN_POINT('Origin',(0.,4.95,0.));
#43177=CARTESIAN_POINT('',(-31.0304893797598,4.55,62.7463841894704));
#43178=CARTESIAN_POINT('Origin',(0.,0.0499999999999643,0.));
#43179=CARTESIAN_POINT('',(-31.0304893797598,0.75,62.7463841894704));
#43180=CARTESIAN_POINT('',(-31.0304893797598,0.,62.7463841894704));
#43181=CARTESIAN_POINT('',(-38.8247180138197,0.75,58.2463841894704));
#43182=CARTESIAN_POINT('Origin',(0.,0.75,0.));
#43183=CARTESIAN_POINT('',(-38.8247180138197,4.55,58.2463841894704));
#43184=CARTESIAN_POINT('',(-38.8247180138197,0.,58.2463841894704));
#43185=CARTESIAN_POINT('',(-39.1576691766457,4.95,58.0230725199241));
#43186=CARTESIAN_POINT('Origin',(0.,0.0500000000000048,0.));
#43187=CARTESIAN_POINT('',(-43.0828359798445,4.95,55.1712719078853));
#43188=CARTESIAN_POINT('Origin',(0.,4.95,0.));
#43189=CARTESIAN_POINT('',(-43.3981055659414,4.55,54.9236236358036));
#43190=CARTESIAN_POINT('Origin',(0.,0.0499999999999487,0.));
#43191=CARTESIAN_POINT('',(-43.3981055659414,0.75,54.9236236358036));
#43192=CARTESIAN_POINT('',(-43.3981055659414,0.,54.9236236358036));
#43193=CARTESIAN_POINT('',(-50.0864089952379,0.75,48.9014481785739));
#43194=CARTESIAN_POINT('Origin',(0.,0.75,0.));
#43195=CARTESIAN_POINT('',(-50.0864089952379,4.55,48.9014481785739));
#43196=CARTESIAN_POINT('',(-50.0864089952379,0.,48.9014481785739));
#43197=CARTESIAN_POINT('',(-50.365655269523,4.95,48.6137919655685));
#43198=CARTESIAN_POINT('Origin',(0.,0.0499999999999987,0.));
#43199=CARTESIAN_POINT('',(-53.6121250734278,4.95,45.0082219723368));
#43200=CARTESIAN_POINT('Origin',(0.,4.95,0.));
#43201=CARTESIAN_POINT('',(-53.8690162916761,4.55,44.7004371764654));
#43202=CARTESIAN_POINT('Origin',(0.,0.0500000000000923,0.));
#43203=CARTESIAN_POINT('',(-53.8690162916761,0.75,44.7004371764654));
#43204=CARTESIAN_POINT('',(-53.8690162916761,0.,44.7004371764654));
#43205=CARTESIAN_POINT('',(-59.1590835623084,0.75,37.4192842270909));
#43206=CARTESIAN_POINT('Origin',(0.,0.75,0.));
#43207=CARTESIAN_POINT('',(-59.1590835623084,4.55,37.4192842270909));
#43208=CARTESIAN_POINT('',(-59.1590835623084,0.,37.4192842270909));
#43209=CARTESIAN_POINT('',(-59.372420545894,4.95,37.0798554274623));
#43210=CARTESIAN_POINT('Origin',(0.,0.0499999999999955,0.));
#43211=CARTESIAN_POINT('',(-61.7983070417837,4.95,32.8780967631862));
#43212=CARTESIAN_POINT('Origin',(0.,4.95,0.));
#43213=CARTESIAN_POINT('',(-61.9855925132453,4.55,32.52362711602));
#43214=CARTESIAN_POINT('Origin',(0.,0.0500000000000143,0.));
#43215=CARTESIAN_POINT('',(-61.9855925132453,0.75,32.52362711602));
#43216=CARTESIAN_POINT('',(-61.9855925132453,0.,32.52362711602));
#43217=CARTESIAN_POINT('',(-65.6462223009275,0.75,24.3017179972366));
#43218=CARTESIAN_POINT('Origin',(0.,0.75,0.));
#43219=CARTESIAN_POINT('',(-65.6462223009275,4.55,24.3017179972366));
#43220=CARTESIAN_POINT('',(-65.6462223009275,0.,24.3017179972366));
#43221=CARTESIAN_POINT('',(-65.7843261439265,4.95,23.9253512782887));
#43222=CARTESIAN_POINT('Origin',(0.,0.0500000000000877,0.));
#43223=CARTESIAN_POINT('',(-67.2836064512357,4.95,19.3110409588722));
#43224=CARTESIAN_POINT('Origin',(0.,4.95,0.));
#43225=CARTESIAN_POINT('',(-67.3931009021123,4.55,18.9253784849265));
#43226=CARTESIAN_POINT('Origin',(0.,0.0499999999999909,0.));
#43227=CARTESIAN_POINT('',(-67.3931009021123,0.75,18.9253784849265));
#43228=CARTESIAN_POINT('',(-67.3931009021123,0.,18.9253784849265));
#43229=CARTESIAN_POINT('',(-69.2643061194721,0.75,10.1220500783222));
#43230=CARTESIAN_POINT('Origin',(0.,0.75,0.));
#43231=CARTESIAN_POINT('',(-69.2643061194721,4.55,10.1220500783222));
#43232=CARTESIAN_POINT('',(-69.2643061194721,0.,10.1220500783222));
#43233=CARTESIAN_POINT('',(-69.3211410212497,4.95,9.7251944716809));
#43234=CARTESIAN_POINT('Origin',(0.,0.0499999999999944,0.));
#43235=CARTESIAN_POINT('',(-69.8282893962039,4.95,4.89999999999999));
#43236=CARTESIAN_POINT('Origin',(0.,4.95,0.));
#43237=CARTESIAN_POINT('',(-69.8552073935795,4.55,4.49999999999999));
#43238=CARTESIAN_POINT('Origin',(0.,0.0499999999999932,0.));
#43239=CARTESIAN_POINT('',(-69.8552073935795,0.75,4.49999999999999));
#43240=CARTESIAN_POINT('',(-69.8552073935795,0.,4.49999999999999));
#43241=CARTESIAN_POINT('',(-69.8552073935795,0.75,-4.50000000000001));
#43242=CARTESIAN_POINT('Origin',(0.,0.75,0.));
#43243=CARTESIAN_POINT('',(-69.8552073935795,4.55,-4.50000000000001));
#43244=CARTESIAN_POINT('',(-69.8552073935795,0.,-4.50000000000001));
#43245=CARTESIAN_POINT('',(-69.8282893962039,4.95,-4.90000000000001));
#43246=CARTESIAN_POINT('Origin',(0.,0.0499999999999932,0.));
#43247=CARTESIAN_POINT('',(-69.3211410212497,4.95,-9.72519447168095));
#43248=CARTESIAN_POINT('Origin',(0.,4.95,0.));
#43249=CARTESIAN_POINT('',(-69.2643061194721,4.55,-10.1220500783223));
#43250=CARTESIAN_POINT('Origin',(0.,0.0499999999999889,0.));
#43251=CARTESIAN_POINT('',(-69.2643061194721,0.75,-10.1220500783223));
#43252=CARTESIAN_POINT('',(-69.2643061194721,0.,-10.1220500783223));
#43253=CARTESIAN_POINT('',(-67.3931009021122,0.75,-18.9253784849265));
#43254=CARTESIAN_POINT('Origin',(0.,0.75,0.));
#43255=CARTESIAN_POINT('',(-67.3931009021122,4.55,-18.9253784849265));
#43256=CARTESIAN_POINT('',(-67.3931009021122,0.,-18.9253784849265));
#43257=CARTESIAN_POINT('',(-67.2836064512356,4.95,-19.3110409588722));
#43258=CARTESIAN_POINT('Origin',(0.,0.0500000000000143,0.));
#43259=CARTESIAN_POINT('',(-65.7843261439265,4.95,-23.9253512782887));
#43260=CARTESIAN_POINT('Origin',(0.,4.95,0.));
#43261=CARTESIAN_POINT('',(-65.6462223009274,4.55,-24.3017179972367));
#43262=CARTESIAN_POINT('Origin',(0.,0.0499999999999854,0.));
#43263=CARTESIAN_POINT('',(-65.6462223009275,0.75,-24.3017179972367));
#43264=CARTESIAN_POINT('',(-65.6462223009274,0.,-24.3017179972367));
#43265=CARTESIAN_POINT('',(-61.9855925132453,0.75,-32.5236271160201));
#43266=CARTESIAN_POINT('Origin',(0.,0.75,0.));
#43267=CARTESIAN_POINT('',(-61.9855925132453,4.55,-32.5236271160201));
#43268=CARTESIAN_POINT('',(-61.9855925132453,0.,-32.5236271160201));
#43269=CARTESIAN_POINT('',(-61.7983070417836,4.95,-32.8780967631862));
#43270=CARTESIAN_POINT('Origin',(0.,0.0499999999999737,0.));
#43271=CARTESIAN_POINT('',(-59.372420545894,4.95,-37.0798554274623));
#43272=CARTESIAN_POINT('Origin',(0.,4.95,0.));
#43273=CARTESIAN_POINT('',(-59.1590835623084,4.55,-37.4192842270909));
#43274=CARTESIAN_POINT('Origin',(0.,0.0499999999999986,0.));
#43275=CARTESIAN_POINT('',(-59.1590835623084,0.75,-37.4192842270909));
#43276=CARTESIAN_POINT('',(-59.1590835623084,0.,-37.4192842270909));
#43277=CARTESIAN_POINT('',(-53.8690162916761,0.75,-44.7004371764654));
#43278=CARTESIAN_POINT('Origin',(0.,0.75,0.));
#43279=CARTESIAN_POINT('',(-53.8690162916761,4.55,-44.7004371764654));
#43280=CARTESIAN_POINT('',(-53.8690162916761,0.,-44.7004371764654));
#43281=CARTESIAN_POINT('',(-53.6121250734277,4.95,-45.0082219723368));
#43282=CARTESIAN_POINT('Origin',(0.,0.0500000000000955,0.));
#43283=CARTESIAN_POINT('',(-50.3656552695229,4.95,-48.6137919655685));
#43284=CARTESIAN_POINT('Origin',(0.,4.95,0.));
#43285=CARTESIAN_POINT('',(-50.0864089952379,4.55,-48.901448178574));
#43286=CARTESIAN_POINT('Origin',(0.,0.0499999999999581,0.));
#43287=CARTESIAN_POINT('',(-50.0864089952379,0.75,-48.901448178574));
#43288=CARTESIAN_POINT('',(-50.0864089952379,0.,-48.901448178574));
#43289=CARTESIAN_POINT('',(-43.3981055659413,0.75,-54.9236236358037));
#43290=CARTESIAN_POINT('Origin',(0.,0.75,0.));
#43291=CARTESIAN_POINT('',(-43.3981055659413,4.55,-54.9236236358037));
#43292=CARTESIAN_POINT('',(-43.3981055659413,0.,-54.9236236358037));
#43293=CARTESIAN_POINT('',(-43.0828359798445,4.95,-55.1712719078853));
#43294=CARTESIAN_POINT('Origin',(0.,0.0499999999999987,0.));
#43295=CARTESIAN_POINT('',(-39.1576691766457,4.95,-58.0230725199241));
#43296=CARTESIAN_POINT('Origin',(0.,4.95,0.));
#43297=CARTESIAN_POINT('',(-38.8247180138197,4.55,-58.2463841894704));
#43298=CARTESIAN_POINT('Origin',(0.,0.0499999999999831,0.));
#43299=CARTESIAN_POINT('',(-38.8247180138197,0.75,-58.2463841894704));
#43300=CARTESIAN_POINT('',(-38.8247180138197,0.,-58.2463841894704));
#43301=CARTESIAN_POINT('Origin',(0.,0.75,0.));
#43302=CARTESIAN_POINT('Origin',(-11.8060173724113,4.75,-21.1256658124263));
#43303=CARTESIAN_POINT('',(-21.8937230027002,4.55,-52.8196449541365));
#43304=CARTESIAN_POINT('',(-11.6158060691523,4.55,-21.1874692113013));
#43305=CARTESIAN_POINT('',(-22.1505388114683,4.95,-52.3156155498685));
#43306=CARTESIAN_POINT('',(-11.9962286756703,4.95,-21.0638624135513));
#43307=CARTESIAN_POINT('',(-22.1505388114683,4.95,-52.3156155498685));
#43308=CARTESIAN_POINT('Origin',(-16.8832207126948,4.75,-54.2373633913317));
#43309=CARTESIAN_POINT('',(-12.8301849517758,4.95,-55.343982094743));
#43310=CARTESIAN_POINT('',(-16.8214173138198,4.95,-54.0471520880726));
#43311=CARTESIAN_POINT('',(-13.3342143560438,4.55,-55.600797903511));
#43312=CARTESIAN_POINT('',(-12.8301849517758,4.95,-55.343982094743));
#43313=CARTESIAN_POINT('',(-16.9450241115698,4.55,-54.4275746945907));
#43314=CARTESIAN_POINT('Origin',(-5.02920507986149,4.75,-30.6878211736169));
#43315=CARTESIAN_POINT('',(-4.83899377660246,4.95,-30.7496245724919));
#43316=CARTESIAN_POINT('',(-5.21941638312053,4.55,-30.6260177747419));
#43317=CARTESIAN_POINT('Origin',(-21.8937230027002,4.95,-52.8196449541365));
#43318=CARTESIAN_POINT('',(-21.8937230027002,0.75,-52.8196449541365));
#43319=CARTESIAN_POINT('',(-21.8937230027002,4.95,-52.8196449541365));
#43320=CARTESIAN_POINT('',(-21.8937230027002,0.75,-52.8196449541365));
#43321=CARTESIAN_POINT('Origin',(-13.3342143560438,4.95,-55.600797903511));
#43322=CARTESIAN_POINT('',(-13.3342143560438,0.75,-55.600797903511));
#43323=CARTESIAN_POINT('',(-13.3342143560438,4.95,-55.600797903511));
#43324=CARTESIAN_POINT('',(-13.3342143560438,0.75,-55.600797903511));
#43325=CARTESIAN_POINT('Origin',(-17.6604522772931,4.95,-68.9155891316432));
#43326=CARTESIAN_POINT('',(-17.6604522772931,0.75,-68.9155891316432));
#43327=CARTESIAN_POINT('Origin',(-7.13301510508756,4.75,-22.9022758698015));
#43328=CARTESIAN_POINT('',(-10.4334709354135,4.55,-56.2173699512871));
#43329=CARTESIAN_POINT('',(-6.93411072601391,4.55,-22.923181562455));
#43330=CARTESIAN_POINT('',(-10.7894683082537,4.95,-55.7777498078328));
#43331=CARTESIAN_POINT('',(-7.33191948416122,4.95,-22.881370177148));
#43332=CARTESIAN_POINT('',(-10.7894683082537,4.95,-55.7777498078328));
#43333=CARTESIAN_POINT('Origin',(-4.21984145529554,4.75,-56.6693470701065));
#43334=CARTESIAN_POINT('',(-1.04315373364464,4.95,-56.8021287478558));
#43335=CARTESIAN_POINT('',(-4.19893576264201,4.95,-56.4704426910328));
#43336=CARTESIAN_POINT('',(-1.48277387709901,4.55,-57.158126120696));
#43337=CARTESIAN_POINT('',(-1.04315373364464,4.95,-56.8021287478558));
#43338=CARTESIAN_POINT('',(-4.24074714794907,4.55,-56.8682514491801));
#43339=CARTESIAN_POINT('Origin',(1.48379146850063,4.75,-30.8464966920953));
#43340=CARTESIAN_POINT('',(1.68269584757429,4.95,-30.8674023847489));
#43341=CARTESIAN_POINT('',(1.28488708942698,4.55,-30.8255909994418));
#43342=CARTESIAN_POINT('Origin',(-10.4334709354135,4.95,-56.2173699512871));
#43343=CARTESIAN_POINT('',(-10.4334709354135,0.75,-56.2173699512871));
#43344=CARTESIAN_POINT('',(-10.4334709354135,4.95,-56.2173699512871));
#43345=CARTESIAN_POINT('',(-10.4334709354135,0.75,-56.2173699512871));
#43346=CARTESIAN_POINT('Origin',(-1.48277387709901,4.95,-57.158126120696));
#43347=CARTESIAN_POINT('',(-1.48277387709901,0.75,-57.158126120696));
#43348=CARTESIAN_POINT('',(-1.48277387709901,4.95,-57.158126120696));
#43349=CARTESIAN_POINT('',(-1.48277387709901,0.75,-57.158126120696));
#43350=CARTESIAN_POINT('Origin',(-2.94617236284616,4.95,-71.0814326558519));
#43351=CARTESIAN_POINT('',(-2.94617236284616,0.75,-71.0814326558519));
#43352=CARTESIAN_POINT('Origin',(-2.2154907113742,4.75,-23.8848434245174));
#43353=CARTESIAN_POINT('',(1.48277387709903,4.55,-57.158126120696));
#43354=CARTESIAN_POINT('',(-2.01658633230054,4.55,-23.8639377318639));
#43355=CARTESIAN_POINT('',(1.04315373364466,4.95,-56.8021287478558));
#43356=CARTESIAN_POINT('',(-2.41439509044785,4.95,-23.9057491171709));
#43357=CARTESIAN_POINT('',(1.04315373364466,4.95,-56.8021287478558));
#43358=CARTESIAN_POINT('Origin',(8.69518998445279,4.75,-56.198968985402));
#43359=CARTESIAN_POINT('',(10.7894683082537,4.95,-55.7777498078327));
#43360=CARTESIAN_POINT('',(8.67428429179926,4.95,-56.0000646063284));
#43361=CARTESIAN_POINT('',(10.4334709354135,4.55,-56.2173699512871));
#43362=CARTESIAN_POINT('',(10.7894683082537,4.95,-55.7777498078327));
#43363=CARTESIAN_POINT('',(8.71609567710632,4.55,-56.3978733644757));
#43364=CARTESIAN_POINT('Origin',(7.86471434796115,4.75,-29.8639291373794));
#43365=CARTESIAN_POINT('',(8.0636187270348,4.95,-29.8430234447259));
#43366=CARTESIAN_POINT('',(7.66580996888749,4.55,-29.8848348300329));
#43367=CARTESIAN_POINT('Origin',(1.48277387709903,4.95,-57.158126120696));
#43368=CARTESIAN_POINT('',(1.48277387709903,0.75,-57.158126120696));
#43369=CARTESIAN_POINT('',(1.48277387709903,4.95,-57.158126120696));
#43370=CARTESIAN_POINT('',(1.48277387709903,0.75,-57.158126120696));
#43371=CARTESIAN_POINT('Origin',(10.4334709354135,4.95,-56.2173699512871));
#43372=CARTESIAN_POINT('',(10.4334709354135,0.75,-56.2173699512871));
#43373=CARTESIAN_POINT('',(10.4334709354135,4.95,-56.2173699512871));
#43374=CARTESIAN_POINT('',(10.4334709354135,0.75,-56.2173699512871));
#43375=CARTESIAN_POINT('Origin',(11.8968694211606,4.95,-70.140676486443));
#43376=CARTESIAN_POINT('',(11.8968694211606,0.75,-70.140676486443));
#43377=CARTESIAN_POINT('Origin',(2.86608611923687,4.75,-24.0304255595508));
#43378=CARTESIAN_POINT('',(13.3342143560438,4.55,-55.600797903511));
#43379=CARTESIAN_POINT('',(3.0562974224959,4.55,-23.9686221606758));
#43380=CARTESIAN_POINT('',(12.8301849517758,4.95,-55.343982094743));
#43381=CARTESIAN_POINT('',(2.67587481597784,4.95,-24.0922289584258));
#43382=CARTESIAN_POINT('',(12.8301849517758,4.95,-55.343982094743));
#43383=CARTESIAN_POINT('Origin',(21.162975036023,4.75,-52.8467869166444));
#43384=CARTESIAN_POINT('',(22.1505388114683,4.95,-52.3156155498685));
#43385=CARTESIAN_POINT('',(21.101171637148,4.95,-52.6565756133854));
#43386=CARTESIAN_POINT('',(21.8937230027002,4.55,-52.8196449541365));
#43387=CARTESIAN_POINT('',(24.714060081258,8.94277798681721,-47.2844217746935));
#43388=CARTESIAN_POINT('',(21.224778434898,4.55,-53.0369982199034));
#43389=CARTESIAN_POINT('Origin',(13.3342143560438,4.95,-55.600797903511));
#43390=CARTESIAN_POINT('',(13.3342143560438,0.75,-55.600797903511));
#43391=CARTESIAN_POINT('',(13.3342143560438,4.95,-55.600797903511));
#43392=CARTESIAN_POINT('',(13.3342143560438,0.75,-55.600797903511));
#43393=CARTESIAN_POINT('Origin',(21.8937230027002,4.95,-52.8196449541365));
#43394=CARTESIAN_POINT('',(21.8937230027002,0.75,-52.8196449541365));
#43395=CARTESIAN_POINT('',(21.8937230027002,4.95,-52.8196449541365));
#43396=CARTESIAN_POINT('',(21.8937230027002,0.75,-52.8196449541365));
#43397=CARTESIAN_POINT('Origin',(13.9691363330359,4.75,-27.7830614264924));
#43398=CARTESIAN_POINT('',(13.7789250297769,4.55,-27.8448648253674));
#43399=CARTESIAN_POINT('',(14.159347636295,4.95,-27.7212580276174));
#43400=CARTESIAN_POINT('Origin',(0.,4.95,10.01));
#43401=CARTESIAN_POINT('',(-32.5435244785437,4.95,-46.5670378541992));
#43402=CARTESIAN_POINT('',(-28.5186714144556,4.95,-48.8907878541992));
#43403=CARTESIAN_POINT('',(-16.3262959055732,4.95,-18.4779740078565));
#43404=CARTESIAN_POINT('',(-34.2313826750721,4.95,-45.3407370931789));
#43405=CARTESIAN_POINT('',(-17.6239358377411,4.95,-26.8962987962786));
#43406=CARTESIAN_POINT('',(-41.5142019647506,4.95,-38.7832571508621));
#43407=CARTESIAN_POINT('',(-38.6895075057463,4.95,-41.3266234656553));
#43408=CARTESIAN_POINT('',(-20.2228408829076,4.95,-15.13680507562));
#43409=CARTESIAN_POINT('',(-42.9102141453889,4.95,-37.2328285521912));
#43410=CARTESIAN_POINT('',(-23.4599366320489,4.95,-23.1013747572434));
#43411=CARTESIAN_POINT('',(-48.6705096178551,4.95,-29.3044620073167));
#43412=CARTESIAN_POINT('',(-46.8478639959926,4.95,-31.8131184886743));
#43413=CARTESIAN_POINT('',(-23.5571131438905,4.95,-11.0585114463215));
#43414=CARTESIAN_POINT('',(-49.7136633514998,4.95,-27.497666740539));
#43415=CARTESIAN_POINT('',(-28.5781342694837,4.95,-18.0875229140527));
#43416=CARTESIAN_POINT('',(-53.6996824536426,4.95,-18.5449212556416));
#43417=CARTESIAN_POINT('',(-52.6512353814078,4.95,-20.8997719353731));
#43418=CARTESIAN_POINT('',(-26.1693351681284,4.95,-6.28762092762461));
#43419=CARTESIAN_POINT('',(-54.3443869165264,4.95,-16.5607249438808));
#43420=CARTESIAN_POINT('',(-32.6876140917459,4.95,-11.9574357753767));
#43421=CARTESIAN_POINT('',(-56.3819214865404,4.95,-6.97487845668955));
#43422=CARTESIAN_POINT('',(-55.9132113464906,4.95,-9.17998629418566));
#43423=CARTESIAN_POINT('',(-27.8781154566233,4.95,-0.916207452461114));
#43424=CARTESIAN_POINT('',(-56.6,4.95,-4.90000000000001));
#43425=CARTESIAN_POINT('',(-35.5,4.95,-4.9));
#43426=CARTESIAN_POINT('',(-56.6,4.95,4.89999999999999));
#43427=CARTESIAN_POINT('',(-56.6,4.95,2.75499999999999));
#43428=CARTESIAN_POINT('',(-28.5,4.95,4.9));
#43429=CARTESIAN_POINT('',(-56.3819214865404,4.95,6.97487845668952));
#43430=CARTESIAN_POINT('',(-36.7608655603543,4.95,2.80429427268419));
#43431=CARTESIAN_POINT('',(-54.3443869165264,4.95,16.5607249438808));
#43432=CARTESIAN_POINT('',(-54.8130970565762,4.95,14.3556171063847));
#43433=CARTESIAN_POINT('',(-27.8762977852036,4.95,10.9347589241512));
#43434=CARTESIAN_POINT('',(-53.6996824536427,4.95,18.5449212556415));
#43435=CARTESIAN_POINT('',(-36.2835932231409,4.95,10.7907787443291));
#43436=CARTESIAN_POINT('',(-49.7136633514998,4.95,27.497666740539));
#43437=CARTESIAN_POINT('',(-50.7621104237346,4.95,25.1428160608075));
#43438=CARTESIAN_POINT('',(-25.9027559174999,4.95,16.896367727696));
#43439=CARTESIAN_POINT('',(-48.6705096178552,4.95,29.3044620073167));
#43440=CARTESIAN_POINT('',(-33.9802699685724,4.95,18.6313781555222));
#43441=CARTESIAN_POINT('',(-42.9102141453889,4.95,37.2328285521912));
#43442=CARTESIAN_POINT('',(-44.7328597672515,4.95,34.7241720708337));
#43443=CARTESIAN_POINT('',(-22.5568555354815,4.95,22.4452479343494));
#43444=CARTESIAN_POINT('',(-41.5142019647506,4.95,38.7832571508621));
#43445=CARTESIAN_POINT('',(-29.8843372137378,4.95,25.8669838126164));
#43446=CARTESIAN_POINT('',(-34.2313826750722,4.95,45.3407370931789));
#43447=CARTESIAN_POINT('',(-37.0560771340764,4.95,42.7973707783858));
#43448=CARTESIAN_POINT('',(-17.9176036795473,4.95,27.2224499765914));
#43449=CARTESIAN_POINT('',(-32.5435244785438,4.95,46.5670378541992));
#43450=CARTESIAN_POINT('',(-24.1607530515143,4.95,32.0476518343475));
#43451=CARTESIAN_POINT('',(-24.0564755214563,4.95,51.4670378541992));
#43452=CARTESIAN_POINT('',(-28.0813285855444,4.95,49.1432878541992));
#43453=CARTESIAN_POINT('',(-12.1737040944268,4.95,30.8854740078565));
#43454=CARTESIAN_POINT('',(-22.1505388114683,4.95,52.3156155498684));
#43455=CARTESIAN_POINT('',(-17.1012128240188,4.95,36.775388084464));
#43456=CARTESIAN_POINT('',(-12.8301849517758,4.95,55.3439820947429));
#43457=CARTESIAN_POINT('',(-18.1593064494242,4.95,53.6124455565388));
#43458=CARTESIAN_POINT('',(-5.61774000370167,4.95,33.1463590152724));
#43459=CARTESIAN_POINT('',(-10.7894683082538,4.95,55.7777498078328));
#43460=CARTESIAN_POINT('',(-9.10421673957771,4.95,39.7436521863985));
#43461=CARTESIAN_POINT('',(-1.04315373364469,4.95,56.8021287478558));
#43462=CARTESIAN_POINT('',(-7.6336862792564,4.95,56.1094358646557));
#43463=CARTESIAN_POINT('',(1.37379707790495,4.95,33.8063778588436));
#43464=CARTESIAN_POINT('',(1.04315373364462,4.95,56.8021287478558));
#43465=CARTESIAN_POINT('',(-0.64209783503142,4.95,40.7680311264215));
#43466=CARTESIAN_POINT('',(10.7894683082537,4.95,55.7777498078328));
#43467=CARTESIAN_POINT('',(3.1583377500991,4.95,56.5798139493601));
#43468=CARTESIAN_POINT('',(8.37251749670409,4.95,32.7819989188206));
#43469=CARTESIAN_POINT('',(12.8301849517758,4.95,55.3439820947429));
#43470=CARTESIAN_POINT('',(7.78085896432628,4.95,39.8037546293385));
#43471=CARTESIAN_POINT('',(22.1505388114683,4.95,52.3156155498684));
#43472=CARTESIAN_POINT('',(13.879552126096,4.95,55.003022031226));
#43473=CARTESIAN_POINT('',(14.9380938633942,4.95,30.1179924703979));
#43474=CARTESIAN_POINT('',(24.0564755214562,4.95,51.4670378541992));
#43475=CARTESIAN_POINT('',(15.6737040944268,4.95,36.9476518343476));
#43476=CARTESIAN_POINT('',(32.5435244785437,4.95,46.5670378541992));
#43477=CARTESIAN_POINT('',(24.1842142685144,4.95,51.3932878541992));
#43478=CARTESIAN_POINT('',(20.6607530515143,4.95,25.9854740078565));
#43479=CARTESIAN_POINT('',(34.2313826750721,4.95,45.340737093179));
#43480=CARTESIAN_POINT('',(22.6015179240593,4.95,32.4244637549332));
#43481=CARTESIAN_POINT('',(41.5142019647506,4.95,38.7832571508621));
#43482=CARTESIAN_POINT('',(33.7119254194281,4.95,45.8084585070007));
#43483=CARTESIAN_POINT('',(25.2004229692258,4.95,20.6649700342747));
#43484=CARTESIAN_POINT('',(42.9102141453889,4.95,37.2328285521913));
#43485=CARTESIAN_POINT('',(28.2199744961061,4.95,26.5597447003967));
#43486=CARTESIAN_POINT('',(48.6705096178552,4.95,29.3044620073168));
#43487=CARTESIAN_POINT('',(42.0878261319353,4.95,38.3647485455209));
#43488=CARTESIAN_POINT('',(28.3171510079477,4.95,14.5168813894749));
#43489=CARTESIAN_POINT('',(49.7136633514998,4.95,27.4976667405391));
#43490=CARTESIAN_POINT('',(32.2975741209981,4.95,19.7435242292266));
#43491=CARTESIAN_POINT('',(53.6996824536426,4.95,18.5449212556416));
#43492=CARTESIAN_POINT('',(48.9317955298934,4.95,29.2537706201992));
#43493=CARTESIAN_POINT('',(29.8887750196427,4.95,7.94362224279855));
#43494=CARTESIAN_POINT('',(54.3443869165264,4.95,16.5607249438809));
#43495=CARTESIAN_POINT('',(34.7233309903403,4.95,12.3901407598755));
#43496=CARTESIAN_POINT('',(56.3819214865404,4.95,6.97487845668956));
#43497=CARTESIAN_POINT('',(53.8774944478963,4.95,18.7572813096869));
#43498=CARTESIAN_POINT('',(29.9138323552177,4.95,1.3489124369599));
#43499=CARTESIAN_POINT('',(56.6,4.95,4.9));
#43500=CARTESIAN_POINT('',(35.5,4.95,4.9));
#43501=CARTESIAN_POINT('',(56.6,4.95,-4.9));
#43502=CARTESIAN_POINT('',(56.6,4.95,7.255));
#43503=CARTESIAN_POINT('',(28.5,4.95,-4.9));
#43504=CARTESIAN_POINT('',(56.3819214865404,4.95,-6.97487845668953));
#43505=CARTESIAN_POINT('',(34.7251486617599,4.95,-2.37158928818542));
#43506=CARTESIAN_POINT('',(54.3443869165264,4.95,-16.5607249438808));
#43507=CARTESIAN_POINT('',(56.8488139551706,4.95,-4.77832209088351));
#43508=CARTESIAN_POINT('',(25.8405808866093,4.95,-10.5020539396524));
#43509=CARTESIAN_POINT('',(53.6996824536426,4.95,-18.5449212556415));
#43510=CARTESIAN_POINT('',(32.5641533716266,4.95,-9.13477742915521));
#43511=CARTESIAN_POINT('',(49.7136633514998,4.95,-27.497666740539));
#43512=CARTESIAN_POINT('',(54.4815502752489,4.95,-16.7888173759814));
#43513=CARTESIAN_POINT('',(22.1833160659855,4.95,-15.2403664125221));
#43514=CARTESIAN_POINT('',(48.6705096178552,4.95,-29.3044620073167));
#43515=CARTESIAN_POINT('',(29.2202321045151,4.95,-15.1730082123688));
#43516=CARTESIAN_POINT('',(42.9102141453889,4.95,-37.2328285521912));
#43517=CARTESIAN_POINT('',(49.4928976313087,4.95,-28.172542013987));
#43518=CARTESIAN_POINT('',(17.7968176714243,4.95,-18.986877991196));
#43519=CARTESIAN_POINT('',(41.5142019647506,4.95,-38.7832571508621));
#43520=CARTESIAN_POINT('',(24.9067551274196,4.95,-20.3388188539618));
#43521=CARTESIAN_POINT('',(34.2313826750722,4.95,-45.3407370931789));
#43522=CARTESIAN_POINT('',(42.0336592203946,4.95,-38.3155357370404));
#43523=CARTESIAN_POINT('',(12.9400215932291,4.95,-21.6942850179368));
#43524=CARTESIAN_POINT('',(32.5435244785438,4.95,-46.5670378541992));
#43525=CARTESIAN_POINT('',(19.8262959055732,4.95,-24.5401518343476));
#43526=CARTESIAN_POINT('',(24.0564755214563,4.95,-51.4670378541992));
#43527=CARTESIAN_POINT('',(32.4157857314856,4.95,-46.6407878541992));
#43528=CARTESIAN_POINT('',(7.8392469484857,4.95,-23.3779740078565));
#43529=CARTESIAN_POINT('',(-9.56543778402222,4.95,-2.95));
#43530=CARTESIAN_POINT('',(-12.4,4.95,-2.95));
#43531=CARTESIAN_POINT('',(6.,4.95,-2.95));
#43532=CARTESIAN_POINT('',(9.56543778402222,4.95,-2.95));
#43533=CARTESIAN_POINT('Origin',(0.,4.95,0.));
#43534=CARTESIAN_POINT('',(12.4,4.95,-2.95));
#43535=CARTESIAN_POINT('',(6.,4.95,-2.95));
#43536=CARTESIAN_POINT('',(12.4,4.95,2.95));
#43537=CARTESIAN_POINT('',(12.4,4.95,6.28));
#43538=CARTESIAN_POINT('',(9.56543778402222,4.95,2.95));
#43539=CARTESIAN_POINT('',(-6.,4.95,2.95));
#43540=CARTESIAN_POINT('',(-9.56543778402222,4.95,2.95));
#43541=CARTESIAN_POINT('Origin',(0.,4.95,0.));
#43542=CARTESIAN_POINT('',(-12.4,4.95,2.95));
#43543=CARTESIAN_POINT('',(-6.,4.95,2.95));
#43544=CARTESIAN_POINT('',(-12.4,4.95,3.73));
#43545=CARTESIAN_POINT('Origin',(8.01245202924258,4.75,-23.2779740078565));
#43546=CARTESIAN_POINT('',(24.60288568297,4.55,-51.613448015713));
#43547=CARTESIAN_POINT('',(8.18565710999947,4.55,-23.1779740078565));
#43548=CARTESIAN_POINT('',(24.0564755214563,4.95,-51.4670378541992));
#43549=CARTESIAN_POINT('Origin',(32.5157857314856,4.75,-46.8139929349561));
#43550=CARTESIAN_POINT('',(32.39711431703,4.55,-47.113448015713));
#43551=CARTESIAN_POINT('',(32.5435244785438,4.95,-46.5670378541992));
#43552=CARTESIAN_POINT('',(32.6157857314856,4.55,-46.987198015713));
#43553=CARTESIAN_POINT('Origin',(19.6530908248163,4.75,-24.6401518343476));
#43554=CARTESIAN_POINT('',(19.4798857440594,4.55,-24.7401518343476));
#43555=CARTESIAN_POINT('Origin',(13.0886505583246,4.75,-21.5604588966651));
#43556=CARTESIAN_POINT('',(34.7962928478066,4.55,-45.3703427808263));
#43557=CARTESIAN_POINT('',(13.2372795234201,4.55,-21.4266327753933));
#43558=CARTESIAN_POINT('',(34.2313826750722,4.95,-45.3407370931789));
#43559=CARTESIAN_POINT('Origin',(42.1674853416664,4.75,-38.4641647021359));
#43560=CARTESIAN_POINT('',(41.4845962771032,4.55,-39.3481673235966));
#43561=CARTESIAN_POINT('',(41.5142019647506,4.95,-38.7832571508621));
#43562=CARTESIAN_POINT('',(42.3013114629382,4.55,-38.6127936672313));
#43563=CARTESIAN_POINT('Origin',(24.7581261623241,4.75,-20.4726449752336));
#43564=CARTESIAN_POINT('',(24.6094971972286,4.55,-20.6064710965053));
#43565=CARTESIAN_POINT('Origin',(17.9143747218828,4.75,-18.825074592321));
#43566=CARTESIAN_POINT('',(43.4689350440559,4.55,-37.1443358553582));
#43567=CARTESIAN_POINT('',(18.0319317723412,4.55,-18.6632711934461));
#43568=CARTESIAN_POINT('',(42.9102141453889,4.95,-37.2328285521912));
#43569=CARTESIAN_POINT('Origin',(49.6547010301837,4.75,-28.2900990644455));
#43570=CARTESIAN_POINT('',(48.7590023146881,4.55,-29.8631829059837));
#43571=CARTESIAN_POINT('',(48.6705096178552,4.95,-29.3044620073167));
#43572=CARTESIAN_POINT('',(49.8165044290587,4.55,-28.407656114904));
#43573=CARTESIAN_POINT('Origin',(29.1026750540566,4.75,-15.3348116112438));
#43574=CARTESIAN_POINT('',(28.9851180035981,4.55,-15.4966150101188));
#43575=CARTESIAN_POINT('Origin',(22.2646633946007,4.75,-15.0576573209936));
#43576=CARTESIAN_POINT('',(50.2417761917872,4.55,-27.2949432147123));
#43577=CARTESIAN_POINT('',(22.3460107232159,4.55,-14.8749482294651));
#43578=CARTESIAN_POINT('',(49.7136633514998,4.95,-27.497666740539));
#43579=CARTESIAN_POINT('Origin',(54.6642593667775,4.75,-16.8701647045966));
#43580=CARTESIAN_POINT('',(53.9024059794694,4.55,-19.0730340959289));
#43581=CARTESIAN_POINT('',(53.6996824536426,4.95,-18.5449212556415));
#43582=CARTESIAN_POINT('',(54.846968458306,4.55,-16.9515120332117));
#43583=CARTESIAN_POINT('Origin',(32.4828060430114,4.75,-9.31748652068373));
#43584=CARTESIAN_POINT('',(32.4014587143963,4.55,-9.50019561221225));
#43585=CARTESIAN_POINT('Origin',(25.8821632247728,4.75,-10.3064244195056));
#43586=CARTESIAN_POINT('',(54.818810633147,4.55,-16.2526305799144));
#43587=CARTESIAN_POINT('',(25.9237455629364,4.55,-10.1107948993589));
#43588=CARTESIAN_POINT('',(54.3443869165264,4.95,-16.5607249438808));
#43589=CARTESIAN_POINT('Origin',(57.0444434753173,4.75,-4.81990442904706));
#43590=CARTESIAN_POINT('',(56.6900158505068,4.55,-7.44930217331016));
#43591=CARTESIAN_POINT('',(56.3819214865404,4.95,-6.97487845668953));
#43592=CARTESIAN_POINT('',(57.2400729954641,4.55,-4.86148676721061));
#43593=CARTESIAN_POINT('Origin',(34.6835663235964,4.75,-2.56721880833218));
#43594=CARTESIAN_POINT('',(34.6419839854328,4.55,-2.76284832847894));
#43595=CARTESIAN_POINT('Origin',(28.5,4.75,-4.7));
#43596=CARTESIAN_POINT('',(57.,4.55,-4.5));
#43597=CARTESIAN_POINT('',(28.5,4.55,-4.5));
#43598=CARTESIAN_POINT('',(56.6,4.95,-4.9));
#43599=CARTESIAN_POINT('Origin',(56.8,4.75,7.255));
#43600=CARTESIAN_POINT('',(57.,4.55,4.5));
#43601=CARTESIAN_POINT('',(56.6,4.95,4.9));
#43602=CARTESIAN_POINT('',(57.,4.55,7.255));
#43603=CARTESIAN_POINT('Origin',(35.5,4.75,4.7));
#43604=CARTESIAN_POINT('',(35.5,4.55,4.5));
#43605=CARTESIAN_POINT('Origin',(-28.6186714144556,4.75,-49.0639929349561));
#43606=CARTESIAN_POINT('',(-32.39711431703,4.55,-47.113448015713));
#43607=CARTESIAN_POINT('',(-28.7186714144556,4.55,-49.237198015713));
#43608=CARTESIAN_POINT('',(-34.1898431262531,9.44782619099021,-40.4228930154996));
#43609=CARTESIAN_POINT('Origin',(-24.60288568297,4.95,-51.613448015713));
#43610=CARTESIAN_POINT('',(-32.39711431703,0.75,-47.113448015713));
#43611=CARTESIAN_POINT('',(-24.60288568297,0.75,-51.613448015713));
#43612=CARTESIAN_POINT('',(-32.39711431703,4.95,-47.113448015713));
#43613=CARTESIAN_POINT('Origin',(-16.1530908248163,4.75,-18.5779740078565));
#43614=CARTESIAN_POINT('',(-15.9798857440594,4.55,-18.6779740078565));
#43615=CARTESIAN_POINT('Origin',(-20.0742119178121,4.75,-15.2706311968918));
#43616=CARTESIAN_POINT('',(-41.4845962771032,4.55,-39.3481673235966));
#43617=CARTESIAN_POINT('',(-19.9255829527166,4.55,-15.4044573181636));
#43618=CARTESIAN_POINT('',(-41.5142019647506,4.95,-38.7832571508621));
#43619=CARTESIAN_POINT('Origin',(-38.8233336270181,4.75,-41.4752524307507));
#43620=CARTESIAN_POINT('',(-34.7962928478066,4.55,-45.3703427808263));
#43621=CARTESIAN_POINT('',(-38.9571597482899,4.55,-41.6238813958462));
#43622=CARTESIAN_POINT('',(-34.2313826750721,4.95,-45.3407370931789));
#43623=CARTESIAN_POINT('Origin',(-17.7725648028366,4.75,-26.7624726750068));
#43624=CARTESIAN_POINT('',(-17.9211937679321,4.55,-26.6286465537351));
#43625=CARTESIAN_POINT('Origin',(-41.4845962771032,4.95,-39.3481673235966));
#43626=CARTESIAN_POINT('',(-41.4845962771032,0.75,-39.3481673235966));
#43627=CARTESIAN_POINT('',(-41.4845962771032,4.95,-39.3481673235966));
#43628=CARTESIAN_POINT('',(-41.4845962771032,0.75,-39.3481673235966));
#43629=CARTESIAN_POINT('Origin',(-34.7962928478066,4.95,-45.3703427808263));
#43630=CARTESIAN_POINT('',(-34.7962928478066,0.75,-45.3703427808263));
#43631=CARTESIAN_POINT('',(-34.7962928478066,4.95,-45.3703427808263));
#43632=CARTESIAN_POINT('',(-34.7962928478066,0.75,-45.3703427808263));
#43633=CARTESIAN_POINT('Origin',(-44.1641213368306,4.95,-55.7743703375099));
#43634=CARTESIAN_POINT('',(-44.1641213368306,0.75,-55.7743703375099));
#43635=CARTESIAN_POINT('Origin',(-23.439556093432,4.75,-11.2203148451965));
#43636=CARTESIAN_POINT('',(-48.7590023146881,4.55,-29.8631829059837));
#43637=CARTESIAN_POINT('',(-23.3219990429735,4.55,-11.3821182440715));
#43638=CARTESIAN_POINT('',(-48.6705096178551,4.95,-29.3044620073167));
#43639=CARTESIAN_POINT('Origin',(-47.0096673948676,4.75,-31.9306755391328));
#43640=CARTESIAN_POINT('',(-43.4689350440559,4.55,-37.1443358553582));
#43641=CARTESIAN_POINT('',(-47.1714707937426,4.55,-32.0482325895913));
#43642=CARTESIAN_POINT('',(-42.9102141453889,4.95,-37.2328285521912));
#43643=CARTESIAN_POINT('Origin',(-23.5774936825074,4.75,-22.9395713583684));
#43644=CARTESIAN_POINT('',(-23.6950507329659,4.55,-22.7777679594934));
#43645=CARTESIAN_POINT('Origin',(-48.7590023146881,4.95,-29.8631829059837));
#43646=CARTESIAN_POINT('',(-48.7590023146881,0.75,-29.8631829059837));
#43647=CARTESIAN_POINT('',(-48.7590023146881,4.95,-29.8631829059837));
#43648=CARTESIAN_POINT('',(-48.7590023146881,0.75,-29.8631829059837));
#43649=CARTESIAN_POINT('Origin',(-43.4689350440559,4.95,-37.1443358553582));
#43650=CARTESIAN_POINT('',(-43.4689350440559,0.75,-37.1443358553582));
#43651=CARTESIAN_POINT('',(-43.4689350440559,4.95,-37.1443358553582));
#43652=CARTESIAN_POINT('',(-43.4689350440559,0.75,-37.1443358553582));
#43653=CARTESIAN_POINT('Origin',(-54.7951729653051,4.95,-45.3733293874529));
#43654=CARTESIAN_POINT('',(-54.7951729653051,0.75,-45.3733293874529));
#43655=CARTESIAN_POINT('Origin',(-26.0879878395132,4.75,-6.47033001915313));
#43656=CARTESIAN_POINT('',(-53.9024059794693,4.55,-19.0730340959289));
#43657=CARTESIAN_POINT('',(-26.006640510898,4.55,-6.65303911068165));
#43658=CARTESIAN_POINT('',(-53.6996824536426,4.95,-18.5449212556416));
#43659=CARTESIAN_POINT('Origin',(-52.8339444729364,4.75,-20.9811192639883));
#43660=CARTESIAN_POINT('',(-50.2417761917871,4.55,-27.2949432147123));
#43661=CARTESIAN_POINT('',(-53.0166535644649,4.55,-21.0624665926034));
#43662=CARTESIAN_POINT('',(-49.7136633514998,4.95,-27.497666740539));
#43663=CARTESIAN_POINT('Origin',(-28.6594815980989,4.75,-17.9048138225242));
#43664=CARTESIAN_POINT('',(-28.740828926714,4.55,-17.7221047309957));
#43665=CARTESIAN_POINT('Origin',(-53.9024059794693,4.95,-19.0730340959289));
#43666=CARTESIAN_POINT('',(-53.9024059794693,0.75,-19.0730340959289));
#43667=CARTESIAN_POINT('',(-53.9024059794693,4.95,-19.0730340959289));
#43668=CARTESIAN_POINT('',(-53.9024059794693,0.75,-19.0730340959289));
#43669=CARTESIAN_POINT('Origin',(-50.2417761917871,4.95,-27.2949432147123));
#43670=CARTESIAN_POINT('',(-50.2417761917871,0.75,-27.2949432147123));
#43671=CARTESIAN_POINT('',(-50.2417761917871,4.95,-27.2949432147123));
#43672=CARTESIAN_POINT('',(-50.2417761917871,0.75,-27.2949432147123));
#43673=CARTESIAN_POINT('Origin',(-63.0314125987836,4.95,-32.9892562177735));
#43674=CARTESIAN_POINT('',(-63.0314125987836,0.75,-32.9892562177735));
#43675=CARTESIAN_POINT('Origin',(-27.8365331184597,4.75,-1.11183697260787));
#43676=CARTESIAN_POINT('',(-56.6900158505068,4.55,-7.44930217331018));
#43677=CARTESIAN_POINT('',(-27.7949507802962,4.55,-1.30746649275464));
#43678=CARTESIAN_POINT('',(-56.3819214865404,4.95,-6.97487845668955));
#43679=CARTESIAN_POINT('Origin',(-56.1088408666374,4.75,-9.22156863234921));
#43680=CARTESIAN_POINT('',(-54.818810633147,4.55,-16.2526305799144));
#43681=CARTESIAN_POINT('',(-56.3044703867841,4.55,-9.26315097051276));
#43682=CARTESIAN_POINT('',(-54.3443869165264,4.95,-16.5607249438808));
#43683=CARTESIAN_POINT('Origin',(-32.7291964299094,4.75,-11.76180625523));
#43684=CARTESIAN_POINT('',(-32.770778768073,4.55,-11.5661767350832));
#43685=CARTESIAN_POINT('Origin',(-56.6900158505068,4.95,-7.44930217331018));
#43686=CARTESIAN_POINT('',(-56.6900158505068,0.75,-7.44930217331018));
#43687=CARTESIAN_POINT('',(-56.6900158505068,4.95,-7.44930217331018));
#43688=CARTESIAN_POINT('',(-56.6900158505068,0.75,-7.44930217331018));
#43689=CARTESIAN_POINT('Origin',(-54.818810633147,4.95,-16.2526305799144));
#43690=CARTESIAN_POINT('',(-54.818810633147,0.75,-16.2526305799144));
#43691=CARTESIAN_POINT('',(-54.818810633147,4.95,-16.2526305799144));
#43692=CARTESIAN_POINT('',(-54.818810633147,0.75,-16.2526305799144));
#43693=CARTESIAN_POINT('Origin',(-68.5128770434203,4.95,-19.1633942513631));
#43694=CARTESIAN_POINT('',(-68.5128770434203,0.75,-19.1633942513631));
#43695=CARTESIAN_POINT('Origin',(-28.5,4.75,4.7));
#43696=CARTESIAN_POINT('',(-57.,4.55,4.49999999999999));
#43697=CARTESIAN_POINT('',(-28.5,4.55,4.5));
#43698=CARTESIAN_POINT('',(-56.6,4.95,4.89999999999999));
#43699=CARTESIAN_POINT('Origin',(-56.8,4.75,2.75499999999999));
#43700=CARTESIAN_POINT('',(-57.,4.55,-4.50000000000001));
#43701=CARTESIAN_POINT('',(-57.,4.55,2.75499999999999));
#43702=CARTESIAN_POINT('',(-56.6,4.95,-4.90000000000001));
#43703=CARTESIAN_POINT('Origin',(-35.5,4.75,-4.7));
#43704=CARTESIAN_POINT('',(-35.5,4.55,-4.5));
#43705=CARTESIAN_POINT('Origin',(-57.,4.95,4.49999999999999));
#43706=CARTESIAN_POINT('',(-57.,0.75,4.49999999999999));
#43707=CARTESIAN_POINT('',(-57.,4.95,4.49999999999999));
#43708=CARTESIAN_POINT('',(-57.,0.75,4.49999999999999));
#43709=CARTESIAN_POINT('Origin',(-57.,4.95,-4.50000000000001));
#43710=CARTESIAN_POINT('',(-57.,0.75,-4.50000000000001));
#43711=CARTESIAN_POINT('',(-57.,4.95,-4.50000000000001));
#43712=CARTESIAN_POINT('',(-57.,0.75,-4.50000000000001));
#43713=CARTESIAN_POINT('Origin',(-71.,4.95,-4.50000000000001));
#43714=CARTESIAN_POINT('',(-71.,0.75,-4.50000000000001));
#43715=CARTESIAN_POINT('Origin',(-27.9178801233672,4.75,10.7391294040044));
#43716=CARTESIAN_POINT('',(-54.818810633147,4.55,16.2526305799144));
#43717=CARTESIAN_POINT('',(-27.9594624615307,4.55,10.5434998838576));
#43718=CARTESIAN_POINT('',(-54.3443869165264,4.95,16.5607249438808));
#43719=CARTESIAN_POINT('Origin',(-55.0087265767229,4.75,14.3971994445483));
#43720=CARTESIAN_POINT('',(-56.6900158505068,4.55,7.44930217331014));
#43721=CARTESIAN_POINT('',(-55.2043560968697,4.55,14.4387817827118));
#43722=CARTESIAN_POINT('',(-56.3819214865404,4.95,6.97487845668952));
#43723=CARTESIAN_POINT('Origin',(-36.7192832221907,4.75,2.99992379283095));
#43724=CARTESIAN_POINT('',(-36.6777008840272,4.55,3.19555331297771));
#43725=CARTESIAN_POINT('Origin',(-54.818810633147,4.95,16.2526305799144));
#43726=CARTESIAN_POINT('',(-54.818810633147,0.75,16.2526305799144));
#43727=CARTESIAN_POINT('',(-54.818810633147,4.95,16.2526305799144));
#43728=CARTESIAN_POINT('',(-54.818810633147,0.75,16.2526305799144));
#43729=CARTESIAN_POINT('Origin',(-56.6900158505068,4.95,7.44930217331014));
#43730=CARTESIAN_POINT('',(-56.6900158505068,0.75,7.44930217331014));
#43731=CARTESIAN_POINT('',(-56.6900158505068,4.95,7.44930217331014));
#43732=CARTESIAN_POINT('',(-56.6900158505068,0.75,7.44930217331014));
#43733=CARTESIAN_POINT('Origin',(-70.3840822607801,4.95,10.3600658447588));
#43734=CARTESIAN_POINT('',(-70.3840822607801,0.75,10.3600658447588));
#43735=CARTESIAN_POINT('Origin',(-36.2022458945258,4.75,10.9734878358576));
#43736=CARTESIAN_POINT('',(-53.9024059794694,4.55,19.0730340959289));
#43737=CARTESIAN_POINT('',(-36.1208985659106,4.55,11.1561969273861));
#43738=CARTESIAN_POINT('',(-52.7669863049298,6.79033134765063,16.1151647179474));
#43739=CARTESIAN_POINT('Origin',(-66.6920423864658,4.95,24.7673470989901));
#43740=CARTESIAN_POINT('',(-53.9024059794694,0.75,19.0730340959289));
#43741=CARTESIAN_POINT('',(-66.6920423864658,0.75,24.7673470989901));
#43742=CARTESIAN_POINT('',(-53.9024059794694,4.95,19.0730340959289));
#43743=CARTESIAN_POINT('Origin',(-25.984103246115,4.75,16.7136586361675));
#43744=CARTESIAN_POINT('',(-50.2417761917872,4.55,27.2949432147123));
#43745=CARTESIAN_POINT('',(-26.0654505747302,4.55,16.530949544639));
#43746=CARTESIAN_POINT('',(-49.7136633514998,4.95,27.497666740539));
#43747=CARTESIAN_POINT('Origin',(-50.9448195152631,4.75,25.2241633894226));
#43748=CARTESIAN_POINT('',(-51.1275286067916,4.55,25.3055107180378));
#43749=CARTESIAN_POINT('Origin',(-50.2417761917872,4.95,27.2949432147123));
#43750=CARTESIAN_POINT('',(-50.2417761917872,0.75,27.2949432147123));
#43751=CARTESIAN_POINT('',(-50.2417761917872,4.95,27.2949432147123));
#43752=CARTESIAN_POINT('',(-50.2417761917872,0.75,27.2949432147123));
#43753=CARTESIAN_POINT('Origin',(-53.9024059794694,4.95,19.0730340959289));
#43754=CARTESIAN_POINT('',(-53.9024059794694,0.75,19.0730340959289));
#43755=CARTESIAN_POINT('Origin',(-22.67441258594,4.75,22.2834445354744));
#43756=CARTESIAN_POINT('',(-43.4689350440559,4.55,37.1443358553582));
#43757=CARTESIAN_POINT('',(-22.7919696363985,4.55,22.1216411365994));
#43758=CARTESIAN_POINT('',(-42.9102141453889,4.95,37.2328285521912));
#43759=CARTESIAN_POINT('Origin',(-44.8946631661265,4.75,34.8417291212921));
#43760=CARTESIAN_POINT('',(-48.7590023146881,4.55,29.8631829059837));
#43761=CARTESIAN_POINT('',(-45.0564665650015,4.55,34.9592861717506));
#43762=CARTESIAN_POINT('',(-48.6705096178552,4.95,29.3044620073167));
#43763=CARTESIAN_POINT('Origin',(-33.8627129181139,4.75,18.7931815543972));
#43764=CARTESIAN_POINT('',(-33.7451558676554,4.55,18.9549849532722));
#43765=CARTESIAN_POINT('Origin',(-43.4689350440559,4.95,37.1443358553582));
#43766=CARTESIAN_POINT('',(-43.4689350440559,0.75,37.1443358553582));
#43767=CARTESIAN_POINT('',(-43.4689350440559,4.95,37.1443358553582));
#43768=CARTESIAN_POINT('',(-43.4689350440559,0.75,37.1443358553582));
#43769=CARTESIAN_POINT('Origin',(-48.7590023146881,4.95,29.8631829059837));
#43770=CARTESIAN_POINT('',(-48.7590023146881,0.75,29.8631829059837));
#43771=CARTESIAN_POINT('',(-48.7590023146881,4.95,29.8631829059837));
#43772=CARTESIAN_POINT('',(-48.7590023146881,0.75,29.8631829059837));
#43773=CARTESIAN_POINT('Origin',(-60.0852402359374,4.95,38.0921764380783));
#43774=CARTESIAN_POINT('',(-60.0852402359374,0.75,38.0921764380783));
#43775=CARTESIAN_POINT('Origin',(-18.0662326446428,4.75,27.0886238553197));
#43776=CARTESIAN_POINT('',(-34.7962928478067,4.55,45.3703427808263));
#43777=CARTESIAN_POINT('',(-18.2148616097383,4.55,26.9547977340479));
#43778=CARTESIAN_POINT('',(-34.2313826750722,4.95,45.3407370931789));
#43779=CARTESIAN_POINT('Origin',(-37.1899032553482,4.75,42.9459997434813));
#43780=CARTESIAN_POINT('',(-41.4845962771032,4.55,39.3481673235966));
#43781=CARTESIAN_POINT('',(-37.32372937662,4.55,43.0946287085767));
#43782=CARTESIAN_POINT('',(-41.5142019647506,4.95,38.7832571508621));
#43783=CARTESIAN_POINT('Origin',(-29.7357082486423,4.75,26.0008099338882));
#43784=CARTESIAN_POINT('',(-29.5870792835468,4.55,26.1346360551599));
#43785=CARTESIAN_POINT('Origin',(-34.7962928478067,4.95,45.3703427808263));
#43786=CARTESIAN_POINT('',(-34.7962928478067,0.75,45.3703427808263));
#43787=CARTESIAN_POINT('',(-34.7962928478067,4.95,45.3703427808263));
#43788=CARTESIAN_POINT('',(-34.7962928478067,0.75,45.3703427808263));
#43789=CARTESIAN_POINT('Origin',(-41.4845962771032,4.95,39.3481673235966));
#43790=CARTESIAN_POINT('',(-41.4845962771032,0.75,39.3481673235966));
#43791=CARTESIAN_POINT('',(-41.4845962771032,4.95,39.3481673235966));
#43792=CARTESIAN_POINT('',(-41.4845962771032,0.75,39.3481673235966));
#43793=CARTESIAN_POINT('Origin',(-50.8524247661272,4.95,49.7521948802801));
#43794=CARTESIAN_POINT('',(-50.8524247661272,0.75,49.7521948802801));
#43795=CARTESIAN_POINT('Origin',(-12.3469091751837,4.75,30.7854740078565));
#43796=CARTESIAN_POINT('',(-24.6028856829701,4.55,51.613448015713));
#43797=CARTESIAN_POINT('',(-12.5201142559406,4.55,30.6854740078565));
#43798=CARTESIAN_POINT('',(-24.0564755214563,4.95,51.4670378541992));
#43799=CARTESIAN_POINT('Origin',(-28.1813285855445,4.75,49.3164929349561));
#43800=CARTESIAN_POINT('',(-32.39711431703,4.55,47.113448015713));
#43801=CARTESIAN_POINT('',(-28.2813285855445,4.55,49.489698015713));
#43802=CARTESIAN_POINT('',(-32.5435244785438,4.95,46.5670378541992));
#43803=CARTESIAN_POINT('Origin',(-23.9875479707574,4.75,32.1476518343475));
#43804=CARTESIAN_POINT('',(-23.8143428900005,4.55,32.2476518343475));
#43805=CARTESIAN_POINT('Origin',(-24.6028856829701,4.95,51.613448015713));
#43806=CARTESIAN_POINT('',(-24.6028856829701,0.75,51.613448015713));
#43807=CARTESIAN_POINT('',(-24.6028856829701,4.95,51.613448015713));
#43808=CARTESIAN_POINT('',(-24.6028856829701,0.75,51.613448015713));
#43809=CARTESIAN_POINT('Origin',(-32.39711431703,4.95,47.113448015713));
#43810=CARTESIAN_POINT('',(-32.39711431703,0.75,47.113448015713));
#43811=CARTESIAN_POINT('',(-32.39711431703,4.95,47.113448015713));
#43812=CARTESIAN_POINT('',(-32.39711431703,0.75,47.113448015713));
#43813=CARTESIAN_POINT('Origin',(-39.39711431703,4.95,59.2378036686951));
#43814=CARTESIAN_POINT('',(-39.39711431703,0.75,59.2378036686951));
#43815=CARTESIAN_POINT('Origin',(-5.8079513069607,4.75,33.0845556163974));
#43816=CARTESIAN_POINT('',(-13.3342143560438,4.55,55.600797903511));
#43817=CARTESIAN_POINT('',(-5.99816261021973,4.55,33.0227522175225));
#43818=CARTESIAN_POINT('',(-12.8301849517758,4.95,55.3439820947429));
#43819=CARTESIAN_POINT('Origin',(-18.2211098482992,4.75,53.8026568597978));
#43820=CARTESIAN_POINT('',(-21.8937230027002,4.55,52.8196449541365));
#43821=CARTESIAN_POINT('',(-18.2829132471742,4.55,53.9928681630568));
#43822=CARTESIAN_POINT('',(-22.1505388114683,4.95,52.3156155498684));
#43823=CARTESIAN_POINT('Origin',(-16.9110015207598,4.75,36.837191483339));
#43824=CARTESIAN_POINT('',(-16.7207902175007,4.55,36.898994882214));
#43825=CARTESIAN_POINT('Origin',(-13.3342143560438,4.95,55.600797903511));
#43826=CARTESIAN_POINT('',(-13.3342143560438,0.75,55.600797903511));
#43827=CARTESIAN_POINT('',(-13.3342143560438,4.95,55.600797903511));
#43828=CARTESIAN_POINT('',(-13.3342143560438,0.75,55.600797903511));
#43829=CARTESIAN_POINT('Origin',(-21.8937230027002,4.95,52.8196449541365));
#43830=CARTESIAN_POINT('',(-21.8937230027002,0.75,52.8196449541365));
#43831=CARTESIAN_POINT('',(-21.8937230027002,4.95,52.8196449541365));
#43832=CARTESIAN_POINT('',(-21.8937230027002,0.75,52.8196449541365));
#43833=CARTESIAN_POINT('Origin',(-26.2199609239495,4.95,66.1344361822686));
#43834=CARTESIAN_POINT('',(-26.2199609239495,0.75,66.1344361822686));
#43835=CARTESIAN_POINT('Origin',(1.17489269883129,4.75,33.7854721661901));
#43836=CARTESIAN_POINT('',(-1.48277387709906,4.55,57.158126120696));
#43837=CARTESIAN_POINT('',(0.975988319757637,4.55,33.7645664735366));
#43838=CARTESIAN_POINT('',(-1.04315373364469,4.95,56.8021287478558));
#43839=CARTESIAN_POINT('Origin',(-7.65459197190993,4.75,56.3083402437293));
#43840=CARTESIAN_POINT('',(-10.4334709354135,4.55,56.2173699512871));
#43841=CARTESIAN_POINT('',(-7.67549766456346,4.55,56.507244622803));
#43842=CARTESIAN_POINT('',(-10.7894683082538,4.95,55.7777498078328));
#43843=CARTESIAN_POINT('Origin',(-8.90531236050406,4.75,39.7645578790521));
#43844=CARTESIAN_POINT('',(-8.7064079814304,4.55,39.7854635717056));
#43845=CARTESIAN_POINT('Origin',(-1.48277387709906,4.95,57.158126120696));
#43846=CARTESIAN_POINT('',(-1.48277387709906,0.75,57.158126120696));
#43847=CARTESIAN_POINT('',(-1.48277387709906,4.95,57.158126120696));
#43848=CARTESIAN_POINT('',(-1.48277387709906,0.75,57.158126120696));
#43849=CARTESIAN_POINT('Origin',(-10.4334709354135,4.95,56.2173699512871));
#43850=CARTESIAN_POINT('',(-10.4334709354135,0.75,56.2173699512871));
#43851=CARTESIAN_POINT('',(-10.4334709354135,4.95,56.2173699512871));
#43852=CARTESIAN_POINT('',(-10.4334709354135,0.75,56.2173699512871));
#43853=CARTESIAN_POINT('Origin',(-11.8968694211607,4.95,70.140676486443));
#43854=CARTESIAN_POINT('',(-11.8968694211607,0.75,70.140676486443));
#43855=CARTESIAN_POINT('Origin',(8.17361311763044,4.75,32.8029046114742));
#43856=CARTESIAN_POINT('',(10.4334709354135,4.55,56.2173699512871));
#43857=CARTESIAN_POINT('',(7.97470873855678,4.55,32.8238103041277));
#43858=CARTESIAN_POINT('',(10.7894683082537,4.95,55.7777498078328));
#43859=CARTESIAN_POINT('Origin',(3.17924344275264,4.75,56.7787183284338));
#43860=CARTESIAN_POINT('',(1.48277387709899,4.55,57.158126120696));
#43861=CARTESIAN_POINT('',(3.20014913540617,4.55,56.9776227075075));
#43862=CARTESIAN_POINT('',(1.04315373364462,4.95,56.8021287478558));
#43863=CARTESIAN_POINT('Origin',(-0.443193455957765,4.75,40.747125433768));
#43864=CARTESIAN_POINT('',(-0.24428907688411,4.55,40.7262197411145));
#43865=CARTESIAN_POINT('Origin',(10.4334709354135,4.95,56.2173699512871));
#43866=CARTESIAN_POINT('',(10.4334709354135,0.75,56.2173699512871));
#43867=CARTESIAN_POINT('',(10.4334709354135,4.95,56.2173699512871));
#43868=CARTESIAN_POINT('',(10.4334709354135,0.75,56.2173699512871));
#43869=CARTESIAN_POINT('Origin',(1.48277387709899,4.95,57.158126120696));
#43870=CARTESIAN_POINT('',(1.48277387709899,0.75,57.158126120696));
#43871=CARTESIAN_POINT('',(1.48277387709899,4.95,57.158126120696));
#43872=CARTESIAN_POINT('',(1.48277387709899,0.75,57.158126120696));
#43873=CARTESIAN_POINT('Origin',(2.94617236284613,4.95,71.0814326558519));
#43874=CARTESIAN_POINT('',(2.94617236284613,0.75,71.0814326558519));
#43875=CARTESIAN_POINT('Origin',(14.7478825601351,4.75,30.1797958692729));
#43876=CARTESIAN_POINT('',(21.8937230027002,4.55,52.8196449541365));
#43877=CARTESIAN_POINT('',(14.5576712568761,4.55,30.2415992681479));
#43878=CARTESIAN_POINT('',(22.1505388114683,4.95,52.3156155498684));
#43879=CARTESIAN_POINT('Origin',(13.941355524971,4.75,55.193233334485));
#43880=CARTESIAN_POINT('',(13.3342143560438,4.55,55.600797903511));
#43881=CARTESIAN_POINT('',(14.003158923846,4.55,55.3834446377441));
#43882=CARTESIAN_POINT('',(12.8301849517758,4.95,55.3439820947429));
#43883=CARTESIAN_POINT('Origin',(7.97107026758531,4.75,39.7419512304635));
#43884=CARTESIAN_POINT('',(8.16128157084435,4.55,39.6801478315885));
#43885=CARTESIAN_POINT('Origin',(21.8937230027002,4.95,52.8196449541365));
#43886=CARTESIAN_POINT('',(21.8937230027002,0.75,52.8196449541365));
#43887=CARTESIAN_POINT('',(21.8937230027002,4.95,52.8196449541365));
#43888=CARTESIAN_POINT('',(21.8937230027002,0.75,52.8196449541365));
#43889=CARTESIAN_POINT('Origin',(13.3342143560438,4.95,55.600797903511));
#43890=CARTESIAN_POINT('',(13.3342143560438,0.75,55.600797903511));
#43891=CARTESIAN_POINT('',(13.3342143560438,4.95,55.600797903511));
#43892=CARTESIAN_POINT('',(13.3342143560438,0.75,55.600797903511));
#43893=CARTESIAN_POINT('Origin',(17.6604522772931,4.95,68.9155891316432));
#43894=CARTESIAN_POINT('',(17.6604522772931,0.75,68.9155891316432));
#43895=CARTESIAN_POINT('Origin',(20.4875479707574,4.75,26.0854740078565));
#43896=CARTESIAN_POINT('',(32.3971143170299,4.55,47.113448015713));
#43897=CARTESIAN_POINT('',(20.3143428900005,4.55,26.1854740078565));
#43898=CARTESIAN_POINT('',(32.5435244785437,4.95,46.5670378541992));
#43899=CARTESIAN_POINT('Origin',(24.2842142685144,4.75,51.5664929349561));
#43900=CARTESIAN_POINT('',(24.60288568297,4.55,51.613448015713));
#43901=CARTESIAN_POINT('',(24.3842142685144,4.55,51.739698015713));
#43902=CARTESIAN_POINT('',(24.0564755214562,4.95,51.4670378541992));
#43903=CARTESIAN_POINT('Origin',(15.8469091751837,4.75,36.8476518343476));
#43904=CARTESIAN_POINT('',(16.0201142559406,4.55,36.7476518343476));
#43905=CARTESIAN_POINT('Origin',(32.3971143170299,4.95,47.113448015713));
#43906=CARTESIAN_POINT('',(32.3971143170299,0.75,47.113448015713));
#43907=CARTESIAN_POINT('',(32.3971143170299,4.95,47.113448015713));
#43908=CARTESIAN_POINT('',(32.3971143170299,0.75,47.113448015713));
#43909=CARTESIAN_POINT('Origin',(24.60288568297,4.95,51.613448015713));
#43910=CARTESIAN_POINT('',(24.60288568297,0.75,51.613448015713));
#43911=CARTESIAN_POINT('',(24.60288568297,4.95,51.613448015713));
#43912=CARTESIAN_POINT('',(24.60288568297,0.75,51.613448015713));
#43913=CARTESIAN_POINT('Origin',(31.60288568297,4.95,63.7378036686952));
#43914=CARTESIAN_POINT('',(31.60288568297,0.75,63.7378036686952));
#43915=CARTESIAN_POINT('Origin',(25.0517940041303,4.75,20.7987961555464));
#43916=CARTESIAN_POINT('',(41.4845962771032,4.55,39.3481673235966));
#43917=CARTESIAN_POINT('',(24.9031650390348,4.55,20.9326222768182));
#43918=CARTESIAN_POINT('',(41.5142019647506,4.95,38.7832571508621));
#43919=CARTESIAN_POINT('Origin',(33.8457515406999,4.75,45.9570874720961));
#43920=CARTESIAN_POINT('',(34.7962928478066,4.55,45.3703427808264));
#43921=CARTESIAN_POINT('',(33.9795776619717,4.55,46.1057164371916));
#43922=CARTESIAN_POINT('',(34.2313826750721,4.95,45.340737093179));
#43923=CARTESIAN_POINT('Origin',(22.7501468891548,4.75,32.2906376336614));
#43924=CARTESIAN_POINT('',(22.8987758542503,4.55,32.1568115123897));
#43925=CARTESIAN_POINT('Origin',(41.4845962771032,4.95,39.3481673235966));
#43926=CARTESIAN_POINT('',(41.4845962771032,0.75,39.3481673235966));
#43927=CARTESIAN_POINT('',(41.4845962771032,4.95,39.3481673235966));
#43928=CARTESIAN_POINT('',(41.4845962771032,0.75,39.3481673235966));
#43929=CARTESIAN_POINT('Origin',(34.7962928478066,4.95,45.3703427808264));
#43930=CARTESIAN_POINT('',(34.7962928478066,0.75,45.3703427808264));
#43931=CARTESIAN_POINT('',(34.7962928478066,4.95,45.3703427808264));
#43932=CARTESIAN_POINT('',(34.7962928478066,0.75,45.3703427808264));
#43933=CARTESIAN_POINT('Origin',(44.1641213368306,4.95,55.7743703375099));
#43934=CARTESIAN_POINT('',(44.1641213368306,0.75,55.7743703375099));
#43935=CARTESIAN_POINT('Origin',(28.1995939574892,4.75,14.6786847883499));
#43936=CARTESIAN_POINT('',(48.7590023146881,4.55,29.8631829059837));
#43937=CARTESIAN_POINT('',(28.0820369070308,4.55,14.8404881872249));
#43938=CARTESIAN_POINT('',(48.6705096178552,4.95,29.3044620073168));
#43939=CARTESIAN_POINT('Origin',(42.2496295308103,4.75,38.4823055959794));
#43940=CARTESIAN_POINT('',(43.4689350440559,4.55,37.1443358553582));
#43941=CARTESIAN_POINT('',(42.4114329296853,4.55,38.5998626464379));
#43942=CARTESIAN_POINT('',(42.9102141453889,4.95,37.2328285521912));
#43943=CARTESIAN_POINT('Origin',(28.3375315465646,4.75,26.3979413015218));
#43944=CARTESIAN_POINT('',(28.4550885970231,4.55,26.2361379026468));
#43945=CARTESIAN_POINT('Origin',(48.7590023146881,4.95,29.8631829059837));
#43946=CARTESIAN_POINT('',(48.7590023146881,0.75,29.8631829059837));
#43947=CARTESIAN_POINT('',(48.7590023146881,4.95,29.8631829059837));
#43948=CARTESIAN_POINT('',(48.7590023146881,0.75,29.8631829059837));
#43949=CARTESIAN_POINT('Origin',(43.4689350440559,4.95,37.1443358553582));
#43950=CARTESIAN_POINT('',(43.4689350440559,0.75,37.1443358553582));
#43951=CARTESIAN_POINT('',(43.4689350440559,4.95,37.1443358553582));
#43952=CARTESIAN_POINT('',(43.4689350440559,0.75,37.1443358553582));
#43953=CARTESIAN_POINT('Origin',(54.7951729653051,4.95,45.3733293874529));
#43954=CARTESIAN_POINT('',(54.7951729653051,0.75,45.3733293874529));
#43955=CARTESIAN_POINT('Origin',(29.8074276910276,4.75,8.12633133432707));
#43956=CARTESIAN_POINT('',(53.9024059794693,4.55,19.0730340959289));
#43957=CARTESIAN_POINT('',(29.7260803624124,4.55,8.30904042585558));
#43958=CARTESIAN_POINT('',(53.6996824536426,4.95,18.5449212556416));
#43959=CARTESIAN_POINT('Origin',(49.114504621422,4.75,29.3351179488144));
#43960=CARTESIAN_POINT('',(50.2417761917871,4.55,27.2949432147124));
#43961=CARTESIAN_POINT('',(49.2972137129505,4.55,29.4164652774295));
#43962=CARTESIAN_POINT('',(49.7136633514998,4.95,27.4976667405391));
#43963=CARTESIAN_POINT('Origin',(32.3789214496132,4.75,19.5608151376981));
#43964=CARTESIAN_POINT('',(32.4602687782284,4.55,19.3781060461696));
#43965=CARTESIAN_POINT('Origin',(53.9024059794693,4.95,19.0730340959289));
#43966=CARTESIAN_POINT('',(53.9024059794693,0.75,19.0730340959289));
#43967=CARTESIAN_POINT('',(53.9024059794693,4.95,19.0730340959289));
#43968=CARTESIAN_POINT('',(53.9024059794693,0.75,19.0730340959289));
#43969=CARTESIAN_POINT('Origin',(50.2417761917871,4.95,27.2949432147124));
#43970=CARTESIAN_POINT('',(50.2417761917871,0.75,27.2949432147124));
#43971=CARTESIAN_POINT('',(50.2417761917871,4.95,27.2949432147124));
#43972=CARTESIAN_POINT('',(50.2417761917871,0.75,27.2949432147124));
#43973=CARTESIAN_POINT('Origin',(63.0314125987835,4.95,32.9892562177736));
#43974=CARTESIAN_POINT('',(63.0314125987835,0.75,32.9892562177736));
#43975=CARTESIAN_POINT('Origin',(29.8722500170541,4.75,1.54454195710666));
#43976=CARTESIAN_POINT('',(56.6900158505068,4.55,7.44930217331019));
#43977=CARTESIAN_POINT('',(29.8306676788906,4.55,1.74017147725342));
#43978=CARTESIAN_POINT('',(56.3819214865404,4.95,6.97487845668956));
#43979=CARTESIAN_POINT('Origin',(54.073123968043,4.75,18.7988636478504));
#43980=CARTESIAN_POINT('',(54.818810633147,4.55,16.2526305799144));
#43981=CARTESIAN_POINT('',(54.2687534881898,4.55,18.840445986014));
#43982=CARTESIAN_POINT('',(54.3443869165264,4.95,16.5607249438809));
#43983=CARTESIAN_POINT('Origin',(34.7649133285038,4.75,12.1945112397288));
#43984=CARTESIAN_POINT('',(34.8064956666674,4.55,11.998881719582));
#43985=CARTESIAN_POINT('Origin',(56.6900158505068,4.95,7.44930217331019));
#43986=CARTESIAN_POINT('',(56.6900158505068,0.75,7.44930217331019));
#43987=CARTESIAN_POINT('',(56.6900158505068,4.95,7.44930217331019));
#43988=CARTESIAN_POINT('',(56.6900158505068,0.75,7.44930217331019));
#43989=CARTESIAN_POINT('Origin',(54.818810633147,4.95,16.2526305799144));
#43990=CARTESIAN_POINT('',(54.818810633147,0.75,16.2526305799144));
#43991=CARTESIAN_POINT('',(54.818810633147,4.95,16.2526305799144));
#43992=CARTESIAN_POINT('',(54.818810633147,0.75,16.2526305799144));
#43993=CARTESIAN_POINT('Origin',(68.5128770434203,4.95,19.1633942513631));
#43994=CARTESIAN_POINT('',(68.5128770434203,0.75,19.1633942513631));
#43995=CARTESIAN_POINT('Origin',(56.8,-4.75,32.75));
#43996=CARTESIAN_POINT('',(56.6,-4.95,4.9));
#43997=CARTESIAN_POINT('',(56.6,-4.95,-4.9));
#43998=CARTESIAN_POINT('',(56.6,-4.95,32.75));
#43999=CARTESIAN_POINT('',(57.,-4.55,-4.5));
#44000=CARTESIAN_POINT('',(59.4916666666667,-2.05833333333331,-2.0083333333333));
#44001=CARTESIAN_POINT('',(57.,-4.55,4.5));
#44002=CARTESIAN_POINT('',(57.,-4.55,32.75));
#44003=CARTESIAN_POINT('',(57.,-4.55,4.5));
#44004=CARTESIAN_POINT('Origin',(28.5,-4.75,4.7));
#44005=CARTESIAN_POINT('',(28.5,-4.55,4.5));
#44006=CARTESIAN_POINT('',(28.5,-4.95,4.9));
#44007=CARTESIAN_POINT('Origin',(0.,-4.95,70.));
#44008=CARTESIAN_POINT('',(35.5,-4.95,-4.9));
#44009=CARTESIAN_POINT('',(56.3819214865404,-4.95,6.97487845668957));
#44010=CARTESIAN_POINT('',(42.8608983648836,-4.95,4.10089627168932));
#44011=CARTESIAN_POINT('',(54.3443869165264,-4.95,16.5607249438808));
#44012=CARTESIAN_POINT('',(48.7130642520468,-4.95,43.0540151073797));
#44013=CARTESIAN_POINT('',(33.976330589733,-4.95,12.2313609231563));
#44014=CARTESIAN_POINT('',(53.6996824536426,-4.95,18.5449212556416));
#44015=CARTESIAN_POINT('',(47.4289077432382,-4.95,15.7529924754622));
#44016=CARTESIAN_POINT('',(49.7136633514998,-4.95,27.4976667405391));
#44017=CARTESIAN_POINT('',(39.6167959036373,-4.95,50.1756023296745));
#44018=CARTESIAN_POINT('',(37.0480704375971,-4.95,21.8585814588291));
#44019=CARTESIAN_POINT('',(48.6705096178552,-4.95,29.3044620073168));
#44020=CARTESIAN_POINT('',(48.2437400717089,-4.95,28.994395782384));
#44021=CARTESIAN_POINT('',(42.9102141453889,-4.95,37.2328285521913));
#44022=CARTESIAN_POINT('',(30.4693896641149,-4.95,54.3561544439719));
#44023=CARTESIAN_POINT('',(36.8203256386181,-4.95,32.8082655612112));
#44024=CARTESIAN_POINT('',(41.5142019647506,-4.95,38.7832571508621));
#44025=CARTESIAN_POINT('',(44.7996793395235,-4.95,42.4321494404731));
#44026=CARTESIAN_POINT('',(34.2313826750721,-4.95,45.3407370931789));
#44027=CARTESIAN_POINT('',(22.1407350082907,-4.95,56.2272051505292));
#44028=CARTESIAN_POINT('',(32.832945805333,-4.95,43.7876156044481));
#44029=CARTESIAN_POINT('',(32.5435244785437,-4.95,46.5670378541993));
#44030=CARTESIAN_POINT('',(37.1489690447714,-4.95,54.5439018343476));
#44031=CARTESIAN_POINT('',(24.0564755214562,-4.95,51.4670378541992));
#44032=CARTESIAN_POINT('',(15.0931125922873,-4.95,56.6420378541992));
#44033=CARTESIAN_POINT('',(25.1619200876839,-4.95,53.3817240078565));
#44034=CARTESIAN_POINT('',(22.1505388114683,-4.95,52.3156155498685));
#44035=CARTESIAN_POINT('',(25.9165221452752,-4.95,63.9061204576023));
#44036=CARTESIAN_POINT('',(12.8301849517758,-4.95,55.3439820947429));
#44037=CARTESIAN_POINT('',(9.34399712816784,-4.95,56.4767131834005));
#44038=CARTESIAN_POINT('',(14.433049324958,-4.95,60.2770913884107));
#44039=CARTESIAN_POINT('',(10.7894683082537,-4.95,55.7777498078328));
#44040=CARTESIAN_POINT('',(12.222372322617,-4.95,69.4109208284038));
#44041=CARTESIAN_POINT('',(1.04315373364462,-4.95,56.8021287478558));
#44042=CARTESIAN_POINT('',(4.515530696217,-4.95,56.4371672226504));
#44043=CARTESIAN_POINT('',(1.74435850513434,-4.95,63.4736465008489));
#44044=CARTESIAN_POINT('',(-1.04315373364469,-4.95,56.8021287478558));
#44045=CARTESIAN_POINT('',(-2.476057748008,-4.95,70.4352997684268));
#44046=CARTESIAN_POINT('',(-10.7894683082538,-4.95,55.7777498078328));
#44047=CARTESIAN_POINT('',(-0.040182167059801,-4.95,56.9075453073549));
#44048=CARTESIAN_POINT('',(-11.4906730797435,-4.95,62.4492675608259));
#44049=CARTESIAN_POINT('',(-12.8301849517758,-4.95,55.3439820947429));
#44050=CARTESIAN_POINT('',(-16.5961682855827,-4.95,66.9344870024768));
#44051=CARTESIAN_POINT('',(-22.1505388114683,-4.95,52.3156155498685));
#44052=CARTESIAN_POINT('',(-5.06424280483965,-4.95,57.8672896580878));
#44053=CARTESIAN_POINT('',(-23.7534031846505,-4.95,57.2487248435362));
#44054=CARTESIAN_POINT('',(-24.0564755214563,-4.95,51.4670378541992));
#44055=CARTESIAN_POINT('',(-28.6619200876839,-4.95,59.4439018343476));
#44056=CARTESIAN_POINT('',(-32.5435244785438,-4.95,46.5670378541992));
#44057=CARTESIAN_POINT('',(-11.1959982752574,-4.95,58.8920378541992));
#44058=CARTESIAN_POINT('',(-33.6489690447714,-4.95,48.4817240078565));
#44059=CARTESIAN_POINT('',(-34.2313826750722,-4.95,45.3407370931789));
#44060=CARTESIAN_POINT('',(-37.516860049845,-4.95,48.9896293827898));
#44061=CARTESIAN_POINT('',(-41.5142019647506,-4.95,38.7832571508621));
#44062=CARTESIAN_POINT('',(-18.7965832936425,-4.95,59.238292879144));
#44063=CARTESIAN_POINT('',(-40.1157650950115,-4.95,37.2301356621313));
#44064=CARTESIAN_POINT('',(-42.9102141453889,-4.95,37.2328285521912));
#44065=CARTESIAN_POINT('',(-42.4834445992427,-4.95,36.9227623272584));
#44066=CARTESIAN_POINT('',(-48.6705096178552,-4.95,29.3044620073167));
#44067=CARTESIAN_POINT('',(-27.8243560287988,-4.95,57.9967309186592));
#44068=CARTESIAN_POINT('',(-42.5806211110843,-4.95,24.8798990163367));
#44069=CARTESIAN_POINT('',(-49.7136633514998,-4.95,27.497666740539));
#44070=CARTESIAN_POINT('',(-43.4428886410953,-4.95,24.7057379603596));
#44071=CARTESIAN_POINT('',(-53.6996824536427,-4.95,18.5449212556415));
#44072=CARTESIAN_POINT('',(-37.7864810097963,-4.95,54.2865568890662));
#44073=CARTESIAN_POINT('',(-41.0340895397399,-4.95,12.9058359739315));
#44074=CARTESIAN_POINT('',(-54.3443869165264,-4.95,16.5607249438808));
#44075=CARTESIAN_POINT('',(-40.8233637948696,-4.95,13.6867427588806));
#44076=CARTESIAN_POINT('',(-56.3819214865404,-4.95,6.97487845668952));
#44077=CARTESIAN_POINT('',(-47.777461643367,-4.95,47.4556793106817));
#44078=CARTESIAN_POINT('',(-36.013865159747,-4.95,2.64551443596496));
#44079=CARTESIAN_POINT('',(-56.6,-4.95,4.9));
#44080=CARTESIAN_POINT('',(-35.5,-4.95,4.9));
#44081=CARTESIAN_POINT('',(-56.6,-4.95,-4.90000000000001));
#44082=CARTESIAN_POINT('',(-56.6,-4.95,37.25));
#44083=CARTESIAN_POINT('',(-28.5,-4.95,-4.90000000000001));
#44084=CARTESIAN_POINT('',(-56.3819214865404,-4.95,-6.97487845668956));
#44085=CARTESIAN_POINT('',(-28.6251158572306,-4.95,-1.07498728918034));
#44086=CARTESIAN_POINT('',(-54.3443869165264,-4.95,-16.5607249438809));
#44087=CARTESIAN_POINT('',(-62.9488467596999,-4.95,23.9200759101114));
#44088=CARTESIAN_POINT('',(-19.7405480820799,-4.95,-9.20545194064731));
#44089=CARTESIAN_POINT('',(-53.6996824536426,-4.95,-18.5449212556416));
#44090=CARTESIAN_POINT('',(-21.4188388515293,-4.95,-4.17256369802218));
#44091=CARTESIAN_POINT('',(-49.7136633514998,-4.95,-27.497666740539));
#44092=CARTESIAN_POINT('',(-65.6268647953462,-4.95,8.24396889288556));
#44093=CARTESIAN_POINT('',(-11.0380015458883,-4.95,-10.2781526813891));
#44094=CARTESIAN_POINT('',(-48.6705096178552,-4.95,-29.3044620073167));
#44095=CARTESIAN_POINT('',(-14.9567620013786,-4.95,-4.80999058550712));
#44096=CARTESIAN_POINT('',(-42.9102141453889,-4.95,-37.2328285521912));
#44097=CARTESIAN_POINT('',(-63.7563677344453,-4.95,-8.54055964084878));
#44098=CARTESIAN_POINT('',(-3.53334756828769,-4.95,-8.6238603643343));
#44099=CARTESIAN_POINT('',(-41.5142019647506,-4.95,-38.7832571508621));
#44100=CARTESIAN_POINT('',(-9.9914130016339,-4.95,-3.77365322610516));
#44101=CARTESIAN_POINT('',(-34.2313826750721,-4.95,-45.3407370931789));
#44102=CARTESIAN_POINT('',(-56.9490013461803,-4.95,-24.885701364897));
#44103=CARTESIAN_POINT('',(1.97532053255655,-4.95,-5.12911939008019));
#44104=CARTESIAN_POINT('',(-32.5435244785437,-4.95,-46.5670378541993));
#44105=CARTESIAN_POINT('',(-6.83807991231607,-4.95,-2.04390183434758));
#44106=CARTESIAN_POINT('',(-24.0564755214562,-4.95,-51.4670378541992));
#44107=CARTESIAN_POINT('',(-45.4040017247427,-4.95,-39.1420378541993));
#44108=CARTESIAN_POINT('',(5.14896904477143,-4.95,-0.881724007856505));
#44109=CARTESIAN_POINT('',(-22.1505388114683,-4.95,-52.3156155498685));
#44110=CARTESIAN_POINT('',(-5.34403831503861,-4.95,-0.590525654479128));
#44111=CARTESIAN_POINT('',(-12.8301849517758,-4.95,-55.3439820947429));
#44112=CARTESIAN_POINT('',(-29.9164809584044,-4.95,-49.7923079865237));
#44113=CARTESIAN_POINT('',(6.13943450527853,-4.95,3.03850341471246));
#44114=CARTESIAN_POINT('',(-10.7894683082537,-4.95,-55.7777498078328));
#44115=CARTESIAN_POINT('',(-4.94546314399545,-4.95,-0.175754802720606));
#44116=CARTESIAN_POINT('',(-1.04315373364464,-4.95,-56.8021287478558));
#44117=CARTESIAN_POINT('',(-11.7924398748386,-4.95,-55.6723332483337));
#44118=CARTESIAN_POINT('',(5.5325506734872,-4.95,5.76151952483431));
#44119=CARTESIAN_POINT('',(1.04315373364466,-4.95,-56.8021287478558));
#44120=CARTESIAN_POINT('',(-4.80085143061363,-4.95,-1.20013374274361));
#44121=CARTESIAN_POINT('',(10.7894683082537,-4.95,-55.7777498078327));
#44122=CARTESIAN_POINT('',(7.31709134568138,-4.95,-56.1427113330381));
#44123=CARTESIAN_POINT('',(4.21376390112187,-4.95,6.78589846485731));
#44124=CARTESIAN_POINT('',(12.8301849517758,-4.95,-55.343982094743));
#44125=CARTESIAN_POINT('',(-3.9763155446539,-4.95,-3.61889219935362));
#44126=CARTESIAN_POINT('',(22.1505388114683,-4.95,-52.3156155498685));
#44127=CARTESIAN_POINT('',(25.6367266350762,-4.95,-51.1828844612109));
#44128=CARTESIAN_POINT('',(3.18091935441398,-4.95,6.06686995958694));
#44129=CARTESIAN_POINT('',(24.0564755214563,-4.95,-51.4670378541992));
#44130=CARTESIAN_POINT('',(-1.64896904477142,-4.95,-6.94390183434757));
#44131=CARTESIAN_POINT('',(32.5435244785437,-4.95,-46.5670378541992));
#44132=CARTESIAN_POINT('',(41.5068874077127,-4.95,-41.3920378541992));
#44133=CARTESIAN_POINT('',(3.33807991231607,-4.95,4.01827599214349));
#44134=CARTESIAN_POINT('',(34.2313826750722,-4.95,-45.3407370931789));
#44135=CARTESIAN_POINT('',(2.70859371195544,-4.95,-10.331133168422));
#44136=CARTESIAN_POINT('',(41.5142019647506,-4.95,-38.7832571508621));
#44137=CARTESIAN_POINT('',(53.604849631532,-4.95,-27.8967890935119));
#44138=CARTESIAN_POINT('',(5.30749875712191,-4.95,1.42836055223659));
#44139=CARTESIAN_POINT('',(42.9102141453889,-4.95,-37.2328285521912));
#44140=CARTESIAN_POINT('',(9.19646652891232,-4.95,-12.7383571303816));
#44141=CARTESIAN_POINT('',(48.6705096178551,-4.95,-29.3044620073167));
#44142=CARTESIAN_POINT('',(61.1113340991292,-4.95,-12.181136115536));
#44143=CARTESIAN_POINT('',(9.29364304075393,-4.95,-0.695493819459823));
#44144=CARTESIAN_POINT('',(49.7136633514998,-4.95,-27.4976667405391));
#44145=CARTESIAN_POINT('',(17.4328197493865,-4.95,-13.1253091829197));
#44146=CARTESIAN_POINT('',(53.6996824536427,-4.95,-18.5449212556416));
#44147=CARTESIAN_POINT('',(63.7965499015051,-4.95,4.13301433349386));
#44148=CARTESIAN_POINT('',(15.0240206480311,-4.95,-1.32540719649159));
#44149=CARTESIAN_POINT('',(54.3443869165264,-4.95,-16.5607249438808));
#44150=CARTESIAN_POINT('',(26.5875812872166,-4.95,-10.6608337763716));
#44151=CARTESIAN_POINT('',(56.3819214865404,-4.95,-6.97487845668953));
#44152=CARTESIAN_POINT('',(62.01324415102,-4.95,19.5184117068093));
#44153=CARTESIAN_POINT('',(21.778082652094,-4.95,0.380394546543994));
#44154=CARTESIAN_POINT('',(-12.4,-4.95,-2.95));
#44155=CARTESIAN_POINT('',(-9.56543778402222,-4.95,-2.95));
#44156=CARTESIAN_POINT('',(6.,-4.95,-2.95));
#44157=CARTESIAN_POINT('',(-12.4,-4.95,2.95));
#44158=CARTESIAN_POINT('',(-12.4,-4.95,33.725));
#44159=CARTESIAN_POINT('',(-9.56543778402222,-4.95,2.95));
#44160=CARTESIAN_POINT('',(-6.,-4.95,2.95));
#44161=CARTESIAN_POINT('',(9.56543778402222,-4.95,2.95));
#44162=CARTESIAN_POINT('Origin',(0.,-4.95,0.));
#44163=CARTESIAN_POINT('',(12.4,-4.95,2.95));
#44164=CARTESIAN_POINT('',(-6.,-4.95,2.95));
#44165=CARTESIAN_POINT('',(12.4,-4.95,-2.95));
#44166=CARTESIAN_POINT('',(12.4,-4.95,36.275));
#44167=CARTESIAN_POINT('',(9.56543778402222,-4.95,-2.95));
#44168=CARTESIAN_POINT('',(6.,-4.95,-2.95));
#44169=CARTESIAN_POINT('Origin',(0.,-4.95,0.));
#44170=CARTESIAN_POINT('Origin',(35.5,-4.75,-4.7));
#44171=CARTESIAN_POINT('',(35.5,-4.55,-4.5));
#44172=CARTESIAN_POINT('Origin',(62.2088736711667,-4.75,19.4768293686457));
#44173=CARTESIAN_POINT('',(54.818810633147,-4.55,-16.2526305799144));
#44174=CARTESIAN_POINT('',(54.3443869165264,-4.95,-16.5607249438808));
#44175=CARTESIAN_POINT('',(56.6900158505068,-4.55,-7.44930217331016));
#44176=CARTESIAN_POINT('',(62.4045031913135,-4.55,19.4352470304822));
#44177=CARTESIAN_POINT('',(56.6900158505068,-4.55,-7.44930217331016));
#44178=CARTESIAN_POINT('Origin',(26.6291636253801,-4.75,-10.4652042562249));
#44179=CARTESIAN_POINT('',(26.6707459635437,-4.55,-10.2695747360781));
#44180=CARTESIAN_POINT('Origin',(21.7365003139304,-4.75,0.184765026397232));
#44181=CARTESIAN_POINT('',(21.6949179757669,-4.55,-0.0108644937495309));
#44182=CARTESIAN_POINT('Origin',(63.9792589930336,-4.75,4.05166700487871));
#44183=CARTESIAN_POINT('',(50.2417761917872,-4.55,-27.2949432147123));
#44184=CARTESIAN_POINT('',(49.7136633514998,-4.95,-27.4976667405391));
#44185=CARTESIAN_POINT('',(53.9024059794694,-4.55,-19.0730340959289));
#44186=CARTESIAN_POINT('',(64.1619680845621,-4.55,3.97031967626356));
#44187=CARTESIAN_POINT('',(53.9024059794694,-4.55,-19.0730340959289));
#44188=CARTESIAN_POINT('Origin',(17.5141670780017,-4.75,-12.9426000913912));
#44189=CARTESIAN_POINT('',(17.5955144066168,-4.55,-12.7598909998626));
#44190=CARTESIAN_POINT('Origin',(14.942673319416,-4.75,-1.50811628802011));
#44191=CARTESIAN_POINT('',(14.8613259908008,-4.55,-1.69082537954862));
#44192=CARTESIAN_POINT('Origin',(53.9024059794694,-4.95,-19.0730340959289));
#44193=CARTESIAN_POINT('',(53.9024059794694,-0.75,-19.0730340959289));
#44194=CARTESIAN_POINT('',(53.9024059794694,-4.95,-19.0730340959289));
#44195=CARTESIAN_POINT('',(66.6920423864658,-0.75,-24.7673470989901));
#44196=CARTESIAN_POINT('Origin',(50.2417761917872,-4.95,-27.2949432147123));
#44197=CARTESIAN_POINT('',(50.2417761917872,-0.75,-27.2949432147123));
#44198=CARTESIAN_POINT('',(50.2417761917872,-4.95,-27.2949432147123));
#44199=CARTESIAN_POINT('',(53.9024059794694,-0.75,-19.0730340959289));
#44200=CARTESIAN_POINT('Origin',(61.2731374980041,-4.75,-12.2986931659945));
#44201=CARTESIAN_POINT('',(43.4689350440559,-4.55,-37.1443358553582));
#44202=CARTESIAN_POINT('',(42.9102141453889,-4.95,-37.2328285521912));
#44203=CARTESIAN_POINT('',(48.7590023146881,-4.55,-29.8631829059837));
#44204=CARTESIAN_POINT('',(61.4349408968791,-4.55,-12.416250216453));
#44205=CARTESIAN_POINT('',(48.7590023146881,-4.55,-29.8631829059837));
#44206=CARTESIAN_POINT('Origin',(9.31402357937082,-4.75,-12.5765537315066));
#44207=CARTESIAN_POINT('',(9.43158062982931,-4.55,-12.4147503326316));
#44208=CARTESIAN_POINT('Origin',(9.17608599029544,-4.75,-0.85729721833481));
#44209=CARTESIAN_POINT('',(9.05852893983695,-4.55,-1.0191006172098));
#44210=CARTESIAN_POINT('Origin',(53.7386757528038,-4.75,-28.0454180586074));
#44211=CARTESIAN_POINT('',(34.7962928478066,-4.55,-45.3703427808263));
#44212=CARTESIAN_POINT('',(34.2313826750721,-4.95,-45.3407370931789));
#44213=CARTESIAN_POINT('',(41.4845962771032,-4.55,-39.3481673235966));
#44214=CARTESIAN_POINT('',(53.8725018740756,-4.55,-28.1940470237028));
#44215=CARTESIAN_POINT('',(41.4845962771032,-4.55,-39.3481673235966));
#44216=CARTESIAN_POINT('Origin',(2.85722267705093,-4.75,-10.1973070471502));
#44217=CARTESIAN_POINT('',(3.00585164214641,-4.55,-10.0634809258784));
#44218=CARTESIAN_POINT('Origin',(5.15886979202643,-4.75,1.29453443096482));
#44219=CARTESIAN_POINT('',(5.01024082693095,-4.55,1.16070830969305));
#44220=CARTESIAN_POINT('Origin',(41.4845962771032,-4.95,-39.3481673235966));
#44221=CARTESIAN_POINT('',(41.4845962771032,-0.75,-39.3481673235966));
#44222=CARTESIAN_POINT('',(41.4845962771032,-4.95,-39.3481673235966));
#44223=CARTESIAN_POINT('',(50.8524247661272,-0.75,-49.7521948802801));
#44224=CARTESIAN_POINT('Origin',(34.7962928478066,-4.95,-45.3703427808263));
#44225=CARTESIAN_POINT('',(34.7962928478066,-0.75,-45.3703427808263));
#44226=CARTESIAN_POINT('',(34.7962928478066,-4.95,-45.3703427808263));
#44227=CARTESIAN_POINT('',(41.4845962771032,-0.75,-39.3481673235966));
#44228=CARTESIAN_POINT('Origin',(41.6068874077127,-4.75,-41.5652429349561));
#44229=CARTESIAN_POINT('',(24.60288568297,-4.55,-51.613448015713));
#44230=CARTESIAN_POINT('',(24.0564755214563,-4.95,-51.4670378541992));
#44231=CARTESIAN_POINT('',(32.39711431703,-4.55,-47.113448015713));
#44232=CARTESIAN_POINT('',(41.7068874077127,-4.55,-41.738448015713));
#44233=CARTESIAN_POINT('',(32.39711431703,-4.55,-47.113448015713));
#44234=CARTESIAN_POINT('Origin',(-1.47576396401454,-4.75,-6.84390183434757));
#44235=CARTESIAN_POINT('',(-1.30255888325765,-4.55,-6.74390183434757));
#44236=CARTESIAN_POINT('Origin',(3.16487483155919,-4.75,3.91827599214349));
#44237=CARTESIAN_POINT('',(2.9916697508023,-4.55,3.8182759921435));
#44238=CARTESIAN_POINT('Origin',(25.6985300339512,-4.75,-51.3730957644699));
#44239=CARTESIAN_POINT('',(13.3342143560438,-4.55,-55.600797903511));
#44240=CARTESIAN_POINT('',(12.8301849517758,-4.95,-55.343982094743));
#44241=CARTESIAN_POINT('',(21.8937230027002,-4.55,-52.8196449541365));
#44242=CARTESIAN_POINT('',(25.7603334328262,-4.55,-51.563307067729));
#44243=CARTESIAN_POINT('',(21.8937230027002,-4.55,-52.8196449541365));
#44244=CARTESIAN_POINT('Origin',(-3.78610424139487,-4.75,-3.55708880047863));
#44245=CARTESIAN_POINT('',(-3.59589293813584,-4.55,-3.49528540160364));
#44246=CARTESIAN_POINT('Origin',(2.99070805115495,-4.75,6.00506656071195));
#44247=CARTESIAN_POINT('',(2.80049674789591,-4.55,5.94326316183696));
#44248=CARTESIAN_POINT('Origin',(21.8937230027002,-4.95,-52.8196449541365));
#44249=CARTESIAN_POINT('',(21.8937230027002,-0.75,-52.8196449541365));
#44250=CARTESIAN_POINT('',(21.8937230027002,-4.95,-52.8196449541365));
#44251=CARTESIAN_POINT('',(26.2199609239495,-0.75,-66.1344361822686));
#44252=CARTESIAN_POINT('Origin',(13.3342143560438,-4.95,-55.600797903511));
#44253=CARTESIAN_POINT('',(13.3342143560438,-0.75,-55.600797903511));
#44254=CARTESIAN_POINT('',(13.3342143560438,-4.95,-55.600797903511));
#44255=CARTESIAN_POINT('',(21.8937230027002,-0.75,-52.8196449541365));
#44256=CARTESIAN_POINT('Origin',(4.01485952204822,-4.75,6.76499277220378));
#44257=CARTESIAN_POINT('',(10.4334709354135,-4.55,-56.2173699512871));
#44258=CARTESIAN_POINT('',(19.4842239220056,-14.7194604253764,-45.0406208236431));
#44259=CARTESIAN_POINT('',(3.81595514297456,-4.55,6.74408707955025));
#44260=CARTESIAN_POINT('Origin',(7.33799703833491,-4.75,-56.3416157121117));
#44261=CARTESIAN_POINT('',(1.48277387709903,-4.55,-57.158126120696));
#44262=CARTESIAN_POINT('',(7.35890273098844,-4.55,-56.5405200911854));
#44263=CARTESIAN_POINT('',(1.04315373364466,-4.95,-56.8021287478558));
#44264=CARTESIAN_POINT('Origin',(-4.60194705153997,-4.75,-1.17922805009007));
#44265=CARTESIAN_POINT('',(-4.40304267246632,-4.55,-1.15832235743654));
#44266=CARTESIAN_POINT('Origin',(-11.8133455674921,-4.75,-55.8712376274073));
#44267=CARTESIAN_POINT('',(-10.4334709354135,-4.55,-56.2173699512871));
#44268=CARTESIAN_POINT('',(-10.7894683082537,-4.95,-55.7777498078328));
#44269=CARTESIAN_POINT('',(-1.48277387709901,-4.55,-57.158126120696));
#44270=CARTESIAN_POINT('',(-11.8342512601456,-4.55,-56.070142006481));
#44271=CARTESIAN_POINT('',(-1.48277387709901,-4.55,-57.158126120696));
#44272=CARTESIAN_POINT('Origin',(-4.74655876492179,-4.75,-0.196660495374136));
#44273=CARTESIAN_POINT('',(-4.54765438584814,-4.55,-0.217566188027667));
#44274=CARTESIAN_POINT('Origin',(5.33364629441355,-4.75,5.78242521748784));
#44275=CARTESIAN_POINT('',(5.13474191533989,-4.55,5.80333091014137));
#44276=CARTESIAN_POINT('Origin',(-29.9782843572794,-4.75,-49.9825192897827));
#44277=CARTESIAN_POINT('',(-21.8937230027002,-4.55,-52.8196449541365));
#44278=CARTESIAN_POINT('',(-22.1505388114683,-4.95,-52.3156155498685));
#44279=CARTESIAN_POINT('',(-13.3342143560438,-4.55,-55.600797903511));
#44280=CARTESIAN_POINT('',(-30.0400877561544,-4.55,-50.1727305930417));
#44281=CARTESIAN_POINT('',(-13.3342143560438,-4.55,-55.600797903511));
#44282=CARTESIAN_POINT('Origin',(-5.15382701177957,-4.75,-0.652329053354118));
#44283=CARTESIAN_POINT('',(-4.96361570852054,-4.55,-0.714132452229108));
#44284=CARTESIAN_POINT('Origin',(5.9492232020195,-4.75,3.10030681358745));
#44285=CARTESIAN_POINT('',(5.75901189876047,-4.55,3.16211021246244));
#44286=CARTESIAN_POINT('Origin',(-13.3342143560438,-4.95,-55.600797903511));
#44287=CARTESIAN_POINT('',(-13.3342143560438,-0.75,-55.600797903511));
#44288=CARTESIAN_POINT('',(-13.3342143560438,-4.95,-55.600797903511));
#44289=CARTESIAN_POINT('',(-17.6604522772931,-0.75,-68.9155891316432));
#44290=CARTESIAN_POINT('Origin',(-21.8937230027002,-4.95,-52.8196449541365));
#44291=CARTESIAN_POINT('',(-21.8937230027002,-0.75,-52.8196449541365));
#44292=CARTESIAN_POINT('',(-21.8937230027002,-4.95,-52.8196449541365));
#44293=CARTESIAN_POINT('',(-13.3342143560438,-0.75,-55.600797903511));
#44294=CARTESIAN_POINT('Origin',(-45.5040017247427,-4.75,-39.3152429349561));
#44295=CARTESIAN_POINT('',(-32.39711431703,-4.55,-47.113448015713));
#44296=CARTESIAN_POINT('',(-32.5435244785437,-4.95,-46.5670378541992));
#44297=CARTESIAN_POINT('',(-24.60288568297,-4.55,-51.613448015713));
#44298=CARTESIAN_POINT('',(-45.6040017247427,-4.55,-39.488448015713));
#44299=CARTESIAN_POINT('',(-24.60288568297,-4.55,-51.613448015713));
#44300=CARTESIAN_POINT('Origin',(-6.66487483155918,-4.75,-2.14390183434758));
#44301=CARTESIAN_POINT('',(-6.49166975080229,-4.55,-2.24390183434758));
#44302=CARTESIAN_POINT('Origin',(4.97576396401454,-4.75,-0.781724007856504));
#44303=CARTESIAN_POINT('',(4.80255888325765,-4.55,-0.681724007856502));
#44304=CARTESIAN_POINT('Origin',(-57.082827467452,-4.75,-25.0343303299925));
#44305=CARTESIAN_POINT('',(-41.4845962771032,-4.55,-39.3481673235966));
#44306=CARTESIAN_POINT('',(-41.5142019647506,-4.95,-38.7832571508621));
#44307=CARTESIAN_POINT('',(-34.7962928478066,-4.55,-45.3703427808263));
#44308=CARTESIAN_POINT('',(-57.2166535887238,-4.55,-25.182959295088));
#44309=CARTESIAN_POINT('',(-34.7962928478066,-4.55,-45.3703427808263));
#44310=CARTESIAN_POINT('Origin',(-9.84278403653842,-4.75,-3.90747934737692));
#44311=CARTESIAN_POINT('',(-9.69415507144295,-4.55,-4.04130546864869));
#44312=CARTESIAN_POINT('Origin',(1.82669156746108,-4.75,-4.99529326880842));
#44313=CARTESIAN_POINT('',(1.6780626023656,-4.55,-4.86146714753665));
#44314=CARTESIAN_POINT('Origin',(-34.7962928478066,-4.95,-45.3703427808263));
#44315=CARTESIAN_POINT('',(-34.7962928478066,-0.75,-45.3703427808263));
#44316=CARTESIAN_POINT('',(-34.7962928478066,-4.95,-45.3703427808263));
#44317=CARTESIAN_POINT('',(-44.1641213368306,-0.75,-55.7743703375099));
#44318=CARTESIAN_POINT('Origin',(-41.4845962771032,-4.95,-39.3481673235966));
#44319=CARTESIAN_POINT('',(-41.4845962771032,-0.75,-39.3481673235966));
#44320=CARTESIAN_POINT('',(-41.4845962771032,-4.95,-39.3481673235966));
#44321=CARTESIAN_POINT('',(-34.7962928478066,-0.75,-45.3703427808263));
#44322=CARTESIAN_POINT('Origin',(-63.9181711333203,-4.75,-8.65811669130728));
#44323=CARTESIAN_POINT('',(-48.7590023146881,-4.55,-29.8631829059837));
#44324=CARTESIAN_POINT('',(-48.6705096178552,-4.95,-29.3044620073167));
#44325=CARTESIAN_POINT('',(-43.4689350440559,-4.55,-37.1443358553582));
#44326=CARTESIAN_POINT('',(-64.0799745321953,-4.55,-8.77567374176577));
#44327=CARTESIAN_POINT('',(-43.4689350440559,-4.55,-37.1443358553582));
#44328=CARTESIAN_POINT('Origin',(-14.8392049509201,-4.75,-4.97179398438211));
#44329=CARTESIAN_POINT('',(-14.7216479004616,-4.55,-5.1335973832571));
#44330=CARTESIAN_POINT('Origin',(-3.65090461874619,-4.75,-8.46205696545931));
#44331=CARTESIAN_POINT('',(-3.76846166920468,-4.55,-8.30025356658432));
#44332=CARTESIAN_POINT('Origin',(-65.8095738868747,-4.75,8.1626215642704));
#44333=CARTESIAN_POINT('',(-53.9024059794693,-4.55,-19.0730340959289));
#44334=CARTESIAN_POINT('',(-53.6996824536426,-4.95,-18.5449212556416));
#44335=CARTESIAN_POINT('',(-50.2417761917871,-4.55,-27.2949432147123));
#44336=CARTESIAN_POINT('',(-65.9922829784032,-4.55,8.08127423565524));
#44337=CARTESIAN_POINT('',(-50.2417761917871,-4.55,-27.2949432147123));
#44338=CARTESIAN_POINT('Origin',(-21.3374915229142,-4.75,-4.3552727895507));
#44339=CARTESIAN_POINT('',(-21.256144194299,-4.55,-4.53798188107922));
#44340=CARTESIAN_POINT('Origin',(-11.1193488745035,-4.75,-10.0954435898605));
#44341=CARTESIAN_POINT('',(-11.2006962031186,-4.55,-9.91273449833203));
#44342=CARTESIAN_POINT('Origin',(-50.2417761917871,-4.95,-27.2949432147123));
#44343=CARTESIAN_POINT('',(-50.2417761917871,-0.75,-27.2949432147123));
#44344=CARTESIAN_POINT('',(-50.2417761917871,-4.95,-27.2949432147123));
#44345=CARTESIAN_POINT('',(-63.0314125987836,-0.75,-32.9892562177735));
#44346=CARTESIAN_POINT('Origin',(-53.9024059794693,-4.95,-19.0730340959289));
#44347=CARTESIAN_POINT('',(-53.9024059794693,-0.75,-19.0730340959289));
#44348=CARTESIAN_POINT('',(-53.9024059794693,-4.95,-19.0730340959289));
#44349=CARTESIAN_POINT('',(-50.2417761917871,-0.75,-27.2949432147123));
#44350=CARTESIAN_POINT('Origin',(-63.1444762798466,-4.75,23.8784935719478));
#44351=CARTESIAN_POINT('',(-56.6900158505068,-4.55,-7.44930217331018));
#44352=CARTESIAN_POINT('',(-56.3819214865404,-4.95,-6.97487845668956));
#44353=CARTESIAN_POINT('',(-54.818810633147,-4.55,-16.2526305799144));
#44354=CARTESIAN_POINT('',(-63.3401057999934,-4.55,23.8369112337843));
#44355=CARTESIAN_POINT('',(-54.818810633147,-4.55,-16.2526305799144));
#44356=CARTESIAN_POINT('Origin',(-28.5835335190671,-4.75,-1.27061680932709));
#44357=CARTESIAN_POINT('',(-28.5419511809035,-4.55,-1.46624632947385));
#44358=CARTESIAN_POINT('Origin',(-19.7821304202435,-4.75,-9.00982242050055));
#44359=CARTESIAN_POINT('',(-19.823712758407,-4.55,-8.81419290035379));
#44360=CARTESIAN_POINT('Origin',(-56.8,-4.75,37.25));
#44361=CARTESIAN_POINT('',(-57.,-4.55,4.49999999999999));
#44362=CARTESIAN_POINT('',(-56.6,-4.95,4.9));
#44363=CARTESIAN_POINT('',(-57.,-4.55,-4.50000000000001));
#44364=CARTESIAN_POINT('',(-57.,-4.55,37.25));
#44365=CARTESIAN_POINT('',(-57.,-4.55,-4.50000000000001));
#44366=CARTESIAN_POINT('Origin',(-35.5,-4.75,4.7));
#44367=CARTESIAN_POINT('',(-35.5,-4.55,4.5));
#44368=CARTESIAN_POINT('Origin',(-28.5,-4.75,-4.70000000000001));
#44369=CARTESIAN_POINT('',(-28.5,-4.55,-4.5));
#44370=CARTESIAN_POINT('Origin',(-57.,-4.95,-4.50000000000001));
#44371=CARTESIAN_POINT('',(-57.,-0.75,-4.50000000000001));
#44372=CARTESIAN_POINT('',(-57.,-4.95,-4.50000000000001));
#44373=CARTESIAN_POINT('',(-71.,-0.75,-4.50000000000001));
#44374=CARTESIAN_POINT('Origin',(-57.,-4.95,4.49999999999999));
#44375=CARTESIAN_POINT('',(-57.,-0.75,4.49999999999999));
#44376=CARTESIAN_POINT('',(-57.,-4.95,4.49999999999999));
#44377=CARTESIAN_POINT('',(-57.,-0.75,-4.50000000000001));
#44378=CARTESIAN_POINT('Origin',(-47.9730911635137,-4.75,47.4972616488453));
#44379=CARTESIAN_POINT('',(-54.818810633147,-4.55,16.2526305799144));
#44380=CARTESIAN_POINT('',(-54.3443869165264,-4.95,16.5607249438808));
#44381=CARTESIAN_POINT('',(-56.6900158505068,-4.55,7.44930217331014));
#44382=CARTESIAN_POINT('',(-48.1687206836605,-4.55,47.5388439870088));
#44383=CARTESIAN_POINT('',(-56.6900158505068,-4.55,7.44930217331014));
#44384=CARTESIAN_POINT('Origin',(-40.8649461330331,-4.75,13.4911132387338));
#44385=CARTESIAN_POINT('',(-40.9065284711967,-4.55,13.2954837185871));
#44386=CARTESIAN_POINT('Origin',(-35.9722828215834,-4.75,2.84114395611173));
#44387=CARTESIAN_POINT('',(-35.9307004834199,-4.55,3.03677347625849));
#44388=CARTESIAN_POINT('Origin',(-37.9691901013248,-4.75,54.3679042176813));
#44389=CARTESIAN_POINT('',(-50.2417761917872,-4.55,27.2949432147123));
#44390=CARTESIAN_POINT('',(-49.7136633514998,-4.95,27.497666740539));
#44391=CARTESIAN_POINT('',(-53.9024059794694,-4.55,19.0730340959289));
#44392=CARTESIAN_POINT('',(-38.1518991928533,-4.55,54.4492515462965));
#44393=CARTESIAN_POINT('',(-53.9024059794694,-4.55,19.0730340959289));
#44394=CARTESIAN_POINT('Origin',(-43.5242359697105,-4.75,24.5230288688311));
#44395=CARTESIAN_POINT('',(-43.6055832983256,-4.55,24.3403197773026));
#44396=CARTESIAN_POINT('Origin',(-40.9527422111248,-4.75,13.08854506546));
#44397=CARTESIAN_POINT('',(-40.8713948825096,-4.55,13.2712541569886));
#44398=CARTESIAN_POINT('Origin',(-53.9024059794694,-4.95,19.0730340959289));
#44399=CARTESIAN_POINT('',(-53.9024059794694,-0.75,19.0730340959289));
#44400=CARTESIAN_POINT('',(-53.9024059794694,-4.95,19.0730340959289));
#44401=CARTESIAN_POINT('',(-66.6920423864658,-0.75,24.7673470989901));
#44402=CARTESIAN_POINT('Origin',(-50.2417761917872,-4.95,27.2949432147123));
#44403=CARTESIAN_POINT('',(-50.2417761917872,-0.75,27.2949432147123));
#44404=CARTESIAN_POINT('',(-50.2417761917872,-4.95,27.2949432147123));
#44405=CARTESIAN_POINT('',(-53.9024059794694,-0.75,19.0730340959289));
#44406=CARTESIAN_POINT('Origin',(-27.9861594276738,-4.75,58.1142879691177));
#44407=CARTESIAN_POINT('',(-43.4689350440559,-4.55,37.1443358553582));
#44408=CARTESIAN_POINT('',(-42.9102141453889,-4.95,37.2328285521912));
#44409=CARTESIAN_POINT('',(-48.7590023146881,-4.55,29.8631829059837));
#44410=CARTESIAN_POINT('',(-28.1479628265488,-4.55,58.2318450195762));
#44411=CARTESIAN_POINT('',(-48.7590023146881,-4.55,29.8631829059837));
#44412=CARTESIAN_POINT('Origin',(-42.6010016497012,-4.75,36.7609589283835));
#44413=CARTESIAN_POINT('',(-42.7185587001597,-4.55,36.5991555295085));
#44414=CARTESIAN_POINT('Origin',(-42.4630640606258,-4.75,25.0417024152116));
#44415=CARTESIAN_POINT('',(-42.3455070101673,-4.55,25.2035058140866));
#44416=CARTESIAN_POINT('Origin',(-18.9304094149142,-4.75,59.3869218442395));
#44417=CARTESIAN_POINT('',(-34.7962928478067,-4.55,45.3703427808263));
#44418=CARTESIAN_POINT('',(-34.2313826750722,-4.95,45.3407370931789));
#44419=CARTESIAN_POINT('',(-41.4845962771032,-4.55,39.3481673235966));
#44420=CARTESIAN_POINT('',(-19.064235536186,-4.55,59.535550809335));
#44421=CARTESIAN_POINT('',(-41.4845962771032,-4.55,39.3481673235966));
#44422=CARTESIAN_POINT('Origin',(-37.6654890149405,-4.75,48.855803261518));
#44423=CARTESIAN_POINT('',(-37.814117980036,-4.55,48.7219771402463));
#44424=CARTESIAN_POINT('Origin',(-39.967136129916,-4.75,37.363961783403));
#44425=CARTESIAN_POINT('',(-39.8185071648205,-4.55,37.4977879046748));
#44426=CARTESIAN_POINT('Origin',(-41.4845962771032,-4.95,39.3481673235966));
#44427=CARTESIAN_POINT('',(-41.4845962771032,-0.75,39.3481673235966));
#44428=CARTESIAN_POINT('',(-41.4845962771032,-4.95,39.3481673235966));
#44429=CARTESIAN_POINT('',(-50.8524247661272,-0.75,49.7521948802801));
#44430=CARTESIAN_POINT('Origin',(-34.7962928478067,-4.95,45.3703427808263));
#44431=CARTESIAN_POINT('',(-34.7962928478067,-0.75,45.3703427808263));
#44432=CARTESIAN_POINT('',(-34.7962928478067,-4.95,45.3703427808263));
#44433=CARTESIAN_POINT('',(-41.4845962771032,-0.75,39.3481673235966));
#44434=CARTESIAN_POINT('Origin',(-11.2959982752574,-4.75,59.0652429349561));
#44435=CARTESIAN_POINT('',(-24.6028856829701,-4.55,51.613448015713));
#44436=CARTESIAN_POINT('',(-22.9547507919904,-5.75651847792408,51.1718316026574));
#44437=CARTESIAN_POINT('',(-32.39711431703,-4.55,47.113448015713));
#44438=CARTESIAN_POINT('',(-11.3959982752574,-4.55,59.238448015713));
#44439=CARTESIAN_POINT('',(-32.39711431703,-4.55,47.113448015713));
#44440=CARTESIAN_POINT('Origin',(-33.4757639640146,-4.75,48.5817240078565));
#44441=CARTESIAN_POINT('',(-33.3025588832577,-4.55,48.6817240078565));
#44442=CARTESIAN_POINT('Origin',(-28.8351251684408,-4.75,59.3439018343476));
#44443=CARTESIAN_POINT('',(-29.0083302491977,-4.55,59.2439018343476));
#44444=CARTESIAN_POINT('Origin',(-5.12604620371464,-4.75,58.0575009613468));
#44445=CARTESIAN_POINT('',(-13.3342143560438,-4.55,55.600797903511));
#44446=CARTESIAN_POINT('',(-12.8301849517758,-4.95,55.3439820947429));
#44447=CARTESIAN_POINT('',(-21.8937230027002,-4.55,52.8196449541365));
#44448=CARTESIAN_POINT('',(-5.18784960258963,-4.55,58.2477122646058));
#44449=CARTESIAN_POINT('',(-21.8937230027002,-4.55,52.8196449541365));
#44450=CARTESIAN_POINT('Origin',(-16.7863795888417,-4.75,66.8726836036018));
#44451=CARTESIAN_POINT('',(-16.9765908921007,-4.55,66.8108802047268));
#44452=CARTESIAN_POINT('Origin',(-23.5631918813915,-4.75,57.3105282424112));
#44453=CARTESIAN_POINT('',(-23.3729805781325,-4.55,57.3723316412862));
#44454=CARTESIAN_POINT('Origin',(-0.0610878597133323,-4.75,57.1064496864285));
#44455=CARTESIAN_POINT('',(-1.48277387709906,-4.55,57.158126120696));
#44456=CARTESIAN_POINT('',(-1.04315373364469,-4.95,56.8021287478558));
#44457=CARTESIAN_POINT('',(-10.4334709354135,-4.55,56.2173699512871));
#44458=CARTESIAN_POINT('',(-0.0819935523668635,-4.55,57.3053540655022));
#44459=CARTESIAN_POINT('',(-10.4334709354135,-4.55,56.2173699512871));
#44460=CARTESIAN_POINT('Origin',(-2.67496212708166,-4.75,70.4143940757733));
#44461=CARTESIAN_POINT('',(-2.87386650615531,-4.55,70.3934883831197));
#44462=CARTESIAN_POINT('Origin',(-11.2917687006698,-4.75,62.4701732534794));
#44463=CARTESIAN_POINT('',(-11.0928643215962,-4.55,62.4910789461329));
#44464=CARTESIAN_POINT('Origin',(-10.4334709354135,-4.95,56.2173699512871));
#44465=CARTESIAN_POINT('',(-10.4334709354135,-0.75,56.2173699512871));
#44466=CARTESIAN_POINT('',(-10.4334709354135,-4.95,56.2173699512871));
#44467=CARTESIAN_POINT('',(-11.8968694211607,-0.75,70.140676486443));
#44468=CARTESIAN_POINT('Origin',(-1.48277387709906,-4.95,57.158126120696));
#44469=CARTESIAN_POINT('',(-1.48277387709906,-0.75,57.158126120696));
#44470=CARTESIAN_POINT('',(-1.48277387709906,-4.95,57.158126120696));
#44471=CARTESIAN_POINT('',(-10.4334709354135,-0.75,56.2173699512871));
#44472=CARTESIAN_POINT('Origin',(4.53643638887053,-4.75,56.6360716017241));
#44473=CARTESIAN_POINT('',(10.4334709354135,-4.55,56.2173699512871));
#44474=CARTESIAN_POINT('',(10.7894683082537,-4.95,55.7777498078328));
#44475=CARTESIAN_POINT('',(1.48277387709899,-4.55,57.158126120696));
#44476=CARTESIAN_POINT('',(4.55734208152406,-4.55,56.8349759807978));
#44477=CARTESIAN_POINT('',(1.48277387709899,-4.55,57.158126120696));
#44478=CARTESIAN_POINT('Origin',(12.0234679435433,-4.75,69.4318265210573));
#44479=CARTESIAN_POINT('',(11.8245635644697,-4.55,69.4527322137109));
#44480=CARTESIAN_POINT('Origin',(1.943262884208,-4.75,63.4527408081954));
#44481=CARTESIAN_POINT('',(2.14216726328165,-4.55,63.4318351155418));
#44482=CARTESIAN_POINT('Origin',(9.40580052704283,-4.75,56.6669244866595));
#44483=CARTESIAN_POINT('',(21.8937230027002,-4.55,52.8196449541365));
#44484=CARTESIAN_POINT('',(22.1505388114683,-4.95,52.3156155498685));
#44485=CARTESIAN_POINT('',(13.3342143560438,-4.55,55.600797903511));
#44486=CARTESIAN_POINT('',(9.46760392591782,-4.55,56.8571357899185));
#44487=CARTESIAN_POINT('',(13.3342143560438,-4.55,55.600797903511));
#44488=CARTESIAN_POINT('Origin',(25.7263108420161,-4.75,63.9679238564773));
#44489=CARTESIAN_POINT('',(25.5360995387571,-4.55,64.0297272553523));
#44490=CARTESIAN_POINT('Origin',(14.6232606282171,-4.75,60.2152879895357));
#44491=CARTESIAN_POINT('',(14.8134719314761,-4.55,60.1534845906607));
#44492=CARTESIAN_POINT('Origin',(13.3342143560438,-4.95,55.600797903511));
#44493=CARTESIAN_POINT('',(13.3342143560438,-0.75,55.600797903511));
#44494=CARTESIAN_POINT('',(13.3342143560438,-4.95,55.600797903511));
#44495=CARTESIAN_POINT('',(17.6604522772931,-0.75,68.9155891316432));
#44496=CARTESIAN_POINT('Origin',(21.8937230027002,-4.95,52.8196449541365));
#44497=CARTESIAN_POINT('',(21.8937230027002,-0.75,52.8196449541365));
#44498=CARTESIAN_POINT('',(21.8937230027002,-4.95,52.8196449541365));
#44499=CARTESIAN_POINT('',(13.3342143560438,-0.75,55.600797903511));
#44500=CARTESIAN_POINT('Origin',(15.1931125922873,-4.75,56.8152429349561));
#44501=CARTESIAN_POINT('',(32.3971143170299,-4.55,47.113448015713));
#44502=CARTESIAN_POINT('',(32.5435244785437,-4.95,46.5670378541993));
#44503=CARTESIAN_POINT('',(24.60288568297,-4.55,51.613448015713));
#44504=CARTESIAN_POINT('',(15.2931125922873,-4.55,56.988448015713));
#44505=CARTESIAN_POINT('',(24.60288568297,-4.55,51.613448015713));
#44506=CARTESIAN_POINT('Origin',(36.9757639640145,-4.75,54.6439018343476));
#44507=CARTESIAN_POINT('',(36.8025588832576,-4.55,54.7439018343476));
#44508=CARTESIAN_POINT('Origin',(25.3351251684408,-4.75,53.2817240078565));
#44509=CARTESIAN_POINT('',(25.5083302491977,-4.55,53.1817240078565));
#44510=CARTESIAN_POINT('Origin',(22.2745611295625,-4.75,56.3758341156246));
#44511=CARTESIAN_POINT('',(41.4845962771032,-4.55,39.3481673235966));
#44512=CARTESIAN_POINT('',(41.5142019647506,-4.95,38.7832571508621));
#44513=CARTESIAN_POINT('',(34.7962928478066,-4.55,45.3703427808264));
#44514=CARTESIAN_POINT('',(22.4083872508343,-4.55,56.5244630807201));
#44515=CARTESIAN_POINT('',(34.7962928478066,-4.55,45.3703427808264));
#44516=CARTESIAN_POINT('Origin',(44.651050374428,-4.75,42.5659755617448));
#44517=CARTESIAN_POINT('',(44.5024214093325,-4.55,42.6998016830166));
#44518=CARTESIAN_POINT('Origin',(32.9815747704285,-4.75,43.6537894831763));
#44519=CARTESIAN_POINT('',(33.130203735524,-4.55,43.5199633619046));
#44520=CARTESIAN_POINT('Origin',(34.7962928478066,-4.95,45.3703427808264));
#44521=CARTESIAN_POINT('',(34.7962928478066,-0.75,45.3703427808264));
#44522=CARTESIAN_POINT('',(34.7962928478066,-4.95,45.3703427808264));
#44523=CARTESIAN_POINT('',(44.1641213368306,-0.75,55.7743703375099));
#44524=CARTESIAN_POINT('Origin',(41.4845962771032,-4.95,39.3481673235966));
#44525=CARTESIAN_POINT('',(41.4845962771032,-0.75,39.3481673235966));
#44526=CARTESIAN_POINT('',(41.4845962771032,-4.95,39.3481673235966));
#44527=CARTESIAN_POINT('',(34.7962928478066,-0.75,45.3703427808264));
#44528=CARTESIAN_POINT('Origin',(36.9378826890766,-4.75,32.6464621623362));
#44529=CARTESIAN_POINT('',(43.4689350440559,-4.55,37.1443358553582));
#44530=CARTESIAN_POINT('',(36.416687466477,-9.59885182881449,38.2613021409633));
#44531=CARTESIAN_POINT('',(37.0554397395351,-4.55,32.4846587634612));
#44532=CARTESIAN_POINT('Origin',(30.6311930629899,-4.75,54.4737114944304));
#44533=CARTESIAN_POINT('',(48.7590023146881,-4.55,29.8631829059837));
#44534=CARTESIAN_POINT('',(30.7929964618649,-4.55,54.5912685448889));
#44535=CARTESIAN_POINT('',(48.6705096178552,-4.95,29.3044620073168));
#44536=CARTESIAN_POINT('Origin',(48.1261830212504,-4.75,29.156199181259));
#44537=CARTESIAN_POINT('',(48.0086259707919,-4.55,29.318002580134));
#44538=CARTESIAN_POINT('Origin',(39.7995049951658,-4.75,50.2569496582896));
#44539=CARTESIAN_POINT('',(53.9024059794693,-4.55,19.0730340959289));
#44540=CARTESIAN_POINT('',(53.6996824536426,-4.95,18.5449212556416));
#44541=CARTESIAN_POINT('',(50.2417761917871,-4.55,27.2949432147124));
#44542=CARTESIAN_POINT('',(39.9822140866944,-4.55,50.3382969869048));
#44543=CARTESIAN_POINT('',(50.2417761917871,-4.55,27.2949432147124));
#44544=CARTESIAN_POINT('Origin',(47.347560414623,-4.75,15.9357015669907));
#44545=CARTESIAN_POINT('',(47.2662130860078,-4.55,16.1184106585192));
#44546=CARTESIAN_POINT('Origin',(37.1294177662123,-4.75,21.6758723673006));
#44547=CARTESIAN_POINT('',(37.2107650948274,-4.55,21.493163275772));
#44548=CARTESIAN_POINT('Origin',(48.9086937721936,-4.75,43.0955974455432));
#44549=CARTESIAN_POINT('',(56.6900158505068,-4.55,7.44930217331019));
#44550=CARTESIAN_POINT('',(56.3819214865404,-4.95,6.97487845668957));
#44551=CARTESIAN_POINT('',(54.818810633147,-4.55,16.2526305799144));
#44552=CARTESIAN_POINT('',(49.1043232923404,-4.55,43.1371797837068));
#44553=CARTESIAN_POINT('',(54.818810633147,-4.55,16.2526305799144));
#44554=CARTESIAN_POINT('Origin',(42.8193160267201,-4.75,4.29652579183608));
#44555=CARTESIAN_POINT('',(42.7777336885565,-4.55,4.49215531198284));
#44556=CARTESIAN_POINT('Origin',(34.0179129278965,-4.75,12.0357314030095));
#44557=CARTESIAN_POINT('',(34.0594952660601,-4.55,11.8401018828628));
#44558=CARTESIAN_POINT('Origin',(54.818810633147,-4.95,16.2526305799144));
#44559=CARTESIAN_POINT('',(54.818810633147,-0.75,16.2526305799144));
#44560=CARTESIAN_POINT('',(54.818810633147,-4.95,16.2526305799144));
#44561=CARTESIAN_POINT('',(68.5128770434203,-0.75,19.1633942513631));
#44562=CARTESIAN_POINT('Origin',(56.6900158505068,-4.95,7.44930217331019));
#44563=CARTESIAN_POINT('',(56.6900158505068,-0.75,7.44930217331019));
#44564=CARTESIAN_POINT('',(56.6900158505068,-4.95,7.44930217331019));
#44565=CARTESIAN_POINT('',(54.818810633147,-0.75,16.2526305799144));
#44566=CARTESIAN_POINT('Origin',(-12.2,4.75,3.73));
#44567=CARTESIAN_POINT('',(-12.,4.55,2.55));
#44568=CARTESIAN_POINT('',(-12.4,4.95,2.95));
#44569=CARTESIAN_POINT('',(-12.,4.55,-2.55));
#44570=CARTESIAN_POINT('',(-12.,4.55,3.73));
#44571=CARTESIAN_POINT('',(-12.,4.55,-2.55));
#44572=CARTESIAN_POINT('Origin',(-6.,4.75,2.75));
#44573=CARTESIAN_POINT('',(-9.67975206294045,4.55,2.55));
#44574=CARTESIAN_POINT('Origin',(0.,1.99999999999999,0.));
#44575=CARTESIAN_POINT('',(-6.,4.55,2.55));
#44576=CARTESIAN_POINT('Origin',(6.,4.75,-2.75));
#44577=CARTESIAN_POINT('',(-9.67975206294045,4.55,-2.55));
#44578=CARTESIAN_POINT('',(6.,4.55,-2.55));
#44579=CARTESIAN_POINT('Origin',(0.,1.99999999999999,0.));
#44580=CARTESIAN_POINT('Origin',(12.,-4.95,-2.55));
#44581=CARTESIAN_POINT('',(-12.,-4.55,-2.55));
#44582=CARTESIAN_POINT('',(-12.,-4.95,-2.55));
#44583=CARTESIAN_POINT('',(-9.67975206294045,-4.55,-2.55));
#44584=CARTESIAN_POINT('',(6.,-4.55,-2.55));
#44585=CARTESIAN_POINT('',(-9.67975206294045,0.,-2.55));
#44586=CARTESIAN_POINT('Origin',(-12.,-4.95,-2.55));
#44587=CARTESIAN_POINT('',(-12.,-4.55,2.55));
#44588=CARTESIAN_POINT('',(-12.,-4.95,2.55));
#44589=CARTESIAN_POINT('',(-12.,-4.55,33.725));
#44590=CARTESIAN_POINT('Origin',(-12.,-4.95,2.55));
#44591=CARTESIAN_POINT('',(-9.67975206294045,-4.55,2.55));
#44592=CARTESIAN_POINT('',(-9.67975206294045,0.,2.55));
#44593=CARTESIAN_POINT('',(-6.,-4.55,2.55));
#44594=CARTESIAN_POINT('Origin',(0.,0.,0.));
#44595=CARTESIAN_POINT('',(9.67975206294045,4.55,2.55));
#44596=CARTESIAN_POINT('Origin',(0.,1.99999999999999,0.));
#44597=CARTESIAN_POINT('',(9.67975206294045,-4.55,2.55));
#44598=CARTESIAN_POINT('',(9.67975206294045,0.,2.55));
#44599=CARTESIAN_POINT('Origin',(0.,-1.99999999999999,0.));
#44600=CARTESIAN_POINT('Origin',(0.,-1.99999999999999,0.));
#44601=CARTESIAN_POINT('Origin',(-12.2,-4.75,33.725));
#44602=CARTESIAN_POINT('',(-12.,-4.55,2.55));
#44603=CARTESIAN_POINT('',(-12.4,-4.95,-2.95));
#44604=CARTESIAN_POINT('Origin',(-6.,-4.75,2.75));
#44605=CARTESIAN_POINT('Origin',(6.,-4.75,-2.75));
#44606=CARTESIAN_POINT('Origin',(0.,-1.99999999999999,0.));
#44607=CARTESIAN_POINT('Origin',(6.,-4.75,-2.75));
#44608=CARTESIAN_POINT('',(12.,-4.55,-2.55));
#44609=CARTESIAN_POINT('',(9.67975206294045,-4.55,-2.55));
#44610=CARTESIAN_POINT('',(6.,-4.55,-2.55));
#44611=CARTESIAN_POINT('Origin',(0.,-1.99999999999999,0.));
#44612=CARTESIAN_POINT('',(12.4,-4.95,-2.95));
#44613=CARTESIAN_POINT('Origin',(12.2,-4.75,36.275));
#44614=CARTESIAN_POINT('',(12.,-4.55,2.55));
#44615=CARTESIAN_POINT('',(12.4,-4.95,2.95));
#44616=CARTESIAN_POINT('',(12.,-4.55,36.275));
#44617=CARTESIAN_POINT('Origin',(-6.,-4.75,2.75));
#44618=CARTESIAN_POINT('',(-6.,-4.55,2.55));
#44619=CARTESIAN_POINT('Origin',(12.,-4.95,-2.55));
#44620=CARTESIAN_POINT('',(12.,4.55,-2.55));
#44621=CARTESIAN_POINT('',(12.,-4.95,-2.55));
#44622=CARTESIAN_POINT('',(9.67975206294045,4.55,-2.55));
#44623=CARTESIAN_POINT('',(6.,4.55,-2.55));
#44624=CARTESIAN_POINT('',(9.67975206294045,0.,-2.55));
#44625=CARTESIAN_POINT('Origin',(12.,-4.95,2.55));
#44626=CARTESIAN_POINT('',(12.,4.55,2.55));
#44627=CARTESIAN_POINT('',(12.,-4.95,2.55));
#44628=CARTESIAN_POINT('',(12.,4.55,6.28));
#44629=CARTESIAN_POINT('Origin',(-12.,-4.95,2.55));
#44630=CARTESIAN_POINT('',(-6.,4.55,2.55));
#44631=CARTESIAN_POINT('Origin',(6.,4.75,-2.75));
#44632=CARTESIAN_POINT('Origin',(0.,1.99999999999999,0.));
#44633=CARTESIAN_POINT('',(12.,4.55,-2.55));
#44634=CARTESIAN_POINT('Origin',(12.2,4.75,6.28));
#44635=CARTESIAN_POINT('',(12.,4.55,2.55));
#44636=CARTESIAN_POINT('Origin',(-6.,4.75,2.75));
#44637=CARTESIAN_POINT('Origin',(62.6014464469636,0.75,13.3063482123366));
#44638=CARTESIAN_POINT('Origin',(70.3840822607801,-4.95,10.3600658447588));
#44639=CARTESIAN_POINT('',(56.6900158505068,-0.75,7.44930217331019));
#44640=CARTESIAN_POINT('Origin',(62.6014464469636,-0.75,13.3063482123366));
#44641=CARTESIAN_POINT('Origin',(58.4669092891264,0.75,26.0311451568513));
#44642=CARTESIAN_POINT('Origin',(53.9024059794693,-4.95,19.0730340959289));
#44643=CARTESIAN_POINT('',(53.9024059794693,-0.75,19.0730340959289));
#44644=CARTESIAN_POINT('',(53.9024059794693,-4.95,19.0730340959289));
#44645=CARTESIAN_POINT('',(50.2417761917871,-0.75,27.2949432147124));
#44646=CARTESIAN_POINT('',(50.2417761917871,-0.75,27.2949432147124));
#44647=CARTESIAN_POINT('',(50.2417761917871,-4.95,27.2949432147124));
#44648=CARTESIAN_POINT('Origin',(66.6920423864657,-4.95,24.7673470989902));
#44649=CARTESIAN_POINT('',(53.9024059794693,-0.75,19.0730340959289));
#44650=CARTESIAN_POINT('Origin',(50.2417761917871,-4.95,27.2949432147124));
#44651=CARTESIAN_POINT('',(63.0314125987835,-0.75,32.9892562177736));
#44652=CARTESIAN_POINT('Origin',(58.4669092891264,-0.75,26.0311451568513));
#44653=CARTESIAN_POINT('Origin',(51.7770876399966,0.75,37.6182561467183));
#44654=CARTESIAN_POINT('Origin',(48.7590023146881,-4.95,29.8631829059837));
#44655=CARTESIAN_POINT('',(48.7590023146881,-0.75,29.8631829059837));
#44656=CARTESIAN_POINT('',(48.7590023146881,-4.95,29.8631829059837));
#44657=CARTESIAN_POINT('',(43.4689350440559,-0.75,37.1443358553582));
#44658=CARTESIAN_POINT('',(43.4689350440559,-0.75,37.1443358553582));
#44659=CARTESIAN_POINT('',(43.4689350440559,-4.95,37.1443358553582));
#44660=CARTESIAN_POINT('Origin',(60.0852402359374,-4.95,38.0921764380783));
#44661=CARTESIAN_POINT('',(48.7590023146881,-0.75,29.8631829059837));
#44662=CARTESIAN_POINT('Origin',(43.4689350440559,-4.95,37.1443358553582));
#44663=CARTESIAN_POINT('',(54.7951729653051,-0.75,45.3733293874529));
#44664=CARTESIAN_POINT('Origin',(51.7770876399966,-0.75,37.6182561467183));
#44665=CARTESIAN_POINT('Origin',(42.8243588069669,0.75,47.5612688305533));
#44666=CARTESIAN_POINT('Origin',(50.8524247661272,-4.95,49.7521948802802));
#44667=CARTESIAN_POINT('',(41.4845962771032,-0.75,39.3481673235966));
#44668=CARTESIAN_POINT('Origin',(42.8243588069669,-0.75,47.5612688305533));
#44669=CARTESIAN_POINT('Origin',(32.,0.75,55.4256258422041));
#44670=CARTESIAN_POINT('Origin',(32.3971143170299,-4.95,47.113448015713));
#44671=CARTESIAN_POINT('',(32.3971143170299,-0.75,47.113448015713));
#44672=CARTESIAN_POINT('',(32.3971143170299,-4.95,47.113448015713));
#44673=CARTESIAN_POINT('',(24.60288568297,-0.75,51.613448015713));
#44674=CARTESIAN_POINT('',(24.60288568297,-0.75,51.613448015713));
#44675=CARTESIAN_POINT('',(24.60288568297,-4.95,51.613448015713));
#44676=CARTESIAN_POINT('Origin',(39.3971143170299,-4.95,59.2378036686952));
#44677=CARTESIAN_POINT('',(32.3971143170299,-0.75,47.113448015713));
#44678=CARTESIAN_POINT('Origin',(24.60288568297,-4.95,51.613448015713));
#44679=CARTESIAN_POINT('',(31.60288568297,-0.75,63.7378036686952));
#44680=CARTESIAN_POINT('Origin',(32.,-0.75,55.4256258422041));
#44681=CARTESIAN_POINT('Origin',(19.7770876399966,0.75,60.8676170428898));
#44682=CARTESIAN_POINT('Origin',(26.2199609239494,-4.95,66.1344361822686));
#44683=CARTESIAN_POINT('',(21.8937230027002,-0.75,52.8196449541365));
#44684=CARTESIAN_POINT('Origin',(19.7770876399966,-0.75,60.8676170428898));
#44685=CARTESIAN_POINT('Origin',(6.68982164912979,0.75,63.6494013035695));
#44686=CARTESIAN_POINT('Origin',(10.4334709354135,-4.95,56.2173699512871));
#44687=CARTESIAN_POINT('',(10.4334709354135,-0.75,56.2173699512871));
#44688=CARTESIAN_POINT('',(10.4334709354135,-4.95,56.2173699512871));
#44689=CARTESIAN_POINT('',(1.48277387709899,-0.75,57.158126120696));
#44690=CARTESIAN_POINT('',(1.48277387709899,-0.75,57.158126120696));
#44691=CARTESIAN_POINT('',(1.48277387709899,-4.95,57.158126120696));
#44692=CARTESIAN_POINT('Origin',(11.8968694211606,-4.95,70.140676486443));
#44693=CARTESIAN_POINT('',(10.4334709354135,-0.75,56.2173699512871));
#44694=CARTESIAN_POINT('Origin',(1.48277387709899,-4.95,57.158126120696));
#44695=CARTESIAN_POINT('',(2.94617236284613,-0.75,71.0814326558519));
#44696=CARTESIAN_POINT('Origin',(6.68982164912979,-0.75,63.6494013035695));
#44697=CARTESIAN_POINT('Origin',(-6.68982164912987,0.75,63.6494013035695));
#44698=CARTESIAN_POINT('Origin',(-2.94617236284622,-4.95,71.0814326558519));
#44699=CARTESIAN_POINT('',(-1.48277387709906,-0.75,57.158126120696));
#44700=CARTESIAN_POINT('Origin',(-6.68982164912987,-0.75,63.6494013035695));
#44701=CARTESIAN_POINT('Origin',(-19.7770876399966,0.75,60.8676170428898));
#44702=CARTESIAN_POINT('Origin',(-13.3342143560438,-4.95,55.600797903511));
#44703=CARTESIAN_POINT('',(-13.3342143560438,-0.75,55.600797903511));
#44704=CARTESIAN_POINT('',(-13.3342143560438,-4.95,55.600797903511));
#44705=CARTESIAN_POINT('',(-21.8937230027002,-0.75,52.8196449541365));
#44706=CARTESIAN_POINT('',(-21.8937230027002,-0.75,52.8196449541365));
#44707=CARTESIAN_POINT('',(-21.8937230027002,-4.95,52.8196449541365));
#44708=CARTESIAN_POINT('Origin',(-17.6604522772931,-4.95,68.9155891316432));
#44709=CARTESIAN_POINT('',(-13.3342143560438,-0.75,55.600797903511));
#44710=CARTESIAN_POINT('Origin',(-21.8937230027002,-4.95,52.8196449541365));
#44711=CARTESIAN_POINT('',(-26.2199609239495,-0.75,66.1344361822686));
#44712=CARTESIAN_POINT('Origin',(-19.7770876399966,-0.75,60.8676170428898));
#44713=CARTESIAN_POINT('Origin',(-32.,0.75,55.4256258422041));
#44714=CARTESIAN_POINT('Origin',(-24.6028856829701,-4.95,51.613448015713));
#44715=CARTESIAN_POINT('',(-24.6028856829701,-0.75,51.613448015713));
#44716=CARTESIAN_POINT('',(-24.6028856829701,-4.95,51.613448015713));
#44717=CARTESIAN_POINT('',(-32.39711431703,-0.75,47.113448015713));
#44718=CARTESIAN_POINT('',(-32.39711431703,-0.75,47.113448015713));
#44719=CARTESIAN_POINT('',(-32.39711431703,-4.95,47.113448015713));
#44720=CARTESIAN_POINT('Origin',(-31.6028856829701,-4.95,63.7378036686951));
#44721=CARTESIAN_POINT('',(-24.6028856829701,-0.75,51.613448015713));
#44722=CARTESIAN_POINT('Origin',(-32.39711431703,-4.95,47.113448015713));
#44723=CARTESIAN_POINT('',(-39.39711431703,-0.75,59.2378036686951));
#44724=CARTESIAN_POINT('Origin',(-32.,-0.75,55.4256258422041));
#44725=CARTESIAN_POINT('Origin',(-42.8243588069669,0.75,47.5612688305532));
#44726=CARTESIAN_POINT('Origin',(-44.1641213368307,-4.95,55.7743703375098));
#44727=CARTESIAN_POINT('',(-34.7962928478067,-0.75,45.3703427808263));
#44728=CARTESIAN_POINT('Origin',(-42.8243588069669,-0.75,47.5612688305532));
#44729=CARTESIAN_POINT('Origin',(-51.7770876399966,0.75,37.6182561467183));
#44730=CARTESIAN_POINT('Origin',(-43.4689350440559,-4.95,37.1443358553582));
#44731=CARTESIAN_POINT('',(-43.4689350440559,-0.75,37.1443358553582));
#44732=CARTESIAN_POINT('',(-43.4689350440559,-4.95,37.1443358553582));
#44733=CARTESIAN_POINT('',(-48.7590023146881,-0.75,29.8631829059837));
#44734=CARTESIAN_POINT('',(-48.7590023146881,-0.75,29.8631829059837));
#44735=CARTESIAN_POINT('',(-48.7590023146881,-4.95,29.8631829059837));
#44736=CARTESIAN_POINT('Origin',(-54.7951729653051,-4.95,45.3733293874529));
#44737=CARTESIAN_POINT('',(-43.4689350440559,-0.75,37.1443358553582));
#44738=CARTESIAN_POINT('Origin',(-48.7590023146881,-4.95,29.8631829059837));
#44739=CARTESIAN_POINT('',(-60.0852402359374,-0.75,38.0921764380783));
#44740=CARTESIAN_POINT('Origin',(-51.7770876399966,-0.75,37.6182561467183));
#44741=CARTESIAN_POINT('Origin',(-58.4669092891265,0.75,26.0311451568512));
#44742=CARTESIAN_POINT('Origin',(-63.0314125987836,-4.95,32.9892562177735));
#44743=CARTESIAN_POINT('',(-50.2417761917872,-0.75,27.2949432147123));
#44744=CARTESIAN_POINT('Origin',(-58.4669092891265,-0.75,26.0311451568512));
#44745=CARTESIAN_POINT('Origin',(-62.6014464469636,0.75,13.3063482123366));
#44746=CARTESIAN_POINT('Origin',(-54.818810633147,-4.95,16.2526305799144));
#44747=CARTESIAN_POINT('',(-54.818810633147,-0.75,16.2526305799144));
#44748=CARTESIAN_POINT('',(-54.818810633147,-4.95,16.2526305799144));
#44749=CARTESIAN_POINT('',(-56.6900158505068,-0.75,7.44930217331014));
#44750=CARTESIAN_POINT('',(-56.6900158505068,-0.75,7.44930217331014));
#44751=CARTESIAN_POINT('',(-56.6900158505068,-4.95,7.44930217331014));
#44752=CARTESIAN_POINT('Origin',(-68.5128770434203,-4.95,19.163394251363));
#44753=CARTESIAN_POINT('',(-54.818810633147,-0.75,16.2526305799144));
#44754=CARTESIAN_POINT('Origin',(-56.6900158505068,-4.95,7.44930217331014));
#44755=CARTESIAN_POINT('',(-70.3840822607801,-0.75,10.3600658447588));
#44756=CARTESIAN_POINT('Origin',(-62.6014464469636,-0.75,13.3063482123366));
#44757=CARTESIAN_POINT('Origin',(-64.,0.75,-7.83773951454306E-15));
#44758=CARTESIAN_POINT('Origin',(-71.,-4.95,4.49999999999999));
#44759=CARTESIAN_POINT('',(-57.,-0.75,4.49999999999999));
#44760=CARTESIAN_POINT('Origin',(-64.,-0.75,-7.83773951454306E-15));
#44761=CARTESIAN_POINT('Origin',(-62.6014464469636,0.75,-13.3063482123366));
#44762=CARTESIAN_POINT('Origin',(-56.6900158505068,-4.95,-7.44930217331018));
#44763=CARTESIAN_POINT('',(-56.6900158505068,-0.75,-7.44930217331018));
#44764=CARTESIAN_POINT('',(-56.6900158505068,-4.95,-7.44930217331018));
#44765=CARTESIAN_POINT('',(-54.818810633147,-0.75,-16.2526305799144));
#44766=CARTESIAN_POINT('',(-54.818810633147,-0.75,-16.2526305799144));
#44767=CARTESIAN_POINT('',(-54.818810633147,-4.95,-16.2526305799144));
#44768=CARTESIAN_POINT('Origin',(-70.3840822607801,-4.95,-10.3600658447588));
#44769=CARTESIAN_POINT('',(-56.6900158505068,-0.75,-7.44930217331018));
#44770=CARTESIAN_POINT('Origin',(-54.818810633147,-4.95,-16.2526305799144));
#44771=CARTESIAN_POINT('',(-68.5128770434203,-0.75,-19.1633942513631));
#44772=CARTESIAN_POINT('Origin',(-62.6014464469636,-0.75,-13.3063482123366));
#44773=CARTESIAN_POINT('Origin',(-58.4669092891264,0.75,-26.0311451568512));
#44774=CARTESIAN_POINT('Origin',(-66.6920423864657,-4.95,-24.7673470989901));
#44775=CARTESIAN_POINT('',(-53.9024059794693,-0.75,-19.0730340959289));
#44776=CARTESIAN_POINT('Origin',(-58.4669092891264,-0.75,-26.0311451568512));
#44777=CARTESIAN_POINT('Origin',(-51.7770876399966,0.75,-37.6182561467183));
#44778=CARTESIAN_POINT('Origin',(-48.7590023146881,-4.95,-29.8631829059837));
#44779=CARTESIAN_POINT('',(-48.7590023146881,-0.75,-29.8631829059837));
#44780=CARTESIAN_POINT('',(-48.7590023146881,-4.95,-29.8631829059837));
#44781=CARTESIAN_POINT('',(-43.4689350440559,-0.75,-37.1443358553582));
#44782=CARTESIAN_POINT('',(-43.4689350440559,-0.75,-37.1443358553582));
#44783=CARTESIAN_POINT('',(-43.4689350440559,-4.95,-37.1443358553582));
#44784=CARTESIAN_POINT('Origin',(-60.0852402359374,-4.95,-38.0921764380783));
#44785=CARTESIAN_POINT('',(-48.7590023146881,-0.75,-29.8631829059837));
#44786=CARTESIAN_POINT('Origin',(-43.4689350440559,-4.95,-37.1443358553582));
#44787=CARTESIAN_POINT('',(-54.7951729653051,-0.75,-45.3733293874529));
#44788=CARTESIAN_POINT('Origin',(-51.7770876399966,-0.75,-37.6182561467183));
#44789=CARTESIAN_POINT('Origin',(-42.8243588069669,0.75,-47.5612688305532));
#44790=CARTESIAN_POINT('Origin',(-50.8524247661272,-4.95,-49.7521948802801));
#44791=CARTESIAN_POINT('',(-41.4845962771032,-0.75,-39.3481673235966));
#44792=CARTESIAN_POINT('Origin',(-42.8243588069669,-0.75,-47.5612688305532));
#44793=CARTESIAN_POINT('Origin',(-32.39711431703,4.95,-47.113448015713));
#44794=CARTESIAN_POINT('',(-32.39711431703,0.75,-47.113448015713));
#44795=CARTESIAN_POINT('Origin',(-32.,0.75,-55.4256258422041));
#44796=CARTESIAN_POINT('Origin',(-32.39711431703,-4.95,-47.113448015713));
#44797=CARTESIAN_POINT('',(-32.39711431703,-0.75,-47.113448015713));
#44798=CARTESIAN_POINT('',(-32.39711431703,-4.95,-47.113448015713));
#44799=CARTESIAN_POINT('',(-24.60288568297,-0.75,-51.613448015713));
#44800=CARTESIAN_POINT('',(-24.60288568297,-0.75,-51.613448015713));
#44801=CARTESIAN_POINT('',(-24.60288568297,-4.95,-51.613448015713));
#44802=CARTESIAN_POINT('Origin',(-39.39711431703,-4.95,-59.2378036686952));
#44803=CARTESIAN_POINT('',(-32.39711431703,-0.75,-47.113448015713));
#44804=CARTESIAN_POINT('Origin',(-24.60288568297,-4.95,-51.613448015713));
#44805=CARTESIAN_POINT('',(-31.60288568297,-0.75,-63.7378036686952));
#44806=CARTESIAN_POINT('Origin',(-32.,-0.75,-55.4256258422041));
#44807=CARTESIAN_POINT('Origin',(-19.7770876399966,0.75,-60.8676170428898));
#44808=CARTESIAN_POINT('Origin',(-26.2199609239495,-4.95,-66.1344361822686));
#44809=CARTESIAN_POINT('',(-21.8937230027002,-0.75,-52.8196449541365));
#44810=CARTESIAN_POINT('Origin',(-19.7770876399966,-0.75,-60.8676170428898));
#44811=CARTESIAN_POINT('Origin',(-6.68982164912981,0.75,-63.6494013035695));
#44812=CARTESIAN_POINT('Origin',(-10.4334709354135,-4.95,-56.2173699512871));
#44813=CARTESIAN_POINT('',(-10.4334709354135,-0.75,-56.2173699512871));
#44814=CARTESIAN_POINT('',(-10.4334709354135,-4.95,-56.2173699512871));
#44815=CARTESIAN_POINT('',(-1.48277387709901,-0.75,-57.158126120696));
#44816=CARTESIAN_POINT('',(-1.48277387709901,-0.75,-57.158126120696));
#44817=CARTESIAN_POINT('',(-1.48277387709901,-4.95,-57.158126120696));
#44818=CARTESIAN_POINT('Origin',(-11.8968694211606,-4.95,-70.140676486443));
#44819=CARTESIAN_POINT('',(-10.4334709354135,-0.75,-56.2173699512871));
#44820=CARTESIAN_POINT('Origin',(-1.48277387709901,-4.95,-57.158126120696));
#44821=CARTESIAN_POINT('',(-2.94617236284616,-0.75,-71.0814326558519));
#44822=CARTESIAN_POINT('Origin',(-6.68982164912981,-0.75,-63.6494013035695));
#44823=CARTESIAN_POINT('Origin',(6.68982164912984,0.75,-63.6494013035695));
#44824=CARTESIAN_POINT('Origin',(1.48277387709903,-4.95,-57.158126120696));
#44825=CARTESIAN_POINT('',(1.48277387709903,-0.75,-57.158126120696));
#44826=CARTESIAN_POINT('',(1.48277387709903,-4.95,-57.158126120696));
#44827=CARTESIAN_POINT('',(10.4334709354135,-0.75,-56.2173699512871));
#44828=CARTESIAN_POINT('',(10.4334709354135,-0.75,-56.2173699512871));
#44829=CARTESIAN_POINT('',(10.4334709354135,-4.95,-56.2173699512871));
#44830=CARTESIAN_POINT('Origin',(2.94617236284618,-4.95,-71.0814326558518));
#44831=CARTESIAN_POINT('',(1.48277387709903,-0.75,-57.158126120696));
#44832=CARTESIAN_POINT('Origin',(10.4334709354135,-4.95,-56.2173699512871));
#44833=CARTESIAN_POINT('',(11.8968694211606,-0.75,-70.140676486443));
#44834=CARTESIAN_POINT('Origin',(6.68982164912984,-0.75,-63.6494013035695));
#44835=CARTESIAN_POINT('Origin',(19.7770876399966,0.75,-60.8676170428898));
#44836=CARTESIAN_POINT('',(26.2199609239495,0.75,-66.1344361822686));
#44837=CARTESIAN_POINT('Origin',(26.2199609239495,4.95,-66.1344361822686));
#44838=CARTESIAN_POINT('Origin',(17.6604522772931,-4.95,-68.9155891316432));
#44839=CARTESIAN_POINT('',(13.3342143560438,-0.75,-55.600797903511));
#44840=CARTESIAN_POINT('Origin',(19.7770876399966,-0.75,-60.8676170428898));
#44841=CARTESIAN_POINT('Origin',(24.60288568297,4.95,-51.613448015713));
#44842=CARTESIAN_POINT('',(24.60288568297,0.75,-51.613448015713));
#44843=CARTESIAN_POINT('',(24.60288568297,4.95,-51.613448015713));
#44844=CARTESIAN_POINT('',(24.60288568297,0.75,-51.613448015713));
#44845=CARTESIAN_POINT('Origin',(32.,0.75,-55.4256258422041));
#44846=CARTESIAN_POINT('',(32.39711431703,0.75,-47.113448015713));
#44847=CARTESIAN_POINT('',(32.39711431703,0.75,-47.113448015713));
#44848=CARTESIAN_POINT('',(39.39711431703,0.75,-59.2378036686951));
#44849=CARTESIAN_POINT('Origin',(32.39711431703,4.95,-47.113448015713));
#44850=CARTESIAN_POINT('',(32.39711431703,4.95,-47.113448015713));
#44851=CARTESIAN_POINT('Origin',(39.39711431703,4.95,-59.2378036686951));
#44852=CARTESIAN_POINT('Origin',(24.60288568297,-4.95,-51.613448015713));
#44853=CARTESIAN_POINT('',(24.60288568297,-0.75,-51.613448015713));
#44854=CARTESIAN_POINT('',(24.60288568297,-4.95,-51.613448015713));
#44855=CARTESIAN_POINT('',(32.39711431703,-0.75,-47.113448015713));
#44856=CARTESIAN_POINT('',(32.39711431703,-0.75,-47.113448015713));
#44857=CARTESIAN_POINT('',(32.39711431703,-4.95,-47.113448015713));
#44858=CARTESIAN_POINT('Origin',(31.60288568297,-4.95,-63.7378036686951));
#44859=CARTESIAN_POINT('',(24.60288568297,-0.75,-51.613448015713));
#44860=CARTESIAN_POINT('Origin',(32.39711431703,-4.95,-47.113448015713));
#44861=CARTESIAN_POINT('',(39.39711431703,-0.75,-59.2378036686951));
#44862=CARTESIAN_POINT('Origin',(32.,-0.75,-55.4256258422041));
#44863=CARTESIAN_POINT('Origin',(34.7962928478066,4.95,-45.3703427808263));
#44864=CARTESIAN_POINT('',(34.7962928478066,0.75,-45.3703427808263));
#44865=CARTESIAN_POINT('',(34.7962928478066,4.95,-45.3703427808263));
#44866=CARTESIAN_POINT('',(34.7962928478066,0.75,-45.3703427808263));
#44867=CARTESIAN_POINT('Origin',(42.8243588069669,0.75,-47.5612688305532));
#44868=CARTESIAN_POINT('',(41.4845962771032,0.75,-39.3481673235966));
#44869=CARTESIAN_POINT('',(41.4845962771032,0.75,-39.3481673235966));
#44870=CARTESIAN_POINT('',(50.8524247661272,0.75,-49.7521948802801));
#44871=CARTESIAN_POINT('Origin',(41.4845962771032,4.95,-39.3481673235966));
#44872=CARTESIAN_POINT('',(41.4845962771032,4.95,-39.3481673235966));
#44873=CARTESIAN_POINT('Origin',(50.8524247661272,4.95,-49.7521948802801));
#44874=CARTESIAN_POINT('Origin',(44.1641213368307,-4.95,-55.7743703375099));
#44875=CARTESIAN_POINT('',(34.7962928478066,-0.75,-45.3703427808263));
#44876=CARTESIAN_POINT('Origin',(42.8243588069669,-0.75,-47.5612688305532));
#44877=CARTESIAN_POINT('Origin',(43.4689350440559,4.95,-37.1443358553582));
#44878=CARTESIAN_POINT('',(43.4689350440559,0.75,-37.1443358553582));
#44879=CARTESIAN_POINT('',(43.4689350440559,4.95,-37.1443358553582));
#44880=CARTESIAN_POINT('',(43.4689350440559,0.75,-37.1443358553582));
#44881=CARTESIAN_POINT('Origin',(51.7770876399966,0.75,-37.6182561467183));
#44882=CARTESIAN_POINT('',(48.7590023146881,0.75,-29.8631829059837));
#44883=CARTESIAN_POINT('',(48.7590023146881,0.75,-29.8631829059837));
#44884=CARTESIAN_POINT('',(60.0852402359374,0.75,-38.0921764380783));
#44885=CARTESIAN_POINT('Origin',(48.7590023146881,4.95,-29.8631829059837));
#44886=CARTESIAN_POINT('',(48.7590023146881,4.95,-29.8631829059837));
#44887=CARTESIAN_POINT('Origin',(60.0852402359374,4.95,-38.0921764380783));
#44888=CARTESIAN_POINT('Origin',(43.4689350440559,-4.95,-37.1443358553582));
#44889=CARTESIAN_POINT('',(43.4689350440559,-0.75,-37.1443358553582));
#44890=CARTESIAN_POINT('',(43.4689350440559,-4.95,-37.1443358553582));
#44891=CARTESIAN_POINT('',(48.7590023146881,-0.75,-29.8631829059837));
#44892=CARTESIAN_POINT('',(48.7590023146881,-0.75,-29.8631829059837));
#44893=CARTESIAN_POINT('',(48.7590023146881,-4.95,-29.8631829059837));
#44894=CARTESIAN_POINT('Origin',(54.7951729653051,-4.95,-45.3733293874529));
#44895=CARTESIAN_POINT('',(43.4689350440559,-0.75,-37.1443358553582));
#44896=CARTESIAN_POINT('Origin',(48.7590023146881,-4.95,-29.8631829059837));
#44897=CARTESIAN_POINT('',(60.0852402359374,-0.75,-38.0921764380783));
#44898=CARTESIAN_POINT('Origin',(51.7770876399966,-0.75,-37.6182561467183));
#44899=CARTESIAN_POINT('Origin',(50.2417761917872,4.95,-27.2949432147123));
#44900=CARTESIAN_POINT('',(50.2417761917872,0.75,-27.2949432147123));
#44901=CARTESIAN_POINT('',(50.2417761917872,4.95,-27.2949432147123));
#44902=CARTESIAN_POINT('',(50.2417761917872,0.75,-27.2949432147123));
#44903=CARTESIAN_POINT('Origin',(58.4669092891265,0.75,-26.0311451568512));
#44904=CARTESIAN_POINT('',(53.9024059794694,0.75,-19.0730340959289));
#44905=CARTESIAN_POINT('',(53.9024059794694,0.75,-19.0730340959289));
#44906=CARTESIAN_POINT('',(66.6920423864658,0.75,-24.7673470989901));
#44907=CARTESIAN_POINT('Origin',(53.9024059794694,4.95,-19.0730340959289));
#44908=CARTESIAN_POINT('',(53.9024059794694,4.95,-19.0730340959289));
#44909=CARTESIAN_POINT('Origin',(66.6920423864658,4.95,-24.7673470989901));
#44910=CARTESIAN_POINT('Origin',(63.0314125987836,-4.95,-32.9892562177735));
#44911=CARTESIAN_POINT('',(50.2417761917872,-0.75,-27.2949432147123));
#44912=CARTESIAN_POINT('Origin',(58.4669092891265,-0.75,-26.0311451568512));
#44913=CARTESIAN_POINT('Origin',(54.818810633147,4.95,-16.2526305799144));
#44914=CARTESIAN_POINT('',(54.818810633147,0.75,-16.2526305799144));
#44915=CARTESIAN_POINT('',(54.818810633147,4.95,-16.2526305799144));
#44916=CARTESIAN_POINT('',(54.818810633147,0.75,-16.2526305799144));
#44917=CARTESIAN_POINT('Origin',(62.6014464469636,0.75,-13.3063482123366));
#44918=CARTESIAN_POINT('',(56.6900158505068,0.75,-7.44930217331016));
#44919=CARTESIAN_POINT('',(56.6900158505068,0.75,-7.44930217331016));
#44920=CARTESIAN_POINT('',(70.3840822607801,0.75,-10.3600658447588));
#44921=CARTESIAN_POINT('Origin',(56.6900158505068,4.95,-7.44930217331016));
#44922=CARTESIAN_POINT('',(56.6900158505068,4.95,-7.44930217331016));
#44923=CARTESIAN_POINT('Origin',(70.3840822607801,4.95,-10.3600658447588));
#44924=CARTESIAN_POINT('Origin',(54.818810633147,-4.95,-16.2526305799144));
#44925=CARTESIAN_POINT('',(54.818810633147,-0.75,-16.2526305799144));
#44926=CARTESIAN_POINT('',(54.818810633147,-4.95,-16.2526305799144));
#44927=CARTESIAN_POINT('',(56.6900158505068,-0.75,-7.44930217331016));
#44928=CARTESIAN_POINT('',(56.6900158505068,-0.75,-7.44930217331016));
#44929=CARTESIAN_POINT('',(56.6900158505068,-4.95,-7.44930217331016));
#44930=CARTESIAN_POINT('Origin',(68.5128770434203,-4.95,-19.163394251363));
#44931=CARTESIAN_POINT('',(54.818810633147,-0.75,-16.2526305799144));
#44932=CARTESIAN_POINT('Origin',(56.6900158505068,-4.95,-7.44930217331016));
#44933=CARTESIAN_POINT('',(70.3840822607801,-0.75,-10.3600658447588));
#44934=CARTESIAN_POINT('Origin',(62.6014464469636,-0.75,-13.3063482123366));
#44935=CARTESIAN_POINT('Origin',(57.,4.95,-4.5));
#44936=CARTESIAN_POINT('',(57.,0.75,-4.5));
#44937=CARTESIAN_POINT('',(57.,4.95,-4.5));
#44938=CARTESIAN_POINT('',(57.,0.75,-4.5));
#44939=CARTESIAN_POINT('Origin',(64.,0.75,0.));
#44940=CARTESIAN_POINT('',(57.,0.75,4.5));
#44941=CARTESIAN_POINT('',(57.,0.75,4.5));
#44942=CARTESIAN_POINT('',(71.,0.75,4.5));
#44943=CARTESIAN_POINT('Origin',(57.,4.95,4.5));
#44944=CARTESIAN_POINT('',(57.,4.95,4.5));
#44945=CARTESIAN_POINT('Origin',(71.,4.95,4.5));
#44946=CARTESIAN_POINT('Origin',(64.,-0.75,0.));
#44947=CARTESIAN_POINT('',(57.,-0.75,4.5));
#44948=CARTESIAN_POINT('',(71.,-0.75,4.5));
#44949=CARTESIAN_POINT('',(57.,-0.75,-4.5));
#44950=CARTESIAN_POINT('',(57.,-0.75,4.5));
#44951=CARTESIAN_POINT('',(57.,-0.75,-4.5));
#44952=CARTESIAN_POINT('Origin',(71.,-4.95,-4.5));
#44953=CARTESIAN_POINT('',(57.,-4.95,-4.5));
#44954=CARTESIAN_POINT('Origin',(57.,-4.95,-4.5));
#44955=CARTESIAN_POINT('',(57.,-4.95,4.5));
#44956=CARTESIAN_POINT('Origin',(57.,-4.95,4.5));
#44957=CARTESIAN_POINT('Origin',(0.,0.,0.));
#55698=UNCERTAINTY_MEASURE_WITH_UNIT(LENGTH_MEASURE(0.01),#55738,
'DISTANCE_ACCURACY_VALUE',
'Maximum model space distance between geometric entities at asserted c
onnectivities');
#55715=UNCERTAINTY_MEASURE_WITH_UNIT(LENGTH_MEASURE(0.01),#55738,
'DISTANCE_ACCURACY_VALUE',
'Maximum model space distance between geometric entities at asserted c
onnectivities');
#55720=(
GEOMETRIC_REPRESENTATION_CONTEXT(3)
GLOBAL_UNCERTAINTY_ASSIGNED_CONTEXT((#55698))
GLOBAL_UNIT_ASSIGNED_CONTEXT((#55738,#55740,#55741))
REPRESENTATION_CONTEXT('','3D')
);
#55737=(
GEOMETRIC_REPRESENTATION_CONTEXT(3)
GLOBAL_UNCERTAINTY_ASSIGNED_CONTEXT((#55715))
GLOBAL_UNIT_ASSIGNED_CONTEXT((#55738,#55740,#55741))
REPRESENTATION_CONTEXT('','3D')
);
#55738=(
LENGTH_UNIT()
NAMED_UNIT(*)
SI_UNIT(.MILLI.,.METRE.)
);
#55740=(
NAMED_UNIT(*)
PLANE_ANGLE_UNIT()
SI_UNIT($,.RADIAN.)
);
#55741=(
NAMED_UNIT(*)
SI_UNIT($,.STERADIAN.)
SOLID_ANGLE_UNIT()
);
#55746=SHAPE_DEFINITION_REPRESENTATION(#55767,#55824);
#55767=PRODUCT_DEFINITION_SHAPE('',$,#55846);
#55824=SHAPE_REPRESENTATION('',(#28371),#55720);
#55841=PRODUCT_DEFINITION_CONTEXT('part definition',#55906,'design');
#55846=PRODUCT_DEFINITION('2026-10-26-00-34-17-360',
'04_Turbine_Impeller_Brass',#55867,#55841);
#55867=PRODUCT_DEFINITION_FORMATION('',$,#55912);
#55906=APPLICATION_CONTEXT(
'Core Data for Automotive Mechanical Design Process');
#55907=PRODUCT_CONTEXT('part definition',#55906,'mechanical');
#55912=PRODUCT('2026-10-26-00-34-17-360','04_Turbine_Impeller_Brass',$,
(#55907));
#55978=COLOUR_RGB('Sky Blue',0.24,0.69,0.87);
#55979=FILL_AREA_STYLE_COLOUR('',#55978);
#55980=FILL_AREA_STYLE('',(#55979));
#55981=SURFACE_STYLE_FILL_AREA(#55980);
#55982=SURFACE_SIDE_STYLE('',(#55981));
#55983=SURFACE_STYLE_USAGE(.BOTH.,#55982);
#55984=PRESENTATION_STYLE_ASSIGNMENT((#55983));
ENDSEC;
END-ISO-10303-21;
